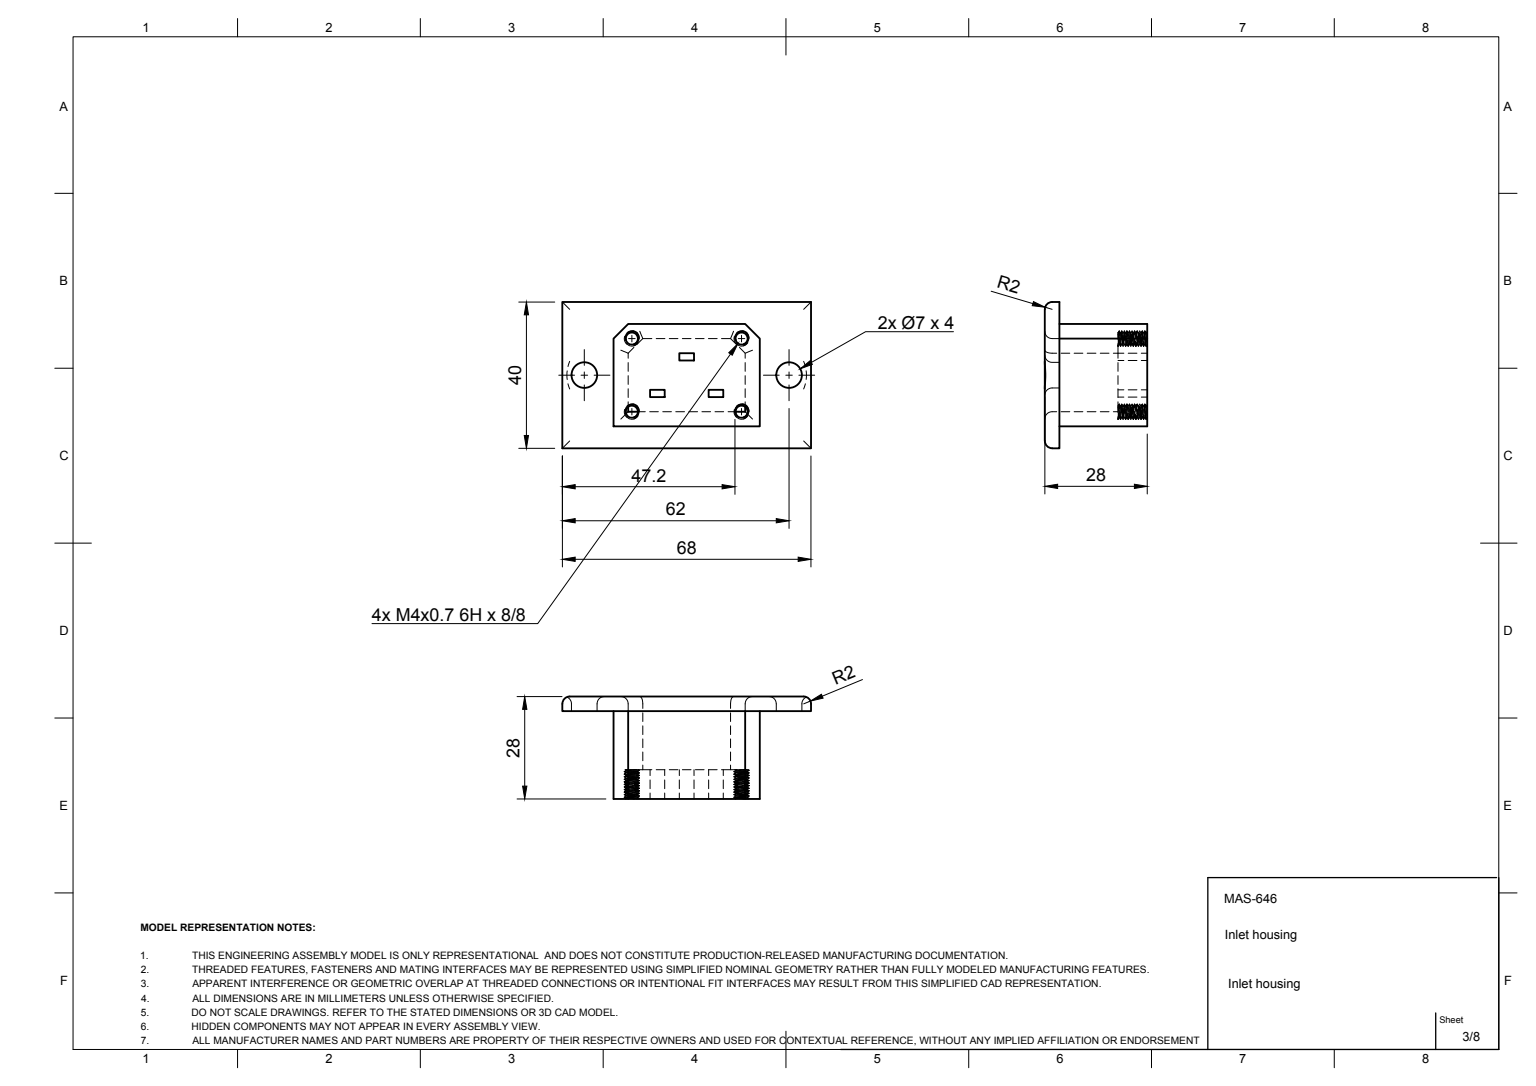
ISO-10303-21;
HEADER;
/* Generated by software containing ST-Developer
 * from STEP Tools, Inc. (www.steptools.com) 
 */

FILE_DESCRIPTION(
/* description */ ('Independent keyed three-contact power inlet for the IEC-connector des
ign category. Longer ground blade, retained contacts, wire termination
 holes and sealed bolted panel interface. Nominal custom interface; IE
C dimensional compatibility and electrical ratings are not assigned.'),

/* implementation_level */ '2;1');

FILE_NAME(
/* name */ 'Inlet housing.step',
/* time_stamp */ '2026-11-08T19:55:04-08:00',
/* author */ (''),
/* organization */ (''),
/* preprocessor_version */ 'ST-DEVELOPER v20.2',
/* originating_system */ 'Autodesk Translation Framework v15.17.0.0',
/* authorisation */ '');

FILE_SCHEMA (('AUTOMOTIVE_DESIGN { 1 0 10303 214 3 1 1 }'));
ENDSEC;

DATA;
#10=MECHANICAL_DESIGN_GEOMETRIC_PRESENTATION_REPRESENTATION('',(#109),#21880);
#89=SHAPE_REPRESENTATION_RELATIONSHIP('SRR','None',#21925,#99);
#99=ADVANCED_BREP_SHAPE_REPRESENTATION('',(#119),#21870);
#109=STYLED_ITEM('',(#21984),#119);
#119=MANIFOLD_SOLID_BREP('Body1',#6381);
#129=B_SPLINE_SURFACE_WITH_KNOTS('',3,3,((#11744,#11745,#11746,#11747,#11748,
#11749,#11750,#11751,#11752,#11753,#11754,#11755,#11756,#11757,#11758,#11759,
#11760,#11761,#11762,#11763,#11764,#11765,#11766,#11767,#11768,#11769,#11770,
#11771,#11772,#11773,#11774,#11775,#11776,#11777,#11778,#11779,#11780,#11781,
#11782,#11783,#11784,#11785,#11786,#11787,#11788,#11789,#11790,#11791,#11792,
#11793,#11794,#11795,#11796,#11797,#11798,#11799,#11800,#11801,#11802,#11803,
#11804,#11805,#11806,#11807,#11808,#11809,#11810,#11811,#11812,#11813,#11814,
#11815,#11816,#11817,#11818,#11819,#11820),(#11821,#11822,#11823,#11824,
#11825,#11826,#11827,#11828,#11829,#11830,#11831,#11832,#11833,#11834,#11835,
#11836,#11837,#11838,#11839,#11840,#11841,#11842,#11843,#11844,#11845,#11846,
#11847,#11848,#11849,#11850,#11851,#11852,#11853,#11854,#11855,#11856,#11857,
#11858,#11859,#11860,#11861,#11862,#11863,#11864,#11865,#11866,#11867,#11868,
#11869,#11870,#11871,#11872,#11873,#11874,#11875,#11876,#11877,#11878,#11879,
#11880,#11881,#11882,#11883,#11884,#11885,#11886,#11887,#11888,#11889,#11890,
#11891,#11892,#11893,#11894,#11895,#11896,#11897),(#11898,#11899,#11900,
#11901,#11902,#11903,#11904,#11905,#11906,#11907,#11908,#11909,#11910,#11911,
#11912,#11913,#11914,#11915,#11916,#11917,#11918,#11919,#11920,#11921,#11922,
#11923,#11924,#11925,#11926,#11927,#11928,#11929,#11930,#11931,#11932,#11933,
#11934,#11935,#11936,#11937,#11938,#11939,#11940,#11941,#11942,#11943,#11944,
#11945,#11946,#11947,#11948,#11949,#11950,#11951,#11952,#11953,#11954,#11955,
#11956,#11957,#11958,#11959,#11960,#11961,#11962,#11963,#11964,#11965,#11966,
#11967,#11968,#11969,#11970,#11971,#11972,#11973,#11974),(#11975,#11976,
#11977,#11978,#11979,#11980,#11981,#11982,#11983,#11984,#11985,#11986,#11987,
#11988,#11989,#11990,#11991,#11992,#11993,#11994,#11995,#11996,#11997,#11998,
#11999,#12000,#12001,#12002,#12003,#12004,#12005,#12006,#12007,#12008,#12009,
#12010,#12011,#12012,#12013,#12014,#12015,#12016,#12017,#12018,#12019,#12020,
#12021,#12022,#12023,#12024,#12025,#12026,#12027,#12028,#12029,#12030,#12031,
#12032,#12033,#12034,#12035,#12036,#12037,#12038,#12039,#12040,#12041,#12042,
#12043,#12044,#12045,#12046,#12047,#12048,#12049,#12050,#12051)),
 .UNSPECIFIED.,.F.,.F.,.F.,(4,4),(4,1,1,1,1,1,1,1,1,1,1,1,1,1,1,1,1,1,1,
1,1,1,1,1,1,1,1,1,1,1,1,1,1,1,1,1,1,1,1,1,1,1,1,1,1,1,1,1,1,1,1,1,1,1,1,
1,1,1,1,1,1,1,1,1,1,1,1,1,1,1,1,1,1,1,4),(0.,0.0448889834294934),(11.8615800042567,
12.859180611653,13.8567812190493,14.8543818264456,15.8519824338419,16.8495830412382,
17.8471836486345,18.8447842560309,19.8423848634272,20.8399854708235,21.8375860782198,
22.8351866856161,23.8327872930124,24.8303879004087,25.827988507805,26.8255891152013,
27.8231897225976,28.8207903299939,29.8183909373903,30.8159915447866,31.8135921521829,
32.8111927595792,33.8087933669755,34.8063939743718,35.8039945817681,36.8015951891644,
37.7991957965607,38.796796403957,39.7943970113533,40.7919976187497,41.789598226146,
42.7871988335423,43.7847994409386,44.7824000483349,45.7800006557312,46.7776012631275,
47.7752018705238,48.7728024779201,49.7704030853164,50.7680036927128,51.7656043001091,
52.7632049075054,53.7608055149017,54.758406122298,55.7560067296943,56.7536073370906,
57.7512079444869,58.7488085518832,59.7464091592795,60.7440097666758,61.7416103740722,
62.7392109814685,63.7368115888648,64.7344121962611,65.7320128036574,66.7296134110537,
67.72721401845,68.7248146258463,69.7224152332426,70.7200158406389,71.7176164480352,
72.7152170554316,73.7128176628279,74.7104182702242,75.7080188776205,76.7056194850168,
77.7032200924131,78.7008206998094,79.6984213072057,80.696021914602,81.6936225219983,
82.6912231293946,83.688823736791,84.6864243441873,85.6840249515836),
 .UNSPECIFIED.);
#130=B_SPLINE_SURFACE_WITH_KNOTS('',3,3,((#12248,#12249,#12250,#12251,#12252,
#12253,#12254,#12255,#12256,#12257,#12258,#12259,#12260,#12261,#12262,#12263,
#12264,#12265,#12266,#12267,#12268,#12269,#12270,#12271,#12272,#12273,#12274,
#12275,#12276,#12277,#12278,#12279,#12280,#12281,#12282,#12283,#12284,#12285,
#12286,#12287,#12288,#12289,#12290,#12291,#12292,#12293,#12294,#12295,#12296,
#12297,#12298,#12299,#12300,#12301,#12302,#12303,#12304,#12305,#12306,#12307,
#12308,#12309,#12310,#12311,#12312,#12313,#12314,#12315,#12316,#12317,#12318,
#12319,#12320,#12321,#12322,#12323,#12324),(#12325,#12326,#12327,#12328,
#12329,#12330,#12331,#12332,#12333,#12334,#12335,#12336,#12337,#12338,#12339,
#12340,#12341,#12342,#12343,#12344,#12345,#12346,#12347,#12348,#12349,#12350,
#12351,#12352,#12353,#12354,#12355,#12356,#12357,#12358,#12359,#12360,#12361,
#12362,#12363,#12364,#12365,#12366,#12367,#12368,#12369,#12370,#12371,#12372,
#12373,#12374,#12375,#12376,#12377,#12378,#12379,#12380,#12381,#12382,#12383,
#12384,#12385,#12386,#12387,#12388,#12389,#12390,#12391,#12392,#12393,#12394,
#12395,#12396,#12397,#12398,#12399,#12400,#12401),(#12402,#12403,#12404,
#12405,#12406,#12407,#12408,#12409,#12410,#12411,#12412,#12413,#12414,#12415,
#12416,#12417,#12418,#12419,#12420,#12421,#12422,#12423,#12424,#12425,#12426,
#12427,#12428,#12429,#12430,#12431,#12432,#12433,#12434,#12435,#12436,#12437,
#12438,#12439,#12440,#12441,#12442,#12443,#12444,#12445,#12446,#12447,#12448,
#12449,#12450,#12451,#12452,#12453,#12454,#12455,#12456,#12457,#12458,#12459,
#12460,#12461,#12462,#12463,#12464,#12465,#12466,#12467,#12468,#12469,#12470,
#12471,#12472,#12473,#12474,#12475,#12476,#12477,#12478),(#12479,#12480,
#12481,#12482,#12483,#12484,#12485,#12486,#12487,#12488,#12489,#12490,#12491,
#12492,#12493,#12494,#12495,#12496,#12497,#12498,#12499,#12500,#12501,#12502,
#12503,#12504,#12505,#12506,#12507,#12508,#12509,#12510,#12511,#12512,#12513,
#12514,#12515,#12516,#12517,#12518,#12519,#12520,#12521,#12522,#12523,#12524,
#12525,#12526,#12527,#12528,#12529,#12530,#12531,#12532,#12533,#12534,#12535,
#12536,#12537,#12538,#12539,#12540,#12541,#12542,#12543,#12544,#12545,#12546,
#12547,#12548,#12549,#12550,#12551,#12552,#12553,#12554,#12555)),
 .UNSPECIFIED.,.F.,.F.,.F.,(4,4),(4,1,1,1,1,1,1,1,1,1,1,1,1,1,1,1,1,1,1,
1,1,1,1,1,1,1,1,1,1,1,1,1,1,1,1,1,1,1,1,1,1,1,1,1,1,1,1,1,1,1,1,1,1,1,1,
1,1,1,1,1,1,1,1,1,1,1,1,1,1,1,1,1,1,1,4),(0.,0.0448889834294934),(14.3981410127769,
15.3957416201732,16.3933422275696,17.3909428349659,18.3885434423622,19.3861440497585,
20.3837446571548,21.3813452645511,22.3789458719474,23.3765464793437,24.37414708674,
25.3717476941363,26.3693483015326,27.366948908929,28.3645495163253,29.3621501237216,
30.3597507311179,31.3573513385142,32.3549519459105,33.3525525533068,34.3501531607031,
35.3477537680994,36.3453543754957,37.342954982892,38.3405555902884,39.3381561976847,
40.335756805081,41.3333574124773,42.3309580198736,43.3285586272699,44.3261592346662,
45.3237598420625,46.3213604494588,47.3189610568551,48.3165616642514,49.3141622716478,
50.3117628790441,51.3093634864404,52.3069640938367,53.304564701233,54.3021653086293,
55.2997659160256,56.2973665234219,57.2949671308182,58.2925677382145,59.2901683456108,
60.2877689530072,61.2853695604035,62.2829701677998,63.2805707751961,64.2781713825924,
65.2757719899887,66.273372597385,67.2709732047813,68.2685738121776,69.2661744195739,
70.2637750269702,71.2613756343666,72.2589762417629,73.2565768491592,74.2541774565555,
75.2517780639518,76.2493786713481,77.2469792787444,78.2445798861407,79.242180493537,
80.2397811009333,81.2373817083296,82.2349823157259,83.2325829231223,84.2301835305186,
85.2277841379149,86.2253847453112,87.2229853527075,88.2205859601038),
 .UNSPECIFIED.);
#131=B_SPLINE_SURFACE_WITH_KNOTS('',3,3,((#13305,#13306,#13307,#13308,#13309,
#13310,#13311,#13312,#13313,#13314,#13315,#13316,#13317,#13318,#13319,#13320,
#13321,#13322,#13323,#13324,#13325,#13326,#13327,#13328,#13329,#13330,#13331,
#13332,#13333,#13334,#13335,#13336,#13337,#13338,#13339,#13340,#13341,#13342,
#13343,#13344,#13345,#13346,#13347,#13348,#13349,#13350,#13351,#13352,#13353,
#13354,#13355,#13356,#13357,#13358,#13359,#13360,#13361,#13362,#13363,#13364,
#13365,#13366,#13367,#13368,#13369,#13370,#13371,#13372,#13373,#13374,#13375,
#13376,#13377,#13378,#13379,#13380,#13381),(#13382,#13383,#13384,#13385,
#13386,#13387,#13388,#13389,#13390,#13391,#13392,#13393,#13394,#13395,#13396,
#13397,#13398,#13399,#13400,#13401,#13402,#13403,#13404,#13405,#13406,#13407,
#13408,#13409,#13410,#13411,#13412,#13413,#13414,#13415,#13416,#13417,#13418,
#13419,#13420,#13421,#13422,#13423,#13424,#13425,#13426,#13427,#13428,#13429,
#13430,#13431,#13432,#13433,#13434,#13435,#13436,#13437,#13438,#13439,#13440,
#13441,#13442,#13443,#13444,#13445,#13446,#13447,#13448,#13449,#13450,#13451,
#13452,#13453,#13454,#13455,#13456,#13457,#13458),(#13459,#13460,#13461,
#13462,#13463,#13464,#13465,#13466,#13467,#13468,#13469,#13470,#13471,#13472,
#13473,#13474,#13475,#13476,#13477,#13478,#13479,#13480,#13481,#13482,#13483,
#13484,#13485,#13486,#13487,#13488,#13489,#13490,#13491,#13492,#13493,#13494,
#13495,#13496,#13497,#13498,#13499,#13500,#13501,#13502,#13503,#13504,#13505,
#13506,#13507,#13508,#13509,#13510,#13511,#13512,#13513,#13514,#13515,#13516,
#13517,#13518,#13519,#13520,#13521,#13522,#13523,#13524,#13525,#13526,#13527,
#13528,#13529,#13530,#13531,#13532,#13533,#13534,#13535),(#13536,#13537,
#13538,#13539,#13540,#13541,#13542,#13543,#13544,#13545,#13546,#13547,#13548,
#13549,#13550,#13551,#13552,#13553,#13554,#13555,#13556,#13557,#13558,#13559,
#13560,#13561,#13562,#13563,#13564,#13565,#13566,#13567,#13568,#13569,#13570,
#13571,#13572,#13573,#13574,#13575,#13576,#13577,#13578,#13579,#13580,#13581,
#13582,#13583,#13584,#13585,#13586,#13587,#13588,#13589,#13590,#13591,#13592,
#13593,#13594,#13595,#13596,#13597,#13598,#13599,#13600,#13601,#13602,#13603,
#13604,#13605,#13606,#13607,#13608,#13609,#13610,#13611,#13612)),
 .UNSPECIFIED.,.F.,.F.,.F.,(4,4),(4,1,1,1,1,1,1,1,1,1,1,1,1,1,1,1,1,1,1,
1,1,1,1,1,1,1,1,1,1,1,1,1,1,1,1,1,1,1,1,1,1,1,1,1,1,1,1,1,1,1,1,1,1,1,1,
1,1,1,1,1,1,1,1,1,1,1,1,1,1,1,1,1,1,1,4),(0.,0.0448889834294934),(11.8615800042567,
12.859180611653,13.8567812190493,14.8543818264456,15.8519824338419,16.8495830412382,
17.8471836486345,18.8447842560308,19.8423848634271,20.8399854708235,21.8375860782198,
22.8351866856161,23.8327872930124,24.8303879004087,25.827988507805,26.8255891152013,
27.8231897225976,28.8207903299939,29.8183909373902,30.8159915447865,31.8135921521829,
32.8111927595792,33.8087933669755,34.8063939743718,35.8039945817681,36.8015951891644,
37.7991957965607,38.796796403957,39.7943970113533,40.7919976187496,41.7895982261459,
42.7871988335423,43.7847994409386,44.7824000483349,45.7800006557312,46.7776012631275,
47.7752018705238,48.7728024779201,49.7704030853164,50.7680036927127,51.765604300109,
52.7632049075054,53.7608055149017,54.758406122298,55.7560067296943,56.7536073370906,
57.7512079444869,58.7488085518832,59.7464091592795,60.7440097666758,61.7416103740721,
62.7392109814684,63.7368115888648,64.7344121962611,65.7320128036574,66.7296134110537,
67.72721401845,68.7248146258463,69.7224152332426,70.7200158406389,71.7176164480352,
72.7152170554315,73.7128176628278,74.7104182702242,75.7080188776205,76.7056194850168,
77.7032200924131,78.7008206998094,79.6984213072057,80.696021914602,81.6936225219983,
82.6912231293946,83.6888237367909,84.6864243441872,85.6840249515836),
 .UNSPECIFIED.);
#132=B_SPLINE_SURFACE_WITH_KNOTS('',3,3,((#13726,#13727,#13728,#13729,#13730,
#13731,#13732,#13733,#13734,#13735,#13736,#13737,#13738,#13739,#13740,#13741,
#13742,#13743,#13744,#13745,#13746,#13747,#13748,#13749,#13750,#13751,#13752,
#13753,#13754,#13755,#13756,#13757,#13758,#13759,#13760,#13761,#13762,#13763,
#13764,#13765,#13766,#13767,#13768,#13769,#13770,#13771,#13772,#13773,#13774,
#13775,#13776,#13777,#13778,#13779,#13780,#13781,#13782,#13783,#13784,#13785,
#13786,#13787,#13788,#13789,#13790,#13791,#13792,#13793,#13794,#13795,#13796,
#13797,#13798,#13799,#13800,#13801,#13802),(#13803,#13804,#13805,#13806,
#13807,#13808,#13809,#13810,#13811,#13812,#13813,#13814,#13815,#13816,#13817,
#13818,#13819,#13820,#13821,#13822,#13823,#13824,#13825,#13826,#13827,#13828,
#13829,#13830,#13831,#13832,#13833,#13834,#13835,#13836,#13837,#13838,#13839,
#13840,#13841,#13842,#13843,#13844,#13845,#13846,#13847,#13848,#13849,#13850,
#13851,#13852,#13853,#13854,#13855,#13856,#13857,#13858,#13859,#13860,#13861,
#13862,#13863,#13864,#13865,#13866,#13867,#13868,#13869,#13870,#13871,#13872,
#13873,#13874,#13875,#13876,#13877,#13878,#13879),(#13880,#13881,#13882,
#13883,#13884,#13885,#13886,#13887,#13888,#13889,#13890,#13891,#13892,#13893,
#13894,#13895,#13896,#13897,#13898,#13899,#13900,#13901,#13902,#13903,#13904,
#13905,#13906,#13907,#13908,#13909,#13910,#13911,#13912,#13913,#13914,#13915,
#13916,#13917,#13918,#13919,#13920,#13921,#13922,#13923,#13924,#13925,#13926,
#13927,#13928,#13929,#13930,#13931,#13932,#13933,#13934,#13935,#13936,#13937,
#13938,#13939,#13940,#13941,#13942,#13943,#13944,#13945,#13946,#13947,#13948,
#13949,#13950,#13951,#13952,#13953,#13954,#13955,#13956),(#13957,#13958,
#13959,#13960,#13961,#13962,#13963,#13964,#13965,#13966,#13967,#13968,#13969,
#13970,#13971,#13972,#13973,#13974,#13975,#13976,#13977,#13978,#13979,#13980,
#13981,#13982,#13983,#13984,#13985,#13986,#13987,#13988,#13989,#13990,#13991,
#13992,#13993,#13994,#13995,#13996,#13997,#13998,#13999,#14000,#14001,#14002,
#14003,#14004,#14005,#14006,#14007,#14008,#14009,#14010,#14011,#14012,#14013,
#14014,#14015,#14016,#14017,#14018,#14019,#14020,#14021,#14022,#14023,#14024,
#14025,#14026,#14027,#14028,#14029,#14030,#14031,#14032,#14033)),
 .UNSPECIFIED.,.F.,.F.,.F.,(4,4),(4,1,1,1,1,1,1,1,1,1,1,1,1,1,1,1,1,1,1,
1,1,1,1,1,1,1,1,1,1,1,1,1,1,1,1,1,1,1,1,1,1,1,1,1,1,1,1,1,1,1,1,1,1,1,1,
1,1,1,1,1,1,1,1,1,1,1,1,1,1,1,1,1,1,1,4),(0.,0.0448889834294934),(14.3981410127769,
15.3957416201732,16.3933422275695,17.3909428349659,18.3885434423622,19.3861440497585,
20.3837446571548,21.3813452645511,22.3789458719474,23.3765464793437,24.37414708674,
25.3717476941363,26.3693483015326,27.3669489089289,28.3645495163252,29.3621501237216,
30.3597507311179,31.3573513385142,32.3549519459105,33.3525525533068,34.3501531607031,
35.3477537680994,36.3453543754957,37.342954982892,38.3405555902883,39.3381561976846,
40.335756805081,41.3333574124773,42.3309580198736,43.3285586272699,44.3261592346662,
45.3237598420625,46.3213604494588,47.3189610568551,48.3165616642514,49.3141622716477,
50.3117628790441,51.3093634864404,52.3069640938367,53.304564701233,54.3021653086293,
55.2997659160256,56.2973665234219,57.2949671308182,58.2925677382145,59.2901683456108,
60.2877689530071,61.2853695604035,62.2829701677998,63.2805707751961,64.2781713825924,
65.2757719899887,66.273372597385,67.2709732047813,68.2685738121776,69.2661744195739,
70.2637750269702,71.2613756343665,72.2589762417629,73.2565768491592,74.2541774565555,
75.2517780639518,76.2493786713481,77.2469792787444,78.2445798861407,79.242180493537,
80.2397811009333,81.2373817083296,82.2349823157259,83.2325829231222,84.2301835305186,
85.2277841379149,86.2253847453112,87.2229853527075,88.2205859601038),
 .UNSPECIFIED.);
#133=B_SPLINE_SURFACE_WITH_KNOTS('',3,3,((#14163,#14164,#14165,#14166,#14167,
#14168,#14169,#14170,#14171,#14172,#14173,#14174,#14175,#14176,#14177,#14178,
#14179,#14180,#14181,#14182,#14183,#14184,#14185,#14186,#14187,#14188,#14189,
#14190,#14191,#14192,#14193,#14194,#14195,#14196,#14197,#14198,#14199,#14200,
#14201,#14202,#14203,#14204,#14205,#14206,#14207,#14208,#14209,#14210,#14211,
#14212,#14213,#14214,#14215,#14216,#14217,#14218,#14219,#14220,#14221,#14222,
#14223,#14224,#14225,#14226,#14227,#14228,#14229,#14230,#14231,#14232,#14233,
#14234,#14235,#14236,#14237,#14238,#14239),(#14240,#14241,#14242,#14243,
#14244,#14245,#14246,#14247,#14248,#14249,#14250,#14251,#14252,#14253,#14254,
#14255,#14256,#14257,#14258,#14259,#14260,#14261,#14262,#14263,#14264,#14265,
#14266,#14267,#14268,#14269,#14270,#14271,#14272,#14273,#14274,#14275,#14276,
#14277,#14278,#14279,#14280,#14281,#14282,#14283,#14284,#14285,#14286,#14287,
#14288,#14289,#14290,#14291,#14292,#14293,#14294,#14295,#14296,#14297,#14298,
#14299,#14300,#14301,#14302,#14303,#14304,#14305,#14306,#14307,#14308,#14309,
#14310,#14311,#14312,#14313,#14314,#14315,#14316),(#14317,#14318,#14319,
#14320,#14321,#14322,#14323,#14324,#14325,#14326,#14327,#14328,#14329,#14330,
#14331,#14332,#14333,#14334,#14335,#14336,#14337,#14338,#14339,#14340,#14341,
#14342,#14343,#14344,#14345,#14346,#14347,#14348,#14349,#14350,#14351,#14352,
#14353,#14354,#14355,#14356,#14357,#14358,#14359,#14360,#14361,#14362,#14363,
#14364,#14365,#14366,#14367,#14368,#14369,#14370,#14371,#14372,#14373,#14374,
#14375,#14376,#14377,#14378,#14379,#14380,#14381,#14382,#14383,#14384,#14385,
#14386,#14387,#14388,#14389,#14390,#14391,#14392,#14393),(#14394,#14395,
#14396,#14397,#14398,#14399,#14400,#14401,#14402,#14403,#14404,#14405,#14406,
#14407,#14408,#14409,#14410,#14411,#14412,#14413,#14414,#14415,#14416,#14417,
#14418,#14419,#14420,#14421,#14422,#14423,#14424,#14425,#14426,#14427,#14428,
#14429,#14430,#14431,#14432,#14433,#14434,#14435,#14436,#14437,#14438,#14439,
#14440,#14441,#14442,#14443,#14444,#14445,#14446,#14447,#14448,#14449,#14450,
#14451,#14452,#14453,#14454,#14455,#14456,#14457,#14458,#14459,#14460,#14461,
#14462,#14463,#14464,#14465,#14466,#14467,#14468,#14469,#14470)),
 .UNSPECIFIED.,.F.,.F.,.F.,(4,4),(4,1,1,1,1,1,1,1,1,1,1,1,1,1,1,1,1,1,1,
1,1,1,1,1,1,1,1,1,1,1,1,1,1,1,1,1,1,1,1,1,1,1,1,1,1,1,1,1,1,1,1,1,1,1,1,
1,1,1,1,1,1,1,1,1,1,1,1,1,1,1,1,1,1,1,4),(0.,0.0448889834294934),(11.8615800042567,
12.859180611653,13.8567812190493,14.8543818264456,15.8519824338419,16.8495830412382,
17.8471836486345,18.8447842560308,19.8423848634271,20.8399854708235,21.8375860782198,
22.8351866856161,23.8327872930124,24.8303879004087,25.827988507805,26.8255891152013,
27.8231897225976,28.8207903299939,29.8183909373902,30.8159915447865,31.8135921521829,
32.8111927595792,33.8087933669755,34.8063939743718,35.8039945817681,36.8015951891644,
37.7991957965607,38.796796403957,39.7943970113533,40.7919976187496,41.7895982261459,
42.7871988335423,43.7847994409386,44.7824000483349,45.7800006557312,46.7776012631275,
47.7752018705238,48.7728024779201,49.7704030853164,50.7680036927127,51.765604300109,
52.7632049075054,53.7608055149017,54.758406122298,55.7560067296943,56.7536073370906,
57.7512079444869,58.7488085518832,59.7464091592795,60.7440097666758,61.7416103740721,
62.7392109814684,63.7368115888648,64.7344121962611,65.7320128036574,66.7296134110537,
67.72721401845,68.7248146258463,69.7224152332426,70.7200158406389,71.7176164480352,
72.7152170554315,73.7128176628278,74.7104182702242,75.7080188776205,76.7056194850168,
77.7032200924131,78.7008206998094,79.6984213072057,80.696021914602,81.6936225219983,
82.6912231293946,83.6888237367909,84.6864243441872,85.6840249515836),
 .UNSPECIFIED.);
#134=B_SPLINE_SURFACE_WITH_KNOTS('',3,3,((#14584,#14585,#14586,#14587,#14588,
#14589,#14590,#14591,#14592,#14593,#14594,#14595,#14596,#14597,#14598,#14599,
#14600,#14601,#14602,#14603,#14604,#14605,#14606,#14607,#14608,#14609,#14610,
#14611,#14612,#14613,#14614,#14615,#14616,#14617,#14618,#14619,#14620,#14621,
#14622,#14623,#14624,#14625,#14626,#14627,#14628,#14629,#14630,#14631,#14632,
#14633,#14634,#14635,#14636,#14637,#14638,#14639,#14640,#14641,#14642,#14643,
#14644,#14645,#14646,#14647,#14648,#14649,#14650,#14651,#14652,#14653,#14654,
#14655,#14656,#14657,#14658,#14659,#14660),(#14661,#14662,#14663,#14664,
#14665,#14666,#14667,#14668,#14669,#14670,#14671,#14672,#14673,#14674,#14675,
#14676,#14677,#14678,#14679,#14680,#14681,#14682,#14683,#14684,#14685,#14686,
#14687,#14688,#14689,#14690,#14691,#14692,#14693,#14694,#14695,#14696,#14697,
#14698,#14699,#14700,#14701,#14702,#14703,#14704,#14705,#14706,#14707,#14708,
#14709,#14710,#14711,#14712,#14713,#14714,#14715,#14716,#14717,#14718,#14719,
#14720,#14721,#14722,#14723,#14724,#14725,#14726,#14727,#14728,#14729,#14730,
#14731,#14732,#14733,#14734,#14735,#14736,#14737),(#14738,#14739,#14740,
#14741,#14742,#14743,#14744,#14745,#14746,#14747,#14748,#14749,#14750,#14751,
#14752,#14753,#14754,#14755,#14756,#14757,#14758,#14759,#14760,#14761,#14762,
#14763,#14764,#14765,#14766,#14767,#14768,#14769,#14770,#14771,#14772,#14773,
#14774,#14775,#14776,#14777,#14778,#14779,#14780,#14781,#14782,#14783,#14784,
#14785,#14786,#14787,#14788,#14789,#14790,#14791,#14792,#14793,#14794,#14795,
#14796,#14797,#14798,#14799,#14800,#14801,#14802,#14803,#14804,#14805,#14806,
#14807,#14808,#14809,#14810,#14811,#14812,#14813,#14814),(#14815,#14816,
#14817,#14818,#14819,#14820,#14821,#14822,#14823,#14824,#14825,#14826,#14827,
#14828,#14829,#14830,#14831,#14832,#14833,#14834,#14835,#14836,#14837,#14838,
#14839,#14840,#14841,#14842,#14843,#14844,#14845,#14846,#14847,#14848,#14849,
#14850,#14851,#14852,#14853,#14854,#14855,#14856,#14857,#14858,#14859,#14860,
#14861,#14862,#14863,#14864,#14865,#14866,#14867,#14868,#14869,#14870,#14871,
#14872,#14873,#14874,#14875,#14876,#14877,#14878,#14879,#14880,#14881,#14882,
#14883,#14884,#14885,#14886,#14887,#14888,#14889,#14890,#14891)),
 .UNSPECIFIED.,.F.,.F.,.F.,(4,4),(4,1,1,1,1,1,1,1,1,1,1,1,1,1,1,1,1,1,1,
1,1,1,1,1,1,1,1,1,1,1,1,1,1,1,1,1,1,1,1,1,1,1,1,1,1,1,1,1,1,1,1,1,1,1,1,
1,1,1,1,1,1,1,1,1,1,1,1,1,1,1,1,1,1,1,4),(0.,0.0448889834294934),(14.3981410127769,
15.3957416201732,16.3933422275695,17.3909428349659,18.3885434423622,19.3861440497585,
20.3837446571548,21.3813452645511,22.3789458719474,23.3765464793437,24.37414708674,
25.3717476941363,26.3693483015326,27.3669489089289,28.3645495163252,29.3621501237216,
30.3597507311179,31.3573513385142,32.3549519459105,33.3525525533068,34.3501531607031,
35.3477537680994,36.3453543754957,37.342954982892,38.3405555902883,39.3381561976846,
40.335756805081,41.3333574124773,42.3309580198736,43.3285586272699,44.3261592346662,
45.3237598420625,46.3213604494588,47.3189610568551,48.3165616642514,49.3141622716477,
50.3117628790441,51.3093634864404,52.3069640938367,53.304564701233,54.3021653086293,
55.2997659160256,56.2973665234219,57.2949671308182,58.2925677382145,59.2901683456108,
60.2877689530071,61.2853695604035,62.2829701677998,63.2805707751961,64.2781713825924,
65.2757719899887,66.273372597385,67.2709732047813,68.2685738121776,69.2661744195739,
70.2637750269702,71.2613756343665,72.2589762417629,73.2565768491592,74.2541774565555,
75.2517780639518,76.2493786713481,77.2469792787444,78.2445798861407,79.242180493537,
80.2397811009333,81.2373817083296,82.2349823157259,83.2325829231222,84.2301835305186,
85.2277841379149,86.2253847453112,87.2229853527075,88.2205859601038),
 .UNSPECIFIED.);
#135=B_SPLINE_SURFACE_WITH_KNOTS('',3,3,((#15021,#15022,#15023,#15024,#15025,
#15026,#15027,#15028,#15029,#15030,#15031,#15032,#15033,#15034,#15035,#15036,
#15037,#15038,#15039,#15040,#15041,#15042,#15043,#15044,#15045,#15046,#15047,
#15048,#15049,#15050,#15051,#15052,#15053,#15054,#15055,#15056,#15057,#15058,
#15059,#15060,#15061,#15062,#15063,#15064,#15065,#15066,#15067,#15068,#15069,
#15070,#15071,#15072,#15073,#15074,#15075,#15076,#15077,#15078,#15079,#15080,
#15081,#15082,#15083,#15084,#15085,#15086,#15087,#15088,#15089,#15090,#15091,
#15092,#15093,#15094,#15095,#15096,#15097),(#15098,#15099,#15100,#15101,
#15102,#15103,#15104,#15105,#15106,#15107,#15108,#15109,#15110,#15111,#15112,
#15113,#15114,#15115,#15116,#15117,#15118,#15119,#15120,#15121,#15122,#15123,
#15124,#15125,#15126,#15127,#15128,#15129,#15130,#15131,#15132,#15133,#15134,
#15135,#15136,#15137,#15138,#15139,#15140,#15141,#15142,#15143,#15144,#15145,
#15146,#15147,#15148,#15149,#15150,#15151,#15152,#15153,#15154,#15155,#15156,
#15157,#15158,#15159,#15160,#15161,#15162,#15163,#15164,#15165,#15166,#15167,
#15168,#15169,#15170,#15171,#15172,#15173,#15174),(#15175,#15176,#15177,
#15178,#15179,#15180,#15181,#15182,#15183,#15184,#15185,#15186,#15187,#15188,
#15189,#15190,#15191,#15192,#15193,#15194,#15195,#15196,#15197,#15198,#15199,
#15200,#15201,#15202,#15203,#15204,#15205,#15206,#15207,#15208,#15209,#15210,
#15211,#15212,#15213,#15214,#15215,#15216,#15217,#15218,#15219,#15220,#15221,
#15222,#15223,#15224,#15225,#15226,#15227,#15228,#15229,#15230,#15231,#15232,
#15233,#15234,#15235,#15236,#15237,#15238,#15239,#15240,#15241,#15242,#15243,
#15244,#15245,#15246,#15247,#15248,#15249,#15250,#15251),(#15252,#15253,
#15254,#15255,#15256,#15257,#15258,#15259,#15260,#15261,#15262,#15263,#15264,
#15265,#15266,#15267,#15268,#15269,#15270,#15271,#15272,#15273,#15274,#15275,
#15276,#15277,#15278,#15279,#15280,#15281,#15282,#15283,#15284,#15285,#15286,
#15287,#15288,#15289,#15290,#15291,#15292,#15293,#15294,#15295,#15296,#15297,
#15298,#15299,#15300,#15301,#15302,#15303,#15304,#15305,#15306,#15307,#15308,
#15309,#15310,#15311,#15312,#15313,#15314,#15315,#15316,#15317,#15318,#15319,
#15320,#15321,#15322,#15323,#15324,#15325,#15326,#15327,#15328)),
 .UNSPECIFIED.,.F.,.F.,.F.,(4,4),(4,1,1,1,1,1,1,1,1,1,1,1,1,1,1,1,1,1,1,
1,1,1,1,1,1,1,1,1,1,1,1,1,1,1,1,1,1,1,1,1,1,1,1,1,1,1,1,1,1,1,1,1,1,1,1,
1,1,1,1,1,1,1,1,1,1,1,1,1,1,1,1,1,1,1,4),(0.,0.0448889834294934),(11.8615800042567,
12.859180611653,13.8567812190493,14.8543818264456,15.8519824338419,16.8495830412382,
17.8471836486345,18.8447842560309,19.8423848634272,20.8399854708235,21.8375860782198,
22.8351866856161,23.8327872930124,24.8303879004087,25.827988507805,26.8255891152013,
27.8231897225976,28.8207903299939,29.8183909373903,30.8159915447866,31.8135921521829,
32.8111927595792,33.8087933669755,34.8063939743718,35.8039945817681,36.8015951891644,
37.7991957965607,38.796796403957,39.7943970113533,40.7919976187497,41.789598226146,
42.7871988335423,43.7847994409386,44.7824000483349,45.7800006557312,46.7776012631275,
47.7752018705238,48.7728024779201,49.7704030853164,50.7680036927127,51.7656043001091,
52.7632049075054,53.7608055149017,54.758406122298,55.7560067296943,56.7536073370906,
57.7512079444869,58.7488085518832,59.7464091592795,60.7440097666758,61.7416103740721,
62.7392109814685,63.7368115888648,64.7344121962611,65.7320128036574,66.7296134110537,
67.72721401845,68.7248146258463,69.7224152332426,70.7200158406389,71.7176164480352,
72.7152170554315,73.7128176628279,74.7104182702242,75.7080188776205,76.7056194850168,
77.7032200924131,78.7008206998094,79.6984213072057,80.696021914602,81.6936225219983,
82.6912231293946,83.688823736791,84.6864243441873,85.6840249515836),
 .UNSPECIFIED.);
#136=B_SPLINE_SURFACE_WITH_KNOTS('',3,3,((#15442,#15443,#15444,#15445,#15446,
#15447,#15448,#15449,#15450,#15451,#15452,#15453,#15454,#15455,#15456,#15457,
#15458,#15459,#15460,#15461,#15462,#15463,#15464,#15465,#15466,#15467,#15468,
#15469,#15470,#15471,#15472,#15473,#15474,#15475,#15476,#15477,#15478,#15479,
#15480,#15481,#15482,#15483,#15484,#15485,#15486,#15487,#15488,#15489,#15490,
#15491,#15492,#15493,#15494,#15495,#15496,#15497,#15498,#15499,#15500,#15501,
#15502,#15503,#15504,#15505,#15506,#15507,#15508,#15509,#15510,#15511,#15512,
#15513,#15514,#15515,#15516,#15517,#15518),(#15519,#15520,#15521,#15522,
#15523,#15524,#15525,#15526,#15527,#15528,#15529,#15530,#15531,#15532,#15533,
#15534,#15535,#15536,#15537,#15538,#15539,#15540,#15541,#15542,#15543,#15544,
#15545,#15546,#15547,#15548,#15549,#15550,#15551,#15552,#15553,#15554,#15555,
#15556,#15557,#15558,#15559,#15560,#15561,#15562,#15563,#15564,#15565,#15566,
#15567,#15568,#15569,#15570,#15571,#15572,#15573,#15574,#15575,#15576,#15577,
#15578,#15579,#15580,#15581,#15582,#15583,#15584,#15585,#15586,#15587,#15588,
#15589,#15590,#15591,#15592,#15593,#15594,#15595),(#15596,#15597,#15598,
#15599,#15600,#15601,#15602,#15603,#15604,#15605,#15606,#15607,#15608,#15609,
#15610,#15611,#15612,#15613,#15614,#15615,#15616,#15617,#15618,#15619,#15620,
#15621,#15622,#15623,#15624,#15625,#15626,#15627,#15628,#15629,#15630,#15631,
#15632,#15633,#15634,#15635,#15636,#15637,#15638,#15639,#15640,#15641,#15642,
#15643,#15644,#15645,#15646,#15647,#15648,#15649,#15650,#15651,#15652,#15653,
#15654,#15655,#15656,#15657,#15658,#15659,#15660,#15661,#15662,#15663,#15664,
#15665,#15666,#15667,#15668,#15669,#15670,#15671,#15672),(#15673,#15674,
#15675,#15676,#15677,#15678,#15679,#15680,#15681,#15682,#15683,#15684,#15685,
#15686,#15687,#15688,#15689,#15690,#15691,#15692,#15693,#15694,#15695,#15696,
#15697,#15698,#15699,#15700,#15701,#15702,#15703,#15704,#15705,#15706,#15707,
#15708,#15709,#15710,#15711,#15712,#15713,#15714,#15715,#15716,#15717,#15718,
#15719,#15720,#15721,#15722,#15723,#15724,#15725,#15726,#15727,#15728,#15729,
#15730,#15731,#15732,#15733,#15734,#15735,#15736,#15737,#15738,#15739,#15740,
#15741,#15742,#15743,#15744,#15745,#15746,#15747,#15748,#15749)),
 .UNSPECIFIED.,.F.,.F.,.F.,(4,4),(4,1,1,1,1,1,1,1,1,1,1,1,1,1,1,1,1,1,1,
1,1,1,1,1,1,1,1,1,1,1,1,1,1,1,1,1,1,1,1,1,1,1,1,1,1,1,1,1,1,1,1,1,1,1,1,
1,1,1,1,1,1,1,1,1,1,1,1,1,1,1,1,1,1,1,4),(0.,0.0448889834294934),(14.3981410127769,
15.3957416201732,16.3933422275696,17.3909428349659,18.3885434423622,19.3861440497585,
20.3837446571548,21.3813452645511,22.3789458719474,23.3765464793437,24.37414708674,
25.3717476941363,26.3693483015326,27.366948908929,28.3645495163253,29.3621501237216,
30.3597507311179,31.3573513385142,32.3549519459105,33.3525525533068,34.3501531607031,
35.3477537680994,36.3453543754957,37.342954982892,38.3405555902884,39.3381561976847,
40.335756805081,41.3333574124773,42.3309580198736,43.3285586272699,44.3261592346662,
45.3237598420625,46.3213604494588,47.3189610568551,48.3165616642514,49.3141622716478,
50.3117628790441,51.3093634864404,52.3069640938367,53.304564701233,54.3021653086293,
55.2997659160256,56.2973665234219,57.2949671308182,58.2925677382145,59.2901683456108,
60.2877689530072,61.2853695604035,62.2829701677998,63.2805707751961,64.2781713825924,
65.2757719899887,66.273372597385,67.2709732047813,68.2685738121776,69.2661744195739,
70.2637750269702,71.2613756343666,72.2589762417629,73.2565768491592,74.2541774565555,
75.2517780639518,76.2493786713481,77.2469792787444,78.2445798861407,79.242180493537,
80.2397811009333,81.2373817083296,82.2349823157259,83.2325829231223,84.2301835305186,
85.2277841379149,86.2253847453112,87.2229853527075,88.2205859601038),
 .UNSPECIFIED.);
#143=TOROIDAL_SURFACE('',#6643,5.5,2.);
#144=TOROIDAL_SURFACE('',#6647,5.5,2.);
#145=FACE_BOUND('',#771,.T.);
#146=FACE_BOUND('',#786,.T.);
#147=FACE_BOUND('',#787,.T.);
#148=FACE_BOUND('',#788,.T.);
#149=FACE_BOUND('',#789,.T.);
#150=FACE_BOUND('',#790,.T.);
#151=FACE_BOUND('',#791,.T.);
#152=FACE_BOUND('',#792,.T.);
#153=FACE_BOUND('',#803,.T.);
#154=FACE_BOUND('',#804,.T.);
#155=FACE_BOUND('',#805,.T.);
#156=FACE_BOUND('',#827,.T.);
#157=FACE_BOUND('',#828,.T.);
#158=FACE_BOUND('',#829,.T.);
#197=PLANE('',#6626);
#198=PLANE('',#6627);
#199=PLANE('',#6628);
#200=PLANE('',#6629);
#201=PLANE('',#6641);
#202=PLANE('',#6642);
#203=PLANE('',#6656);
#204=PLANE('',#6660);
#205=PLANE('',#6661);
#206=PLANE('',#6663);
#207=PLANE('',#6666);
#208=PLANE('',#6668);
#209=PLANE('',#6669);
#210=PLANE('',#6670);
#211=PLANE('',#6671);
#212=PLANE('',#6672);
#213=PLANE('',#6673);
#214=PLANE('',#6674);
#215=PLANE('',#6675);
#216=PLANE('',#6676);
#217=PLANE('',#6677);
#218=PLANE('',#6678);
#219=PLANE('',#6679);
#220=PLANE('',#6680);
#221=PLANE('',#6681);
#222=PLANE('',#6682);
#223=PLANE('',#6683);
#224=PLANE('',#6684);
#225=PLANE('',#6685);
#226=PLANE('',#6686);
#227=PLANE('',#6687);
#228=PLANE('',#6688);
#229=PLANE('',#6689);
#230=PLANE('',#6690);
#231=PLANE('',#6691);
#232=PLANE('',#6692);
#313=ELLIPSE('',#6615,2.16478440058479,2.);
#314=ELLIPSE('',#6616,2.16478440058479,2.);
#315=ELLIPSE('',#6618,2.16478440058479,2.);
#316=ELLIPSE('',#6620,2.16478440058479,2.);
#317=ELLIPSE('',#6622,2.82842712474619,2.);
#318=ELLIPSE('',#6624,2.82842712474619,2.);
#319=ELLIPSE('',#6634,2.82842712474619,2.);
#320=ELLIPSE('',#6635,2.82842712474619,2.);
#321=ELLIPSE('',#6637,2.82842712474619,2.);
#322=ELLIPSE('',#6639,2.82842712474619,2.);
#323=FACE_OUTER_BOUND('',#669,.T.);
#324=FACE_OUTER_BOUND('',#670,.T.);
#325=FACE_OUTER_BOUND('',#671,.T.);
#326=FACE_OUTER_BOUND('',#672,.T.);
#327=FACE_OUTER_BOUND('',#673,.T.);
#328=FACE_OUTER_BOUND('',#674,.T.);
#329=FACE_OUTER_BOUND('',#675,.T.);
#330=FACE_OUTER_BOUND('',#676,.T.);
#331=FACE_OUTER_BOUND('',#677,.T.);
#332=FACE_OUTER_BOUND('',#678,.T.);
#333=FACE_OUTER_BOUND('',#679,.T.);
#334=FACE_OUTER_BOUND('',#680,.T.);
#335=FACE_OUTER_BOUND('',#681,.T.);
#336=FACE_OUTER_BOUND('',#682,.T.);
#337=FACE_OUTER_BOUND('',#683,.T.);
#338=FACE_OUTER_BOUND('',#684,.T.);
#339=FACE_OUTER_BOUND('',#685,.T.);
#340=FACE_OUTER_BOUND('',#686,.T.);
#341=FACE_OUTER_BOUND('',#687,.T.);
#342=FACE_OUTER_BOUND('',#688,.T.);
#343=FACE_OUTER_BOUND('',#689,.T.);
#344=FACE_OUTER_BOUND('',#690,.T.);
#345=FACE_OUTER_BOUND('',#691,.T.);
#346=FACE_OUTER_BOUND('',#692,.T.);
#347=FACE_OUTER_BOUND('',#693,.T.);
#348=FACE_OUTER_BOUND('',#694,.T.);
#349=FACE_OUTER_BOUND('',#695,.T.);
#350=FACE_OUTER_BOUND('',#696,.T.);
#351=FACE_OUTER_BOUND('',#697,.T.);
#352=FACE_OUTER_BOUND('',#698,.T.);
#353=FACE_OUTER_BOUND('',#699,.T.);
#354=FACE_OUTER_BOUND('',#700,.T.);
#355=FACE_OUTER_BOUND('',#701,.T.);
#356=FACE_OUTER_BOUND('',#702,.T.);
#357=FACE_OUTER_BOUND('',#703,.T.);
#358=FACE_OUTER_BOUND('',#704,.T.);
#359=FACE_OUTER_BOUND('',#705,.T.);
#360=FACE_OUTER_BOUND('',#706,.T.);
#361=FACE_OUTER_BOUND('',#707,.T.);
#362=FACE_OUTER_BOUND('',#708,.T.);
#363=FACE_OUTER_BOUND('',#709,.T.);
#364=FACE_OUTER_BOUND('',#710,.T.);
#365=FACE_OUTER_BOUND('',#711,.T.);
#366=FACE_OUTER_BOUND('',#712,.T.);
#367=FACE_OUTER_BOUND('',#713,.T.);
#368=FACE_OUTER_BOUND('',#714,.T.);
#369=FACE_OUTER_BOUND('',#715,.T.);
#370=FACE_OUTER_BOUND('',#716,.T.);
#371=FACE_OUTER_BOUND('',#717,.T.);
#372=FACE_OUTER_BOUND('',#718,.T.);
#373=FACE_OUTER_BOUND('',#719,.T.);
#374=FACE_OUTER_BOUND('',#720,.T.);
#375=FACE_OUTER_BOUND('',#721,.T.);
#376=FACE_OUTER_BOUND('',#722,.T.);
#377=FACE_OUTER_BOUND('',#723,.T.);
#378=FACE_OUTER_BOUND('',#724,.T.);
#379=FACE_OUTER_BOUND('',#725,.T.);
#380=FACE_OUTER_BOUND('',#726,.T.);
#381=FACE_OUTER_BOUND('',#727,.T.);
#382=FACE_OUTER_BOUND('',#728,.T.);
#383=FACE_OUTER_BOUND('',#729,.T.);
#384=FACE_OUTER_BOUND('',#730,.T.);
#385=FACE_OUTER_BOUND('',#731,.T.);
#386=FACE_OUTER_BOUND('',#732,.T.);
#387=FACE_OUTER_BOUND('',#733,.T.);
#388=FACE_OUTER_BOUND('',#734,.T.);
#389=FACE_OUTER_BOUND('',#735,.T.);
#390=FACE_OUTER_BOUND('',#736,.T.);
#391=FACE_OUTER_BOUND('',#737,.T.);
#392=FACE_OUTER_BOUND('',#738,.T.);
#393=FACE_OUTER_BOUND('',#739,.T.);
#394=FACE_OUTER_BOUND('',#740,.T.);
#395=FACE_OUTER_BOUND('',#741,.T.);
#396=FACE_OUTER_BOUND('',#742,.T.);
#397=FACE_OUTER_BOUND('',#743,.T.);
#398=FACE_OUTER_BOUND('',#744,.T.);
#399=FACE_OUTER_BOUND('',#745,.T.);
#400=FACE_OUTER_BOUND('',#746,.T.);
#401=FACE_OUTER_BOUND('',#747,.T.);
#402=FACE_OUTER_BOUND('',#748,.T.);
#403=FACE_OUTER_BOUND('',#749,.T.);
#404=FACE_OUTER_BOUND('',#750,.T.);
#405=FACE_OUTER_BOUND('',#751,.T.);
#406=FACE_OUTER_BOUND('',#752,.T.);
#407=FACE_OUTER_BOUND('',#753,.T.);
#408=FACE_OUTER_BOUND('',#754,.T.);
#409=FACE_OUTER_BOUND('',#755,.T.);
#410=FACE_OUTER_BOUND('',#756,.T.);
#411=FACE_OUTER_BOUND('',#757,.T.);
#412=FACE_OUTER_BOUND('',#758,.T.);
#413=FACE_OUTER_BOUND('',#759,.T.);
#414=FACE_OUTER_BOUND('',#760,.T.);
#415=FACE_OUTER_BOUND('',#761,.T.);
#416=FACE_OUTER_BOUND('',#762,.T.);
#417=FACE_OUTER_BOUND('',#763,.T.);
#418=FACE_OUTER_BOUND('',#764,.T.);
#419=FACE_OUTER_BOUND('',#765,.T.);
#420=FACE_OUTER_BOUND('',#766,.T.);
#421=FACE_OUTER_BOUND('',#767,.T.);
#422=FACE_OUTER_BOUND('',#768,.T.);
#423=FACE_OUTER_BOUND('',#769,.T.);
#424=FACE_OUTER_BOUND('',#770,.T.);
#425=FACE_OUTER_BOUND('',#772,.T.);
#426=FACE_OUTER_BOUND('',#773,.T.);
#427=FACE_OUTER_BOUND('',#774,.T.);
#428=FACE_OUTER_BOUND('',#775,.T.);
#429=FACE_OUTER_BOUND('',#776,.T.);
#430=FACE_OUTER_BOUND('',#777,.T.);
#431=FACE_OUTER_BOUND('',#778,.T.);
#432=FACE_OUTER_BOUND('',#779,.T.);
#433=FACE_OUTER_BOUND('',#780,.T.);
#434=FACE_OUTER_BOUND('',#781,.T.);
#435=FACE_OUTER_BOUND('',#782,.T.);
#436=FACE_OUTER_BOUND('',#783,.T.);
#437=FACE_OUTER_BOUND('',#784,.T.);
#438=FACE_OUTER_BOUND('',#785,.T.);
#439=FACE_OUTER_BOUND('',#793,.T.);
#440=FACE_OUTER_BOUND('',#794,.T.);
#441=FACE_OUTER_BOUND('',#795,.T.);
#442=FACE_OUTER_BOUND('',#796,.T.);
#443=FACE_OUTER_BOUND('',#797,.T.);
#444=FACE_OUTER_BOUND('',#798,.T.);
#445=FACE_OUTER_BOUND('',#799,.T.);
#446=FACE_OUTER_BOUND('',#800,.T.);
#447=FACE_OUTER_BOUND('',#801,.T.);
#448=FACE_OUTER_BOUND('',#802,.T.);
#449=FACE_OUTER_BOUND('',#806,.T.);
#450=FACE_OUTER_BOUND('',#807,.T.);
#451=FACE_OUTER_BOUND('',#808,.T.);
#452=FACE_OUTER_BOUND('',#809,.T.);
#453=FACE_OUTER_BOUND('',#810,.T.);
#454=FACE_OUTER_BOUND('',#811,.T.);
#455=FACE_OUTER_BOUND('',#812,.T.);
#456=FACE_OUTER_BOUND('',#813,.T.);
#457=FACE_OUTER_BOUND('',#814,.T.);
#458=FACE_OUTER_BOUND('',#815,.T.);
#459=FACE_OUTER_BOUND('',#816,.T.);
#460=FACE_OUTER_BOUND('',#817,.T.);
#461=FACE_OUTER_BOUND('',#818,.T.);
#462=FACE_OUTER_BOUND('',#819,.T.);
#463=FACE_OUTER_BOUND('',#820,.T.);
#464=FACE_OUTER_BOUND('',#821,.T.);
#465=FACE_OUTER_BOUND('',#822,.T.);
#466=FACE_OUTER_BOUND('',#823,.T.);
#467=FACE_OUTER_BOUND('',#824,.T.);
#468=FACE_OUTER_BOUND('',#825,.T.);
#469=FACE_OUTER_BOUND('',#826,.T.);
#470=FACE_OUTER_BOUND('',#830,.T.);
#471=FACE_OUTER_BOUND('',#831,.T.);
#472=FACE_OUTER_BOUND('',#832,.T.);
#473=FACE_OUTER_BOUND('',#833,.T.);
#474=FACE_OUTER_BOUND('',#834,.T.);
#475=FACE_OUTER_BOUND('',#835,.T.);
#476=FACE_OUTER_BOUND('',#836,.T.);
#477=FACE_OUTER_BOUND('',#837,.T.);
#478=FACE_OUTER_BOUND('',#838,.T.);
#479=FACE_OUTER_BOUND('',#839,.T.);
#480=FACE_OUTER_BOUND('',#840,.T.);
#669=EDGE_LOOP('',(#3975,#3976,#3977,#3978));
#670=EDGE_LOOP('',(#3979,#3980,#3981,#3982));
#671=EDGE_LOOP('',(#3983,#3984,#3985,#3986));
#672=EDGE_LOOP('',(#3987,#3988,#3989,#3990));
#673=EDGE_LOOP('',(#3991,#3992,#3993,#3994));
#674=EDGE_LOOP('',(#3995,#3996,#3997,#3998));
#675=EDGE_LOOP('',(#3999,#4000,#4001,#4002));
#676=EDGE_LOOP('',(#4003,#4004,#4005,#4006));
#677=EDGE_LOOP('',(#4007,#4008,#4009,#4010));
#678=EDGE_LOOP('',(#4011,#4012,#4013,#4014));
#679=EDGE_LOOP('',(#4015,#4016,#4017,#4018));
#680=EDGE_LOOP('',(#4019,#4020,#4021,#4022));
#681=EDGE_LOOP('',(#4023,#4024,#4025,#4026));
#682=EDGE_LOOP('',(#4027,#4028,#4029,#4030));
#683=EDGE_LOOP('',(#4031,#4032,#4033,#4034));
#684=EDGE_LOOP('',(#4035,#4036,#4037,#4038));
#685=EDGE_LOOP('',(#4039,#4040,#4041,#4042));
#686=EDGE_LOOP('',(#4043,#4044,#4045,#4046));
#687=EDGE_LOOP('',(#4047,#4048,#4049,#4050));
#688=EDGE_LOOP('',(#4051,#4052,#4053,#4054));
#689=EDGE_LOOP('',(#4055,#4056,#4057,#4058));
#690=EDGE_LOOP('',(#4059,#4060,#4061,#4062));
#691=EDGE_LOOP('',(#4063,#4064,#4065,#4066));
#692=EDGE_LOOP('',(#4067,#4068,#4069,#4070));
#693=EDGE_LOOP('',(#4071,#4072,#4073,#4074));
#694=EDGE_LOOP('',(#4075,#4076,#4077,#4078));
#695=EDGE_LOOP('',(#4079,#4080,#4081,#4082));
#696=EDGE_LOOP('',(#4083,#4084,#4085,#4086));
#697=EDGE_LOOP('',(#4087,#4088,#4089,#4090));
#698=EDGE_LOOP('',(#4091,#4092,#4093,#4094));
#699=EDGE_LOOP('',(#4095,#4096,#4097,#4098));
#700=EDGE_LOOP('',(#4099,#4100,#4101,#4102));
#701=EDGE_LOOP('',(#4103,#4104,#4105,#4106,#4107));
#702=EDGE_LOOP('',(#4108,#4109,#4110,#4111));
#703=EDGE_LOOP('',(#4112,#4113,#4114,#4115));
#704=EDGE_LOOP('',(#4116,#4117,#4118,#4119));
#705=EDGE_LOOP('',(#4120,#4121,#4122,#4123));
#706=EDGE_LOOP('',(#4124,#4125,#4126,#4127));
#707=EDGE_LOOP('',(#4128,#4129,#4130,#4131));
#708=EDGE_LOOP('',(#4132,#4133,#4134,#4135));
#709=EDGE_LOOP('',(#4136,#4137,#4138,#4139));
#710=EDGE_LOOP('',(#4140,#4141,#4142,#4143));
#711=EDGE_LOOP('',(#4144,#4145,#4146,#4147));
#712=EDGE_LOOP('',(#4148,#4149,#4150,#4151,#4152));
#713=EDGE_LOOP('',(#4153,#4154,#4155,#4156));
#714=EDGE_LOOP('',(#4157,#4158,#4159,#4160));
#715=EDGE_LOOP('',(#4161,#4162,#4163,#4164));
#716=EDGE_LOOP('',(#4165,#4166,#4167,#4168));
#717=EDGE_LOOP('',(#4169,#4170,#4171,#4172));
#718=EDGE_LOOP('',(#4173,#4174,#4175,#4176));
#719=EDGE_LOOP('',(#4177,#4178,#4179,#4180));
#720=EDGE_LOOP('',(#4181,#4182,#4183,#4184));
#721=EDGE_LOOP('',(#4185,#4186,#4187,#4188));
#722=EDGE_LOOP('',(#4189,#4190,#4191,#4192));
#723=EDGE_LOOP('',(#4193,#4194,#4195,#4196));
#724=EDGE_LOOP('',(#4197,#4198,#4199,#4200));
#725=EDGE_LOOP('',(#4201,#4202,#4203,#4204));
#726=EDGE_LOOP('',(#4205,#4206,#4207,#4208));
#727=EDGE_LOOP('',(#4209,#4210,#4211,#4212));
#728=EDGE_LOOP('',(#4213,#4214,#4215,#4216));
#729=EDGE_LOOP('',(#4217,#4218,#4219,#4220));
#730=EDGE_LOOP('',(#4221,#4222,#4223,#4224));
#731=EDGE_LOOP('',(#4225,#4226,#4227,#4228));
#732=EDGE_LOOP('',(#4229,#4230,#4231,#4232));
#733=EDGE_LOOP('',(#4233,#4234,#4235,#4236));
#734=EDGE_LOOP('',(#4237,#4238,#4239,#4240));
#735=EDGE_LOOP('',(#4241,#4242,#4243,#4244));
#736=EDGE_LOOP('',(#4245,#4246,#4247,#4248));
#737=EDGE_LOOP('',(#4249,#4250,#4251,#4252));
#738=EDGE_LOOP('',(#4253,#4254,#4255,#4256));
#739=EDGE_LOOP('',(#4257,#4258,#4259,#4260));
#740=EDGE_LOOP('',(#4261,#4262,#4263,#4264));
#741=EDGE_LOOP('',(#4265,#4266,#4267,#4268));
#742=EDGE_LOOP('',(#4269,#4270,#4271,#4272));
#743=EDGE_LOOP('',(#4273,#4274,#4275,#4276));
#744=EDGE_LOOP('',(#4277,#4278,#4279,#4280));
#745=EDGE_LOOP('',(#4281,#4282,#4283,#4284));
#746=EDGE_LOOP('',(#4285,#4286,#4287,#4288));
#747=EDGE_LOOP('',(#4289,#4290,#4291,#4292));
#748=EDGE_LOOP('',(#4293,#4294,#4295,#4296));
#749=EDGE_LOOP('',(#4297,#4298,#4299,#4300));
#750=EDGE_LOOP('',(#4301,#4302,#4303,#4304));
#751=EDGE_LOOP('',(#4305,#4306,#4307,#4308));
#752=EDGE_LOOP('',(#4309,#4310,#4311,#4312));
#753=EDGE_LOOP('',(#4313,#4314,#4315,#4316));
#754=EDGE_LOOP('',(#4317,#4318,#4319,#4320));
#755=EDGE_LOOP('',(#4321,#4322,#4323,#4324));
#756=EDGE_LOOP('',(#4325,#4326,#4327,#4328));
#757=EDGE_LOOP('',(#4329,#4330,#4331,#4332));
#758=EDGE_LOOP('',(#4333,#4334,#4335,#4336));
#759=EDGE_LOOP('',(#4337,#4338,#4339,#4340));
#760=EDGE_LOOP('',(#4341,#4342,#4343,#4344));
#761=EDGE_LOOP('',(#4345,#4346,#4347,#4348));
#762=EDGE_LOOP('',(#4349,#4350,#4351,#4352));
#763=EDGE_LOOP('',(#4353,#4354,#4355,#4356));
#764=EDGE_LOOP('',(#4357,#4358,#4359,#4360));
#765=EDGE_LOOP('',(#4361,#4362,#4363,#4364));
#766=EDGE_LOOP('',(#4365,#4366,#4367,#4368));
#767=EDGE_LOOP('',(#4369,#4370,#4371,#4372,#4373,#4374));
#768=EDGE_LOOP('',(#4375,#4376,#4377,#4378,#4379));
#769=EDGE_LOOP('',(#4380,#4381,#4382,#4383));
#770=EDGE_LOOP('',(#4384,#4385,#4386,#4387,#4388,#4389,#4390,#4391,#4392));
#771=EDGE_LOOP('',(#4393,#4394,#4395,#4396,#4397,#4398));
#772=EDGE_LOOP('',(#4399,#4400,#4401,#4402,#4403,#4404,#4405));
#773=EDGE_LOOP('',(#4406,#4407,#4408,#4409));
#774=EDGE_LOOP('',(#4410,#4411,#4412,#4413,#4414,#4415));
#775=EDGE_LOOP('',(#4416,#4417,#4418,#4419));
#776=EDGE_LOOP('',(#4420,#4421,#4422,#4423));
#777=EDGE_LOOP('',(#4424,#4425,#4426,#4427));
#778=EDGE_LOOP('',(#4428,#4429,#4430,#4431,#4432,#4433,#4434));
#779=EDGE_LOOP('',(#4435,#4436,#4437,#4438,#4439,#4440,#4441));
#780=EDGE_LOOP('',(#4442,#4443,#4444,#4445,#4446));
#781=EDGE_LOOP('',(#4447,#4448,#4449,#4450,#4451));
#782=EDGE_LOOP('',(#4452,#4453,#4454,#4455));
#783=EDGE_LOOP('',(#4456,#4457,#4458,#4459,#4460,#4461,#4462,#4463,#4464,
#4465,#4466,#4467,#4468,#4469,#4470,#4471,#4472,#4473,#4474,#4475,#4476,
#4477,#4478,#4479,#4480,#4481,#4482,#4483));
#784=EDGE_LOOP('',(#4484,#4485,#4486,#4487,#4488,#4489,#4490,#4491,#4492,
#4493,#4494,#4495,#4496,#4497,#4498,#4499,#4500,#4501,#4502,#4503,#4504,
#4505,#4506,#4507,#4508,#4509,#4510));
#785=EDGE_LOOP('',(#4511,#4512,#4513,#4514,#4515,#4516));
#786=EDGE_LOOP('',(#4517,#4518,#4519,#4520));
#787=EDGE_LOOP('',(#4521,#4522,#4523,#4524));
#788=EDGE_LOOP('',(#4525,#4526,#4527,#4528));
#789=EDGE_LOOP('',(#4529,#4530,#4531,#4532));
#790=EDGE_LOOP('',(#4533,#4534,#4535,#4536));
#791=EDGE_LOOP('',(#4537,#4538,#4539,#4540));
#792=EDGE_LOOP('',(#4541,#4542,#4543,#4544));
#793=EDGE_LOOP('',(#4545,#4546,#4547,#4548));
#794=EDGE_LOOP('',(#4549,#4550,#4551,#4552,#4553,#4554,#4555,#4556,#4557,
#4558,#4559,#4560,#4561,#4562,#4563,#4564,#4565,#4566,#4567,#4568,#4569,
#4570,#4571,#4572,#4573,#4574,#4575));
#795=EDGE_LOOP('',(#4576,#4577,#4578,#4579,#4580,#4581,#4582,#4583,#4584,
#4585,#4586,#4587,#4588,#4589,#4590,#4591,#4592,#4593,#4594,#4595,#4596,
#4597,#4598,#4599,#4600,#4601,#4602));
#796=EDGE_LOOP('',(#4603,#4604,#4605,#4606));
#797=EDGE_LOOP('',(#4607,#4608,#4609,#4610,#4611,#4612,#4613,#4614,#4615,
#4616,#4617,#4618,#4619,#4620,#4621,#4622,#4623,#4624,#4625,#4626,#4627,
#4628,#4629,#4630,#4631,#4632,#4633));
#798=EDGE_LOOP('',(#4634,#4635,#4636,#4637,#4638,#4639,#4640,#4641,#4642,
#4643,#4644,#4645,#4646,#4647,#4648,#4649,#4650,#4651,#4652,#4653,#4654,
#4655,#4656,#4657,#4658,#4659,#4660));
#799=EDGE_LOOP('',(#4661,#4662,#4663,#4664));
#800=EDGE_LOOP('',(#4665,#4666,#4667,#4668,#4669,#4670,#4671,#4672,#4673,
#4674,#4675,#4676,#4677,#4678,#4679,#4680,#4681,#4682,#4683,#4684,#4685,
#4686,#4687,#4688,#4689,#4690,#4691));
#801=EDGE_LOOP('',(#4692,#4693,#4694,#4695,#4696,#4697,#4698,#4699,#4700,
#4701,#4702,#4703,#4704,#4705,#4706,#4707,#4708,#4709,#4710,#4711,#4712,
#4713,#4714,#4715,#4716,#4717,#4718,#4719));
#802=EDGE_LOOP('',(#4720,#4721,#4722,#4723,#4724,#4725,#4726,#4727,#4728,
#4729));
#803=EDGE_LOOP('',(#4730,#4731,#4732,#4733));
#804=EDGE_LOOP('',(#4734,#4735,#4736,#4737));
#805=EDGE_LOOP('',(#4738,#4739,#4740,#4741));
#806=EDGE_LOOP('',(#4742,#4743,#4744,#4745,#4746,#4747));
#807=EDGE_LOOP('',(#4748,#4749,#4750,#4751));
#808=EDGE_LOOP('',(#4752,#4753,#4754,#4755,#4756,#4757));
#809=EDGE_LOOP('',(#4758,#4759,#4760,#4761));
#810=EDGE_LOOP('',(#4762,#4763,#4764,#4765));
#811=EDGE_LOOP('',(#4766,#4767,#4768,#4769));
#812=EDGE_LOOP('',(#4770,#4771,#4772,#4773));
#813=EDGE_LOOP('',(#4774,#4775,#4776,#4777));
#814=EDGE_LOOP('',(#4778,#4779,#4780,#4781));
#815=EDGE_LOOP('',(#4782,#4783,#4784,#4785));
#816=EDGE_LOOP('',(#4786,#4787,#4788,#4789));
#817=EDGE_LOOP('',(#4790,#4791,#4792,#4793));
#818=EDGE_LOOP('',(#4794,#4795,#4796,#4797));
#819=EDGE_LOOP('',(#4798,#4799,#4800,#4801));
#820=EDGE_LOOP('',(#4802,#4803,#4804,#4805));
#821=EDGE_LOOP('',(#4806,#4807,#4808,#4809));
#822=EDGE_LOOP('',(#4810,#4811,#4812,#4813));
#823=EDGE_LOOP('',(#4814,#4815,#4816,#4817));
#824=EDGE_LOOP('',(#4818,#4819,#4820,#4821));
#825=EDGE_LOOP('',(#4822,#4823,#4824,#4825));
#826=EDGE_LOOP('',(#4826,#4827,#4828,#4829));
#827=EDGE_LOOP('',(#4830));
#828=EDGE_LOOP('',(#4831));
#829=EDGE_LOOP('',(#4832,#4833,#4834,#4835,#4836,#4837));
#830=EDGE_LOOP('',(#4838,#4839,#4840,#4841));
#831=EDGE_LOOP('',(#4842,#4843,#4844,#4845));
#832=EDGE_LOOP('',(#4846,#4847,#4848,#4849));
#833=EDGE_LOOP('',(#4850,#4851,#4852,#4853));
#834=EDGE_LOOP('',(#4854,#4855,#4856,#4857));
#835=EDGE_LOOP('',(#4858,#4859,#4860,#4861));
#836=EDGE_LOOP('',(#4862,#4863,#4864,#4865));
#837=EDGE_LOOP('',(#4866,#4867,#4868,#4869,#4870));
#838=EDGE_LOOP('',(#4871,#4872,#4873,#4874));
#839=EDGE_LOOP('',(#4875,#4876,#4877,#4878));
#840=EDGE_LOOP('',(#4879,#4880,#4881,#4882));
#1067=CIRCLE('',#6505,1.666);
#1068=CIRCLE('',#6516,1.666);
#1069=CIRCLE('',#6518,1.666);
#1070=CIRCLE('',#6529,1.666);
#1071=CIRCLE('',#6531,1.666);
#1072=CIRCLE('',#6542,1.666);
#1073=CIRCLE('',#6543,1.666);
#1074=CIRCLE('',#6545,1.666);
#1075=CIRCLE('',#6556,1.666);
#1076=CIRCLE('',#6557,1.666);
#1077=CIRCLE('',#6559,2.05475);
#1078=CIRCLE('',#6571,2.05475);
#1079=CIRCLE('',#6573,2.05475);
#1080=CIRCLE('',#6585,2.05475);
#1081=CIRCLE('',#6587,2.05475);
#1082=CIRCLE('',#6599,2.05475);
#1083=CIRCLE('',#6601,2.05475);
#1084=CIRCLE('',#6613,2.05475);
#1085=CIRCLE('',#6630,5.5);
#1086=CIRCLE('',#6631,5.5);
#1087=CIRCLE('',#6632,5.5);
#1088=CIRCLE('',#6644,2.);
#1089=CIRCLE('',#6645,3.5);
#1090=CIRCLE('',#6646,3.5);
#1091=CIRCLE('',#6648,2.);
#1092=CIRCLE('',#6649,3.5);
#1093=CIRCLE('',#6650,3.5);
#1094=CIRCLE('',#6652,3.5);
#1095=CIRCLE('',#6654,3.5);
#1162=B_SPLINE_CURVE_WITH_KNOTS('',3,(#8360,#8361,#8362,#8363,#8364,#8365,
#8366,#8367,#8368,#8369,#8370,#8371,#8372),.UNSPECIFIED.,.F.,.F.,(4,3,3,
3,4),(70.4248606341474,70.8296431251379,71.8272437325342,72.8248443399306,
73.8224449473268),.UNSPECIFIED.);
#1163=B_SPLINE_CURVE_WITH_KNOTS('',3,(#8375,#8376,#8377,#8378,#8379,#8380,
#8381,#8382,#8383,#8384,#8385,#8386,#8387,#8388,#8389,#8390,#8391,#8392,
#8393),.UNSPECIFIED.,.F.,.F.,(4,3,3,3,3,3,4),(-71.8078320820524,-70.829643125138,
-69.8320425177416,-68.8344419103453,-67.836841302949,-66.8392406955527,
-66.6782363354882),.UNSPECIFIED.);
#1164=B_SPLINE_CURVE_WITH_KNOTS('',3,(#8398,#8399,#8400,#8401,#8402,#8403,
#8404,#8405,#8406,#8407,#8408,#8409,#8410,#8411,#8412,#8413,#8414,#8415,
#8416,#8417,#8418,#8419),.UNSPECIFIED.,.F.,.F.,(4,3,3,3,3,3,3,4),(64.1416753269678,
64.8440394807601,65.8416400881564,66.8392406955527,67.836841302949,68.8344419103453,
69.8320425177416,70.4248606341474),.UNSPECIFIED.);
#1165=B_SPLINE_CURVE_WITH_KNOTS('',3,(#8420,#8421,#8422,#8423,#8424,#8425,
#8426,#8427,#8428,#8429,#8430,#8431,#8432,#8433,#8434,#8435,#8436,#8437,
#8438,#8439,#8440,#8441),.UNSPECIFIED.,.F.,.F.,(4,3,3,3,3,3,3,4),(-66.6782363354882,
-65.8416400881564,-64.8440394807601,-63.8464388733638,-62.8488382659675,
-61.8512376585712,-60.8536370511749,-60.3950510283086),.UNSPECIFIED.);
#1166=B_SPLINE_CURVE_WITH_KNOTS('',3,(#8446,#8447,#8448,#8449,#8450,#8451,
#8452,#8453,#8454,#8455,#8456,#8457,#8458,#8459,#8460,#8461,#8462,#8463,
#8464,#8465,#8466,#8467),.UNSPECIFIED.,.F.,.F.,(4,3,3,3,3,3,3,4),(57.8584900197882,
58.8584358363822,59.8560364437785,60.8536370511749,61.8512376585712,62.8488382659675,
63.8464388733638,64.1416753269678),.UNSPECIFIED.);
#1167=B_SPLINE_CURVE_WITH_KNOTS('',3,(#8468,#8469,#8470,#8471,#8472,#8473,
#8474,#8475,#8476,#8477,#8478,#8479,#8480,#8481,#8482,#8483,#8484,#8485,
#8486,#8487,#8488,#8489),.UNSPECIFIED.,.F.,.F.,(4,3,3,3,3,3,3,4),(-60.3950510283086,
-59.8560364437785,-58.8584358363822,-57.8608352289859,-56.8632346215896,
-55.8656340141933,-54.868033406797,-54.111865721129),.UNSPECIFIED.);
#1168=B_SPLINE_CURVE_WITH_KNOTS('',3,(#8494,#8495,#8496,#8497,#8498,#8499,
#8500,#8501,#8502,#8503,#8504,#8505,#8506,#8507,#8508,#8509,#8510,#8511,
#8512,#8513,#8514,#8515),.UNSPECIFIED.,.F.,.F.,(4,3,3,3,3,3,3,4),(51.5753047126087,
51.8752315846081,52.8728321920044,53.8704327994007,54.868033406797,55.8656340141933,
56.8632346215896,57.8584900197882),.UNSPECIFIED.);
#1169=B_SPLINE_CURVE_WITH_KNOTS('',3,(#8516,#8517,#8518,#8519,#8520,#8521,
#8522,#8523,#8524,#8525,#8526,#8527,#8528,#8529,#8530,#8531,#8532,#8533,
#8534,#8535,#8536,#8537,#8538,#8539,#8540),.UNSPECIFIED.,.F.,.F.,(4,3,3,
3,3,3,3,3,4),(-54.111865721129,-53.8704327994007,-52.8728321920044,-51.8752315846081,
-50.8776309772118,-49.8800303698155,-48.8824297624191,-47.8848291550228,
-47.8286804139494),.UNSPECIFIED.);
#1170=B_SPLINE_CURVE_WITH_KNOTS('',3,(#8545,#8546,#8547,#8548,#8549,#8550,
#8551,#8552,#8553,#8554,#8555,#8556,#8557,#8558,#8559,#8560,#8561,#8562,
#8563,#8564,#8565,#8566),.UNSPECIFIED.,.F.,.F.,(4,3,3,3,3,3,3,4),(45.2921194054291,
45.8896279402302,46.8872285476265,47.8848291550228,48.8824297624192,49.8800303698155,
50.8776309772118,51.5753047126087),.UNSPECIFIED.);
#1171=B_SPLINE_CURVE_WITH_KNOTS('',3,(#8567,#8568,#8569,#8570,#8571,#8572,
#8573,#8574,#8575,#8576,#8577,#8578,#8579,#8580,#8581,#8582,#8583,#8584,
#8585,#8586,#8587,#8588),.UNSPECIFIED.,.F.,.F.,(4,3,3,3,3,3,3,4),(-47.8286804139494,
-46.8872285476265,-45.8896279402302,-44.8920273328339,-43.8944267254376,
-42.8968261180413,-41.899225510645,-41.5454951067698),.UNSPECIFIED.);
#1172=B_SPLINE_CURVE_WITH_KNOTS('',3,(#8593,#8594,#8595,#8596,#8597,#8598,
#8599,#8600,#8601,#8602,#8603,#8604,#8605,#8606,#8607,#8608,#8609,#8610,
#8611,#8612,#8613,#8614),.UNSPECIFIED.,.F.,.F.,(4,3,3,3,3,3,3,4),(39.0089340982495,
39.9040242958524,40.9016249032487,41.899225510645,42.8968261180413,43.8944267254376,
44.8920273328339,45.2921194054291),.UNSPECIFIED.);
#1173=B_SPLINE_CURVE_WITH_KNOTS('',3,(#8615,#8616,#8617,#8618,#8619,#8620,
#8621,#8622,#8623,#8624,#8625,#8626,#8627,#8628,#8629,#8630,#8631,#8632,
#8633,#8634,#8635,#8636),.UNSPECIFIED.,.F.,.F.,(4,3,3,3,3,3,3,4),(-41.5454951067698,
-40.9016249032487,-39.9040242958524,-38.9064236884561,-37.9088230810597,
-36.9112224736634,-35.9136218662671,-35.2623097995902),.UNSPECIFIED.);
#1174=B_SPLINE_CURVE_WITH_KNOTS('',3,(#8641,#8642,#8643,#8644,#8645,#8646,
#8647,#8648,#8649,#8650,#8651,#8652,#8653,#8654,#8655,#8656,#8657,#8658,
#8659,#8660,#8661,#8662,#8663,#8664,#8665),.UNSPECIFIED.,.F.,.F.,(4,3,3,
3,3,3,3,3,4),(32.7257487910699,32.9208200440782,33.9184206514745,34.9160212588708,
35.9136218662671,36.9112224736634,37.9088230810598,38.9064236884561,39.0089340982495),
 .UNSPECIFIED.);
#1175=B_SPLINE_CURVE_WITH_KNOTS('',3,(#8666,#8667,#8668,#8669,#8670,#8671,
#8672,#8673,#8674,#8675,#8676,#8677,#8678,#8679,#8680,#8681,#8682,#8683,
#8684,#8685,#8686,#8687),.UNSPECIFIED.,.F.,.F.,(4,3,3,3,3,3,3,4),(-35.2623097995902,
-34.9160212588708,-33.9184206514745,-32.9208200440782,-31.9232194366819,
-30.9256188292856,-29.9280182218893,-28.9791244924106),.UNSPECIFIED.);
#1176=B_SPLINE_CURVE_WITH_KNOTS('',3,(#8692,#8693,#8694,#8695,#8696,#8697,
#8698,#8699,#8700,#8701,#8702,#8703,#8704,#8705,#8706,#8707,#8708,#8709,
#8710,#8711,#8712,#8713),.UNSPECIFIED.,.F.,.F.,(4,3,3,3,3,3,3,4),(26.4425634838903,
26.9352163997003,27.9328170070967,28.930417614493,29.9280182218893,30.9256188292856,
31.9232194366819,32.7257487910699),.UNSPECIFIED.);
#1177=B_SPLINE_CURVE_WITH_KNOTS('',3,(#8714,#8715,#8716,#8717,#8718,#8719,
#8720,#8721,#8722,#8723,#8724,#8725,#8726,#8727,#8728,#8729,#8730,#8731,
#8732,#8733,#8734,#8735,#8736,#8737,#8738),.UNSPECIFIED.,.F.,.F.,(4,3,3,
3,3,3,3,3,4),(-28.9791244924106,-28.930417614493,-27.9328170070967,-26.9352163997003,
-25.937615792304,-24.9400151849077,-23.9424145775114,-22.9448139701151,
-22.695939185231),.UNSPECIFIED.);
#1178=B_SPLINE_CURVE_WITH_KNOTS('',3,(#8743,#8744,#8745,#8746,#8747,#8748,
#8749,#8750,#8751,#8752,#8753,#8754,#8755,#8756,#8757,#8758,#8759,#8760,
#8761,#8762,#8763,#8764),.UNSPECIFIED.,.F.,.F.,(4,3,3,3,3,3,3,4),(20.1593781767107,
20.9496127553225,21.9472133627188,22.9448139701151,23.9424145775114,24.9400151849077,
25.937615792304,26.4425634838903),.UNSPECIFIED.);
#1179=B_SPLINE_CURVE_WITH_KNOTS('',3,(#8765,#8766,#8767,#8768,#8769,#8770,
#8771,#8772,#8773,#8774,#8775,#8776,#8777,#8778,#8779,#8780,#8781,#8782,
#8783,#8784,#8785,#8786),.UNSPECIFIED.,.F.,.F.,(4,3,3,3,3,3,3,4),(-22.695939185231,
-21.9472133627188,-20.9496127553225,-19.9520121479262,-18.9544115405299,
-17.9568109331336,-16.9592103257373,-16.4127538780514),.UNSPECIFIED.);
#1180=B_SPLINE_CURVE_WITH_KNOTS('',3,(#8791,#8792,#8793,#8794,#8795,#8796,
#8797,#8798,#8799,#8800,#8801,#8802,#8803,#8804,#8805,#8806,#8807,#8808,
#8809,#8810,#8811,#8812,#8813,#8814,#8815),.UNSPECIFIED.,.F.,.F.,(4,3,3,
3,3,3,3,3,4),(13.8761928695311,13.9664085035483,14.9640091109446,15.9616097183409,
16.9592103257373,17.9568109331336,18.9544115405299,19.9520121479262,20.1593781767107),
 .UNSPECIFIED.);
#1181=B_SPLINE_CURVE_WITH_KNOTS('',3,(#8816,#8817,#8818,#8819,#8820,#8821,
#8822,#8823,#8824,#8825,#8826,#8827,#8828,#8829,#8830,#8831,#8832,#8833,
#8834,#8835,#8836,#8837),.UNSPECIFIED.,.F.,.F.,(4,3,3,3,3,3,3,4),(-16.4127538780514,
-15.9616097183409,-14.9640091109446,-13.9664085035483,-12.968807896152,
-11.9712072887557,-10.9736066813594,-10.1295685708718),.UNSPECIFIED.);
#1182=B_SPLINE_CURVE_WITH_KNOTS('',3,(#8843,#8844,#8845,#8846,#8847,#8848,
#8849,#8850,#8851,#8852,#8853,#8854,#8855),.UNSPECIFIED.,.F.,.F.,(4,3,3,
3,4),(-3.84638326369224,-2.99280182218893,-1.99520121479262,-0.99760060739631,
0.),.UNSPECIFIED.);
#1183=B_SPLINE_CURVE_WITH_KNOTS('',3,(#8858,#8859,#8860,#8861,#8862,#8863,
#8864,#8865,#8866,#8867,#8868,#8869,#8870,#8871,#8872,#8873,#8874,#8875,
#8876),.UNSPECIFIED.,.F.,.F.,(4,3,3,3,3,3,4),(2.01461286527443,2.99280182218893,
3.99040242958524,4.98800303698155,5.98560364437786,6.98320425177416,7.59300756235153),
 .UNSPECIFIED.);
#1184=B_SPLINE_CURVE_WITH_KNOTS('',3,(#8882,#8883,#8884,#8885,#8886,#8887,
#8888,#8889,#8890,#8891,#8892,#8893,#8894),.UNSPECIFIED.,.F.,.F.,(4,3,3,
3,4),(70.4248606341474,70.8296431251379,71.8272437325342,72.8248443399306,
73.8224449473269),.UNSPECIFIED.);
#1185=B_SPLINE_CURVE_WITH_KNOTS('',3,(#8897,#8898,#8899,#8900,#8901,#8902,
#8903,#8904,#8905,#8906,#8907,#8908,#8909,#8910,#8911,#8912,#8913,#8914,
#8915),.UNSPECIFIED.,.F.,.F.,(4,3,3,3,3,3,4),(-71.8078320820524,-70.829643125138,
-69.8320425177416,-68.8344419103453,-67.836841302949,-66.8392406955527,
-66.6782363354882),.UNSPECIFIED.);
#1186=B_SPLINE_CURVE_WITH_KNOTS('',3,(#8920,#8921,#8922,#8923,#8924,#8925,
#8926,#8927,#8928,#8929,#8930,#8931,#8932,#8933,#8934,#8935,#8936,#8937,
#8938,#8939,#8940,#8941),.UNSPECIFIED.,.F.,.F.,(4,3,3,3,3,3,3,4),(64.1416753269678,
64.8440394807601,65.8416400881564,66.8392406955527,67.836841302949,68.8344419103453,
69.8320425177416,70.4248606341474),.UNSPECIFIED.);
#1187=B_SPLINE_CURVE_WITH_KNOTS('',3,(#8942,#8943,#8944,#8945,#8946,#8947,
#8948,#8949,#8950,#8951,#8952,#8953,#8954,#8955,#8956,#8957,#8958,#8959,
#8960,#8961,#8962,#8963),.UNSPECIFIED.,.F.,.F.,(4,3,3,3,3,3,3,4),(-66.6782363354882,
-65.8416400881564,-64.8440394807601,-63.8464388733638,-62.8488382659675,
-61.8512376585712,-60.8536370511749,-60.3950510283086),.UNSPECIFIED.);
#1188=B_SPLINE_CURVE_WITH_KNOTS('',3,(#8968,#8969,#8970,#8971,#8972,#8973,
#8974,#8975,#8976,#8977,#8978,#8979,#8980,#8981,#8982,#8983,#8984,#8985,
#8986,#8987,#8988,#8989),.UNSPECIFIED.,.F.,.F.,(4,3,3,3,3,3,3,4),(57.8584900197882,
58.8584358363822,59.8560364437785,60.8536370511749,61.8512376585712,62.8488382659675,
63.8464388733638,64.1416753269678),.UNSPECIFIED.);
#1189=B_SPLINE_CURVE_WITH_KNOTS('',3,(#8990,#8991,#8992,#8993,#8994,#8995,
#8996,#8997,#8998,#8999,#9000,#9001,#9002,#9003,#9004,#9005,#9006,#9007,
#9008,#9009,#9010,#9011),.UNSPECIFIED.,.F.,.F.,(4,3,3,3,3,3,3,4),(-60.3950510283086,
-59.8560364437785,-58.8584358363822,-57.8608352289859,-56.8632346215896,
-55.8656340141933,-54.868033406797,-54.111865721129),.UNSPECIFIED.);
#1190=B_SPLINE_CURVE_WITH_KNOTS('',3,(#9016,#9017,#9018,#9019,#9020,#9021,
#9022,#9023,#9024,#9025,#9026,#9027,#9028,#9029,#9030,#9031,#9032,#9033,
#9034,#9035,#9036,#9037),.UNSPECIFIED.,.F.,.F.,(4,3,3,3,3,3,3,4),(51.5753047126087,
51.8752315846081,52.8728321920044,53.8704327994007,54.868033406797,55.8656340141933,
56.8632346215896,57.8584900197882),.UNSPECIFIED.);
#1191=B_SPLINE_CURVE_WITH_KNOTS('',3,(#9038,#9039,#9040,#9041,#9042,#9043,
#9044,#9045,#9046,#9047,#9048,#9049,#9050,#9051,#9052,#9053,#9054,#9055,
#9056,#9057,#9058,#9059,#9060,#9061,#9062),.UNSPECIFIED.,.F.,.F.,(4,3,3,
3,3,3,3,3,4),(-54.111865721129,-53.8704327994007,-52.8728321920044,-51.8752315846081,
-50.8776309772118,-49.8800303698155,-48.8824297624191,-47.8848291550228,
-47.8286804139494),.UNSPECIFIED.);
#1192=B_SPLINE_CURVE_WITH_KNOTS('',3,(#9067,#9068,#9069,#9070,#9071,#9072,
#9073,#9074,#9075,#9076,#9077,#9078,#9079,#9080,#9081,#9082,#9083,#9084,
#9085,#9086,#9087,#9088),.UNSPECIFIED.,.F.,.F.,(4,3,3,3,3,3,3,4),(45.2921194054291,
45.8896279402302,46.8872285476265,47.8848291550228,48.8824297624192,49.8800303698155,
50.8776309772118,51.5753047126087),.UNSPECIFIED.);
#1193=B_SPLINE_CURVE_WITH_KNOTS('',3,(#9089,#9090,#9091,#9092,#9093,#9094,
#9095,#9096,#9097,#9098,#9099,#9100,#9101,#9102,#9103,#9104,#9105,#9106,
#9107,#9108,#9109,#9110),.UNSPECIFIED.,.F.,.F.,(4,3,3,3,3,3,3,4),(-47.8286804139494,
-46.8872285476265,-45.8896279402302,-44.8920273328339,-43.8944267254376,
-42.8968261180413,-41.899225510645,-41.5454951067698),.UNSPECIFIED.);
#1194=B_SPLINE_CURVE_WITH_KNOTS('',3,(#9115,#9116,#9117,#9118,#9119,#9120,
#9121,#9122,#9123,#9124,#9125,#9126,#9127,#9128,#9129,#9130,#9131,#9132,
#9133,#9134,#9135,#9136),.UNSPECIFIED.,.F.,.F.,(4,3,3,3,3,3,3,4),(39.0089340982495,
39.9040242958524,40.9016249032487,41.899225510645,42.8968261180413,43.8944267254376,
44.8920273328339,45.2921194054291),.UNSPECIFIED.);
#1195=B_SPLINE_CURVE_WITH_KNOTS('',3,(#9137,#9138,#9139,#9140,#9141,#9142,
#9143,#9144,#9145,#9146,#9147,#9148,#9149,#9150,#9151,#9152,#9153,#9154,
#9155,#9156,#9157,#9158),.UNSPECIFIED.,.F.,.F.,(4,3,3,3,3,3,3,4),(-41.5454951067698,
-40.9016249032487,-39.9040242958524,-38.9064236884561,-37.9088230810597,
-36.9112224736634,-35.9136218662671,-35.2623097995902),.UNSPECIFIED.);
#1196=B_SPLINE_CURVE_WITH_KNOTS('',3,(#9163,#9164,#9165,#9166,#9167,#9168,
#9169,#9170,#9171,#9172,#9173,#9174,#9175,#9176,#9177,#9178,#9179,#9180,
#9181,#9182,#9183,#9184,#9185,#9186,#9187),.UNSPECIFIED.,.F.,.F.,(4,3,3,
3,3,3,3,3,4),(32.7257487910699,32.9208200440782,33.9184206514745,34.9160212588708,
35.9136218662671,36.9112224736634,37.9088230810598,38.9064236884561,39.0089340982495),
 .UNSPECIFIED.);
#1197=B_SPLINE_CURVE_WITH_KNOTS('',3,(#9188,#9189,#9190,#9191,#9192,#9193,
#9194,#9195,#9196,#9197,#9198,#9199,#9200,#9201,#9202,#9203,#9204,#9205,
#9206,#9207,#9208,#9209),.UNSPECIFIED.,.F.,.F.,(4,3,3,3,3,3,3,4),(-35.2623097995902,
-34.9160212588708,-33.9184206514745,-32.9208200440782,-31.9232194366819,
-30.9256188292856,-29.9280182218893,-28.9791244924106),.UNSPECIFIED.);
#1198=B_SPLINE_CURVE_WITH_KNOTS('',3,(#9214,#9215,#9216,#9217,#9218,#9219,
#9220,#9221,#9222,#9223,#9224,#9225,#9226,#9227,#9228,#9229,#9230,#9231,
#9232,#9233,#9234,#9235),.UNSPECIFIED.,.F.,.F.,(4,3,3,3,3,3,3,4),(26.4425634838903,
26.9352163997003,27.9328170070967,28.930417614493,29.9280182218893,30.9256188292856,
31.9232194366819,32.7257487910699),.UNSPECIFIED.);
#1199=B_SPLINE_CURVE_WITH_KNOTS('',3,(#9236,#9237,#9238,#9239,#9240,#9241,
#9242,#9243,#9244,#9245,#9246,#9247,#9248,#9249,#9250,#9251,#9252,#9253,
#9254,#9255,#9256,#9257,#9258,#9259,#9260),.UNSPECIFIED.,.F.,.F.,(4,3,3,
3,3,3,3,3,4),(-28.9791244924106,-28.930417614493,-27.9328170070967,-26.9352163997003,
-25.937615792304,-24.9400151849077,-23.9424145775114,-22.9448139701151,
-22.695939185231),.UNSPECIFIED.);
#1200=B_SPLINE_CURVE_WITH_KNOTS('',3,(#9265,#9266,#9267,#9268,#9269,#9270,
#9271,#9272,#9273,#9274,#9275,#9276,#9277,#9278,#9279,#9280,#9281,#9282,
#9283,#9284,#9285,#9286),.UNSPECIFIED.,.F.,.F.,(4,3,3,3,3,3,3,4),(20.1593781767107,
20.9496127553225,21.9472133627188,22.9448139701151,23.9424145775114,24.9400151849077,
25.937615792304,26.4425634838903),.UNSPECIFIED.);
#1201=B_SPLINE_CURVE_WITH_KNOTS('',3,(#9287,#9288,#9289,#9290,#9291,#9292,
#9293,#9294,#9295,#9296,#9297,#9298,#9299,#9300,#9301,#9302,#9303,#9304,
#9305,#9306,#9307,#9308),.UNSPECIFIED.,.F.,.F.,(4,3,3,3,3,3,3,4),(-22.695939185231,
-21.9472133627188,-20.9496127553225,-19.9520121479262,-18.9544115405299,
-17.9568109331336,-16.9592103257373,-16.4127538780514),.UNSPECIFIED.);
#1202=B_SPLINE_CURVE_WITH_KNOTS('',3,(#9313,#9314,#9315,#9316,#9317,#9318,
#9319,#9320,#9321,#9322,#9323,#9324,#9325,#9326,#9327,#9328,#9329,#9330,
#9331,#9332,#9333,#9334,#9335,#9336,#9337),.UNSPECIFIED.,.F.,.F.,(4,3,3,
3,3,3,3,3,4),(13.8761928695311,13.9664085035483,14.9640091109446,15.9616097183409,
16.9592103257373,17.9568109331336,18.9544115405299,19.9520121479262,20.1593781767107),
 .UNSPECIFIED.);
#1203=B_SPLINE_CURVE_WITH_KNOTS('',3,(#9338,#9339,#9340,#9341,#9342,#9343,
#9344,#9345,#9346,#9347,#9348,#9349,#9350,#9351,#9352,#9353,#9354,#9355,
#9356,#9357,#9358,#9359),.UNSPECIFIED.,.F.,.F.,(4,3,3,3,3,3,3,4),(-16.4127538780514,
-15.9616097183409,-14.9640091109446,-13.9664085035483,-12.968807896152,
-11.9712072887557,-10.9736066813594,-10.1295685708718),.UNSPECIFIED.);
#1204=B_SPLINE_CURVE_WITH_KNOTS('',3,(#9365,#9366,#9367,#9368,#9369,#9370,
#9371,#9372,#9373,#9374,#9375,#9376,#9377),.UNSPECIFIED.,.F.,.F.,(4,3,3,
3,4),(-3.84638326369225,-2.99280182218893,-1.99520121479262,-0.997600607396308,
0.),.UNSPECIFIED.);
#1205=B_SPLINE_CURVE_WITH_KNOTS('',3,(#9380,#9381,#9382,#9383,#9384,#9385,
#9386,#9387,#9388,#9389,#9390,#9391,#9392,#9393,#9394,#9395,#9396,#9397,
#9398),.UNSPECIFIED.,.F.,.F.,(4,3,3,3,3,3,4),(2.01461286527445,2.99280182218893,
3.99040242958524,4.98800303698155,5.98560364437786,6.98320425177416,7.59300756235153),
 .UNSPECIFIED.);
#1206=B_SPLINE_CURVE_WITH_KNOTS('',3,(#9404,#9405,#9406,#9407,#9408,#9409,
#9410,#9411,#9412,#9413,#9414,#9415,#9416),.UNSPECIFIED.,.F.,.F.,(4,3,3,
3,4),(70.4248606341474,70.8296431251379,71.8272437325342,72.8248443399306,
73.8224449473269),.UNSPECIFIED.);
#1207=B_SPLINE_CURVE_WITH_KNOTS('',3,(#9419,#9420,#9421,#9422,#9423,#9424,
#9425,#9426,#9427,#9428,#9429,#9430,#9431,#9432,#9433,#9434,#9435,#9436,
#9437),.UNSPECIFIED.,.F.,.F.,(4,3,3,3,3,3,4),(-71.8078320820524,-70.829643125138,
-69.8320425177417,-68.8344419103453,-67.836841302949,-66.8392406955527,
-66.6782363354881),.UNSPECIFIED.);
#1208=B_SPLINE_CURVE_WITH_KNOTS('',3,(#9442,#9443,#9444,#9445,#9446,#9447,
#9448,#9449,#9450,#9451,#9452,#9453,#9454,#9455,#9456,#9457,#9458,#9459,
#9460,#9461,#9462,#9463),.UNSPECIFIED.,.F.,.F.,(4,3,3,3,3,3,3,4),(64.1416753269678,
64.8440394807601,65.8416400881564,66.8392406955527,67.836841302949,68.8344419103453,
69.8320425177416,70.4248606341474),.UNSPECIFIED.);
#1209=B_SPLINE_CURVE_WITH_KNOTS('',3,(#9464,#9465,#9466,#9467,#9468,#9469,
#9470,#9471,#9472,#9473,#9474,#9475,#9476,#9477,#9478,#9479,#9480,#9481,
#9482,#9483,#9484,#9485),.UNSPECIFIED.,.F.,.F.,(4,3,3,3,3,3,3,4),(-66.6782363354881,
-65.8416400881564,-64.8440394807601,-63.8464388733638,-62.8488382659675,
-61.8512376585712,-60.8536370511749,-60.3950510283085),.UNSPECIFIED.);
#1210=B_SPLINE_CURVE_WITH_KNOTS('',3,(#9490,#9491,#9492,#9493,#9494,#9495,
#9496,#9497,#9498,#9499,#9500,#9501,#9502,#9503,#9504,#9505,#9506,#9507,
#9508,#9509,#9510,#9511),.UNSPECIFIED.,.F.,.F.,(4,3,3,3,3,3,3,4),(57.8584900197882,
58.8584358363823,59.8560364437786,60.8536370511749,61.8512376585712,62.8488382659675,
63.8464388733638,64.1416753269678),.UNSPECIFIED.);
#1211=B_SPLINE_CURVE_WITH_KNOTS('',3,(#9512,#9513,#9514,#9515,#9516,#9517,
#9518,#9519,#9520,#9521,#9522,#9523,#9524,#9525,#9526,#9527,#9528,#9529,
#9530,#9531,#9532,#9533),.UNSPECIFIED.,.F.,.F.,(4,3,3,3,3,3,3,4),(-60.3950510283085,
-59.8560364437786,-58.8584358363823,-57.8608352289859,-56.8632346215896,
-55.8656340141933,-54.868033406797,-54.111865721129),.UNSPECIFIED.);
#1212=B_SPLINE_CURVE_WITH_KNOTS('',3,(#9538,#9539,#9540,#9541,#9542,#9543,
#9544,#9545,#9546,#9547,#9548,#9549,#9550,#9551,#9552,#9553,#9554,#9555,
#9556,#9557,#9558,#9559),.UNSPECIFIED.,.F.,.F.,(4,3,3,3,3,3,3,4),(51.5753047126087,
51.8752315846081,52.8728321920044,53.8704327994007,54.868033406797,55.8656340141933,
56.8632346215896,57.8584900197882),.UNSPECIFIED.);
#1213=B_SPLINE_CURVE_WITH_KNOTS('',3,(#9560,#9561,#9562,#9563,#9564,#9565,
#9566,#9567,#9568,#9569,#9570,#9571,#9572,#9573,#9574,#9575,#9576,#9577,
#9578,#9579,#9580,#9581,#9582,#9583,#9584),.UNSPECIFIED.,.F.,.F.,(4,3,3,
3,3,3,3,3,4),(-54.111865721129,-53.8704327994007,-52.8728321920044,-51.8752315846081,
-50.8776309772118,-49.8800303698155,-48.8824297624192,-47.8848291550228,
-47.8286804139494),.UNSPECIFIED.);
#1214=B_SPLINE_CURVE_WITH_KNOTS('',3,(#9589,#9590,#9591,#9592,#9593,#9594,
#9595,#9596,#9597,#9598,#9599,#9600,#9601,#9602,#9603,#9604,#9605,#9606,
#9607,#9608,#9609,#9610),.UNSPECIFIED.,.F.,.F.,(4,3,3,3,3,3,3,4),(45.2921194054291,
45.8896279402302,46.8872285476265,47.8848291550228,48.8824297624192,49.8800303698155,
50.8776309772118,51.5753047126087),.UNSPECIFIED.);
#1215=B_SPLINE_CURVE_WITH_KNOTS('',3,(#9611,#9612,#9613,#9614,#9615,#9616,
#9617,#9618,#9619,#9620,#9621,#9622,#9623,#9624,#9625,#9626,#9627,#9628,
#9629,#9630,#9631,#9632),.UNSPECIFIED.,.F.,.F.,(4,3,3,3,3,3,3,4),(-47.8286804139494,
-46.8872285476265,-45.8896279402302,-44.8920273328339,-43.8944267254376,
-42.8968261180413,-41.899225510645,-41.5454951067698),.UNSPECIFIED.);
#1216=B_SPLINE_CURVE_WITH_KNOTS('',3,(#9637,#9638,#9639,#9640,#9641,#9642,
#9643,#9644,#9645,#9646,#9647,#9648,#9649,#9650,#9651,#9652,#9653,#9654,
#9655,#9656,#9657,#9658),.UNSPECIFIED.,.F.,.F.,(4,3,3,3,3,3,3,4),(39.0089340982495,
39.9040242958524,40.9016249032487,41.899225510645,42.8968261180413,43.8944267254376,
44.8920273328339,45.2921194054291),.UNSPECIFIED.);
#1217=B_SPLINE_CURVE_WITH_KNOTS('',3,(#9659,#9660,#9661,#9662,#9663,#9664,
#9665,#9666,#9667,#9668,#9669,#9670,#9671,#9672,#9673,#9674,#9675,#9676,
#9677,#9678,#9679,#9680),.UNSPECIFIED.,.F.,.F.,(4,3,3,3,3,3,3,4),(-41.5454951067698,
-40.9016249032487,-39.9040242958524,-38.9064236884561,-37.9088230810597,
-36.9112224736634,-35.9136218662671,-35.2623097995902),.UNSPECIFIED.);
#1218=B_SPLINE_CURVE_WITH_KNOTS('',3,(#9685,#9686,#9687,#9688,#9689,#9690,
#9691,#9692,#9693,#9694,#9695,#9696,#9697,#9698,#9699,#9700,#9701,#9702,
#9703,#9704,#9705,#9706,#9707,#9708,#9709),.UNSPECIFIED.,.F.,.F.,(4,3,3,
3,3,3,3,3,4),(32.7257487910699,32.9208200440782,33.9184206514745,34.9160212588708,
35.9136218662671,36.9112224736634,37.9088230810597,38.9064236884561,39.0089340982495),
 .UNSPECIFIED.);
#1219=B_SPLINE_CURVE_WITH_KNOTS('',3,(#9710,#9711,#9712,#9713,#9714,#9715,
#9716,#9717,#9718,#9719,#9720,#9721,#9722,#9723,#9724,#9725,#9726,#9727,
#9728,#9729,#9730,#9731),.UNSPECIFIED.,.F.,.F.,(4,3,3,3,3,3,3,4),(-35.2623097995902,
-34.9160212588708,-33.9184206514745,-32.9208200440782,-31.9232194366819,
-30.9256188292856,-29.9280182218893,-28.9791244924106),.UNSPECIFIED.);
#1220=B_SPLINE_CURVE_WITH_KNOTS('',3,(#9736,#9737,#9738,#9739,#9740,#9741,
#9742,#9743,#9744,#9745,#9746,#9747,#9748,#9749,#9750,#9751,#9752,#9753,
#9754,#9755,#9756,#9757),.UNSPECIFIED.,.F.,.F.,(4,3,3,3,3,3,3,4),(26.4425634838903,
26.9352163997003,27.9328170070966,28.930417614493,29.9280182218893,30.9256188292856,
31.9232194366819,32.7257487910699),.UNSPECIFIED.);
#1221=B_SPLINE_CURVE_WITH_KNOTS('',3,(#9758,#9759,#9760,#9761,#9762,#9763,
#9764,#9765,#9766,#9767,#9768,#9769,#9770,#9771,#9772,#9773,#9774,#9775,
#9776,#9777,#9778,#9779,#9780,#9781,#9782),.UNSPECIFIED.,.F.,.F.,(4,3,3,
3,3,3,3,3,4),(-28.9791244924106,-28.930417614493,-27.9328170070967,-26.9352163997004,
-25.937615792304,-24.9400151849077,-23.9424145775114,-22.9448139701151,
-22.695939185231),.UNSPECIFIED.);
#1222=B_SPLINE_CURVE_WITH_KNOTS('',3,(#9787,#9788,#9789,#9790,#9791,#9792,
#9793,#9794,#9795,#9796,#9797,#9798,#9799,#9800,#9801,#9802,#9803,#9804,
#9805,#9806,#9807,#9808),.UNSPECIFIED.,.F.,.F.,(4,3,3,3,3,3,3,4),(20.1593781767107,
20.9496127553225,21.9472133627188,22.9448139701151,23.9424145775114,24.9400151849077,
25.937615792304,26.4425634838903),.UNSPECIFIED.);
#1223=B_SPLINE_CURVE_WITH_KNOTS('',3,(#9809,#9810,#9811,#9812,#9813,#9814,
#9815,#9816,#9817,#9818,#9819,#9820,#9821,#9822,#9823,#9824,#9825,#9826,
#9827,#9828,#9829,#9830),.UNSPECIFIED.,.F.,.F.,(4,3,3,3,3,3,3,4),(-22.695939185231,
-21.9472133627188,-20.9496127553225,-19.9520121479262,-18.9544115405299,
-17.9568109331336,-16.9592103257373,-16.4127538780514),.UNSPECIFIED.);
#1224=B_SPLINE_CURVE_WITH_KNOTS('',3,(#9835,#9836,#9837,#9838,#9839,#9840,
#9841,#9842,#9843,#9844,#9845,#9846,#9847,#9848,#9849,#9850,#9851,#9852,
#9853,#9854,#9855,#9856,#9857,#9858,#9859),.UNSPECIFIED.,.F.,.F.,(4,3,3,
3,3,3,3,3,4),(13.8761928695311,13.9664085035483,14.9640091109446,15.9616097183409,
16.9592103257373,17.9568109331336,18.9544115405299,19.9520121479262,20.1593781767107),
 .UNSPECIFIED.);
#1225=B_SPLINE_CURVE_WITH_KNOTS('',3,(#9860,#9861,#9862,#9863,#9864,#9865,
#9866,#9867,#9868,#9869,#9870,#9871,#9872,#9873,#9874,#9875,#9876,#9877,
#9878,#9879,#9880,#9881),.UNSPECIFIED.,.F.,.F.,(4,3,3,3,3,3,3,4),(-16.4127538780514,
-15.9616097183409,-14.9640091109446,-13.9664085035483,-12.968807896152,
-11.9712072887557,-10.9736066813594,-10.1295685708718),.UNSPECIFIED.);
#1226=B_SPLINE_CURVE_WITH_KNOTS('',3,(#9887,#9888,#9889,#9890,#9891,#9892,
#9893,#9894,#9895,#9896,#9897,#9898,#9899),.UNSPECIFIED.,.F.,.F.,(4,3,3,
3,4),(-3.84638326369224,-2.99280182218893,-1.99520121479262,-0.99760060739631,
0.),.UNSPECIFIED.);
#1227=B_SPLINE_CURVE_WITH_KNOTS('',3,(#9904,#9905,#9906,#9907,#9908,#9909,
#9910,#9911,#9912,#9913,#9914,#9915,#9916,#9917,#9918,#9919,#9920,#9921,
#9922),.UNSPECIFIED.,.F.,.F.,(4,3,3,3,3,3,4),(2.01461286527445,2.99280182218893,
3.99040242958524,4.98800303698155,5.98560364437786,6.98320425177417,7.59300756235153),
 .UNSPECIFIED.);
#1228=B_SPLINE_CURVE_WITH_KNOTS('',3,(#9928,#9929,#9930,#9931,#9932,#9933,
#9934,#9935,#9936,#9937,#9938,#9939,#9940),.UNSPECIFIED.,.F.,.F.,(4,3,3,
3,4),(70.4248606341474,70.8296431251379,71.8272437325342,72.8248443399306,
73.8224449473269),.UNSPECIFIED.);
#1229=B_SPLINE_CURVE_WITH_KNOTS('',3,(#9943,#9944,#9945,#9946,#9947,#9948,
#9949,#9950,#9951,#9952,#9953,#9954,#9955,#9956,#9957,#9958,#9959,#9960,
#9961),.UNSPECIFIED.,.F.,.F.,(4,3,3,3,3,3,4),(-71.8078320820524,-70.8296431251379,
-69.8320425177416,-68.8344419103453,-67.836841302949,-66.8392406955527,
-66.6782363354881),.UNSPECIFIED.);
#1230=B_SPLINE_CURVE_WITH_KNOTS('',3,(#9966,#9967,#9968,#9969,#9970,#9971,
#9972,#9973,#9974,#9975,#9976,#9977,#9978,#9979,#9980,#9981,#9982,#9983,
#9984,#9985,#9986,#9987),.UNSPECIFIED.,.F.,.F.,(4,3,3,3,3,3,3,4),(64.1416753269678,
64.8440394807601,65.8416400881564,66.8392406955527,67.836841302949,68.8344419103453,
69.8320425177416,70.4248606341474),.UNSPECIFIED.);
#1231=B_SPLINE_CURVE_WITH_KNOTS('',3,(#9988,#9989,#9990,#9991,#9992,#9993,
#9994,#9995,#9996,#9997,#9998,#9999,#10000,#10001,#10002,#10003,#10004,
#10005,#10006,#10007,#10008,#10009),.UNSPECIFIED.,.F.,.F.,(4,3,3,3,3,3,
3,4),(-66.6782363354881,-65.8416400881564,-64.8440394807601,-63.8464388733638,
-62.8488382659675,-61.8512376585712,-60.8536370511749,-60.3950510283085),
 .UNSPECIFIED.);
#1232=B_SPLINE_CURVE_WITH_KNOTS('',3,(#10014,#10015,#10016,#10017,#10018,
#10019,#10020,#10021,#10022,#10023,#10024,#10025,#10026,#10027,#10028,#10029,
#10030,#10031,#10032,#10033,#10034,#10035),.UNSPECIFIED.,.F.,.F.,(4,3,3,
3,3,3,3,4),(57.8584900197882,58.8584358363823,59.8560364437786,60.8536370511749,
61.8512376585712,62.8488382659675,63.8464388733638,64.1416753269678),
 .UNSPECIFIED.);
#1233=B_SPLINE_CURVE_WITH_KNOTS('',3,(#10036,#10037,#10038,#10039,#10040,
#10041,#10042,#10043,#10044,#10045,#10046,#10047,#10048,#10049,#10050,#10051,
#10052,#10053,#10054,#10055,#10056,#10057),.UNSPECIFIED.,.F.,.F.,(4,3,3,
3,3,3,3,4),(-60.3950510283085,-59.8560364437785,-58.8584358363822,-57.8608352289859,
-56.8632346215896,-55.8656340141933,-54.868033406797,-54.111865721129),
 .UNSPECIFIED.);
#1234=B_SPLINE_CURVE_WITH_KNOTS('',3,(#10062,#10063,#10064,#10065,#10066,
#10067,#10068,#10069,#10070,#10071,#10072,#10073,#10074,#10075,#10076,#10077,
#10078,#10079,#10080,#10081,#10082,#10083),.UNSPECIFIED.,.F.,.F.,(4,3,3,
3,3,3,3,4),(51.5753047126087,51.8752315846081,52.8728321920044,53.8704327994007,
54.868033406797,55.8656340141933,56.8632346215896,57.8584900197882),
 .UNSPECIFIED.);
#1235=B_SPLINE_CURVE_WITH_KNOTS('',3,(#10084,#10085,#10086,#10087,#10088,
#10089,#10090,#10091,#10092,#10093,#10094,#10095,#10096,#10097,#10098,#10099,
#10100,#10101,#10102,#10103,#10104,#10105,#10106,#10107,#10108),
 .UNSPECIFIED.,.F.,.F.,(4,3,3,3,3,3,3,3,4),(-54.111865721129,-53.8704327994007,
-52.8728321920044,-51.8752315846081,-50.8776309772118,-49.8800303698155,
-48.8824297624191,-47.8848291550228,-47.8286804139494),.UNSPECIFIED.);
#1236=B_SPLINE_CURVE_WITH_KNOTS('',3,(#10113,#10114,#10115,#10116,#10117,
#10118,#10119,#10120,#10121,#10122,#10123,#10124,#10125,#10126,#10127,#10128,
#10129,#10130,#10131,#10132,#10133,#10134),.UNSPECIFIED.,.F.,.F.,(4,3,3,
3,3,3,3,4),(45.2921194054291,45.8896279402302,46.8872285476265,47.8848291550228,
48.8824297624192,49.8800303698155,50.8776309772118,51.5753047126087),
 .UNSPECIFIED.);
#1237=B_SPLINE_CURVE_WITH_KNOTS('',3,(#10135,#10136,#10137,#10138,#10139,
#10140,#10141,#10142,#10143,#10144,#10145,#10146,#10147,#10148,#10149,#10150,
#10151,#10152,#10153,#10154,#10155,#10156),.UNSPECIFIED.,.F.,.F.,(4,3,3,
3,3,3,3,4),(-47.8286804139494,-46.8872285476265,-45.8896279402302,-44.8920273328339,
-43.8944267254376,-42.8968261180413,-41.899225510645,-41.5454951067698),
 .UNSPECIFIED.);
#1238=B_SPLINE_CURVE_WITH_KNOTS('',3,(#10161,#10162,#10163,#10164,#10165,
#10166,#10167,#10168,#10169,#10170,#10171,#10172,#10173,#10174,#10175,#10176,
#10177,#10178,#10179,#10180,#10181,#10182),.UNSPECIFIED.,.F.,.F.,(4,3,3,
3,3,3,3,4),(39.0089340982495,39.9040242958524,40.9016249032487,41.899225510645,
42.8968261180413,43.8944267254376,44.8920273328339,45.2921194054291),
 .UNSPECIFIED.);
#1239=B_SPLINE_CURVE_WITH_KNOTS('',3,(#10183,#10184,#10185,#10186,#10187,
#10188,#10189,#10190,#10191,#10192,#10193,#10194,#10195,#10196,#10197,#10198,
#10199,#10200,#10201,#10202,#10203,#10204),.UNSPECIFIED.,.F.,.F.,(4,3,3,
3,3,3,3,4),(-41.5454951067698,-40.9016249032487,-39.9040242958524,-38.9064236884561,
-37.9088230810597,-36.9112224736634,-35.9136218662671,-35.2623097995902),
 .UNSPECIFIED.);
#1240=B_SPLINE_CURVE_WITH_KNOTS('',3,(#10209,#10210,#10211,#10212,#10213,
#10214,#10215,#10216,#10217,#10218,#10219,#10220,#10221,#10222,#10223,#10224,
#10225,#10226,#10227,#10228,#10229,#10230,#10231,#10232,#10233),
 .UNSPECIFIED.,.F.,.F.,(4,3,3,3,3,3,3,3,4),(32.7257487910699,32.9208200440782,
33.9184206514745,34.9160212588708,35.9136218662671,36.9112224736634,37.9088230810597,
38.9064236884561,39.0089340982495),.UNSPECIFIED.);
#1241=B_SPLINE_CURVE_WITH_KNOTS('',3,(#10234,#10235,#10236,#10237,#10238,
#10239,#10240,#10241,#10242,#10243,#10244,#10245,#10246,#10247,#10248,#10249,
#10250,#10251,#10252,#10253,#10254,#10255),.UNSPECIFIED.,.F.,.F.,(4,3,3,
3,3,3,3,4),(-35.2623097995902,-34.9160212588708,-33.9184206514745,-32.9208200440782,
-31.9232194366819,-30.9256188292856,-29.9280182218893,-28.9791244924106),
 .UNSPECIFIED.);
#1242=B_SPLINE_CURVE_WITH_KNOTS('',3,(#10260,#10261,#10262,#10263,#10264,
#10265,#10266,#10267,#10268,#10269,#10270,#10271,#10272,#10273,#10274,#10275,
#10276,#10277,#10278,#10279,#10280,#10281),.UNSPECIFIED.,.F.,.F.,(4,3,3,
3,3,3,3,4),(26.4425634838903,26.9352163997003,27.9328170070967,28.930417614493,
29.9280182218893,30.9256188292856,31.9232194366819,32.7257487910699),
 .UNSPECIFIED.);
#1243=B_SPLINE_CURVE_WITH_KNOTS('',3,(#10282,#10283,#10284,#10285,#10286,
#10287,#10288,#10289,#10290,#10291,#10292,#10293,#10294,#10295,#10296,#10297,
#10298,#10299,#10300,#10301,#10302,#10303,#10304,#10305,#10306),
 .UNSPECIFIED.,.F.,.F.,(4,3,3,3,3,3,3,3,4),(-28.9791244924106,-28.930417614493,
-27.9328170070967,-26.9352163997003,-25.937615792304,-24.9400151849077,
-23.9424145775114,-22.9448139701151,-22.695939185231),.UNSPECIFIED.);
#1244=B_SPLINE_CURVE_WITH_KNOTS('',3,(#10311,#10312,#10313,#10314,#10315,
#10316,#10317,#10318,#10319,#10320,#10321,#10322,#10323,#10324,#10325,#10326,
#10327,#10328,#10329,#10330,#10331,#10332),.UNSPECIFIED.,.F.,.F.,(4,3,3,
3,3,3,3,4),(20.1593781767107,20.9496127553225,21.9472133627188,22.9448139701151,
23.9424145775114,24.9400151849077,25.937615792304,26.4425634838903),
 .UNSPECIFIED.);
#1245=B_SPLINE_CURVE_WITH_KNOTS('',3,(#10333,#10334,#10335,#10336,#10337,
#10338,#10339,#10340,#10341,#10342,#10343,#10344,#10345,#10346,#10347,#10348,
#10349,#10350,#10351,#10352,#10353,#10354),.UNSPECIFIED.,.F.,.F.,(4,3,3,
3,3,3,3,4),(-22.695939185231,-21.9472133627188,-20.9496127553225,-19.9520121479262,
-18.9544115405299,-17.9568109331336,-16.9592103257372,-16.4127538780514),
 .UNSPECIFIED.);
#1246=B_SPLINE_CURVE_WITH_KNOTS('',3,(#10359,#10360,#10361,#10362,#10363,
#10364,#10365,#10366,#10367,#10368,#10369,#10370,#10371,#10372,#10373,#10374,
#10375,#10376,#10377,#10378,#10379,#10380,#10381,#10382,#10383),
 .UNSPECIFIED.,.F.,.F.,(4,3,3,3,3,3,3,3,4),(13.8761928695311,13.9664085035483,
14.9640091109446,15.9616097183409,16.9592103257373,17.9568109331336,18.9544115405299,
19.9520121479262,20.1593781767107),.UNSPECIFIED.);
#1247=B_SPLINE_CURVE_WITH_KNOTS('',3,(#10384,#10385,#10386,#10387,#10388,
#10389,#10390,#10391,#10392,#10393,#10394,#10395,#10396,#10397,#10398,#10399,
#10400,#10401,#10402,#10403,#10404,#10405),.UNSPECIFIED.,.F.,.F.,(4,3,3,
3,3,3,3,4),(-16.4127538780514,-15.9616097183409,-14.9640091109446,-13.9664085035483,
-12.968807896152,-11.9712072887557,-10.9736066813594,-10.1295685708718),
 .UNSPECIFIED.);
#1248=B_SPLINE_CURVE_WITH_KNOTS('',3,(#10411,#10412,#10413,#10414,#10415,
#10416,#10417,#10418,#10419,#10420,#10421,#10422,#10423),.UNSPECIFIED.,
 .F.,.F.,(4,3,3,3,4),(-3.84638326369224,-2.99280182218893,-1.99520121479262,
-0.99760060739631,0.),.UNSPECIFIED.);
#1249=B_SPLINE_CURVE_WITH_KNOTS('',3,(#10428,#10429,#10430,#10431,#10432,
#10433,#10434,#10435,#10436,#10437,#10438,#10439,#10440,#10441,#10442,#10443,
#10444,#10445,#10446),.UNSPECIFIED.,.F.,.F.,(4,3,3,3,3,3,4),(2.01461286527445,
2.99280182218893,3.99040242958524,4.98800303698155,5.98560364437786,6.98320425177417,
7.59300756235153),.UNSPECIFIED.);
#1250=B_SPLINE_CURVE_WITH_KNOTS('',3,(#10452,#10453,#10454,#10455),
 .UNSPECIFIED.,.F.,.F.,(4,4),(84.8230016469244,85.6840249515836),
 .UNSPECIFIED.);
#1251=B_SPLINE_CURVE_WITH_KNOTS('',3,(#10458,#10459,#10460,#10461,#10462),
 .UNSPECIFIED.,.F.,.F.,(4,1,4),(84.8230016469244,85.2277841379149,86.2059730948294),
 .UNSPECIFIED.);
#1252=B_SPLINE_CURVE_WITH_KNOTS('',3,(#10467,#10468,#10469,#10470,#10471,
#10472,#10473,#10474,#10475,#10476,#10477),.UNSPECIFIED.,.F.,.F.,(4,1,1,
1,1,1,1,1,4),(78.5398163397448,78.7008206998094,79.6984213072057,80.696021914602,
81.6936225219983,82.6912231293946,83.688823736791,84.6864243441873,84.8230016469244),
 .UNSPECIFIED.);
#1253=B_SPLINE_CURVE_WITH_KNOTS('',3,(#10478,#10479,#10480,#10481,#10482,
#10483,#10484,#10485,#10486,#10487),.UNSPECIFIED.,.F.,.F.,(4,1,1,1,1,1,
1,4),(78.5398163397448,79.242180493537,80.2397811009333,81.2373817083296,
82.2349823157259,83.2325829231223,84.2301835305186,84.8230016469244),
 .UNSPECIFIED.);
#1254=B_SPLINE_CURVE_WITH_KNOTS('',3,(#10492,#10493,#10494,#10495,#10496,
#10497,#10498,#10499,#10500,#10501),.UNSPECIFIED.,.F.,.F.,(4,1,1,1,1,1,
1,4),(72.2566310325652,72.7152170554315,73.7128176628279,74.7104182702242,
75.7080188776205,76.7056194850168,77.7032200924131,78.5398163397448),
 .UNSPECIFIED.);
#1255=B_SPLINE_CURVE_WITH_KNOTS('',3,(#10502,#10503,#10504,#10505,#10506,
#10507,#10508,#10509,#10510,#10511,#10512),.UNSPECIFIED.,.F.,.F.,(4,1,1,
1,1,1,1,1,4),(72.2566310325652,72.2589762417629,73.2565768491592,74.2541774565555,
75.2517780639518,76.2493786713481,77.2469792787444,78.2445798861407,78.5398163397448),
 .UNSPECIFIED.);
#1256=B_SPLINE_CURVE_WITH_KNOTS('',3,(#10517,#10518,#10519,#10520,#10521,
#10522,#10523,#10524,#10525,#10526),.UNSPECIFIED.,.F.,.F.,(4,1,1,1,1,1,
1,4),(65.9734457253856,66.7296134110537,67.72721401845,68.7248146258463,
69.7224152332426,70.7200158406389,71.7176164480352,72.2566310325652),
 .UNSPECIFIED.);
#1257=B_SPLINE_CURVE_WITH_KNOTS('',3,(#10527,#10528,#10529,#10530,#10531,
#10532,#10533,#10534,#10535,#10536),.UNSPECIFIED.,.F.,.F.,(4,1,1,1,1,1,
1,4),(65.9734457253856,66.273372597385,67.2709732047813,68.2685738121776,
69.2661744195739,70.2637750269702,71.2613756343666,72.2566310325652),
 .UNSPECIFIED.);
#1258=B_SPLINE_CURVE_WITH_KNOTS('',3,(#10541,#10542,#10543,#10544,#10545,
#10546,#10547,#10548,#10549,#10550,#10551),.UNSPECIFIED.,.F.,.F.,(4,1,1,
1,1,1,1,1,4),(59.690260418206,59.7464091592795,60.7440097666758,61.7416103740721,
62.7392109814685,63.7368115888648,64.7344121962611,65.7320128036574,65.9734457253856),
 .UNSPECIFIED.);
#1259=B_SPLINE_CURVE_WITH_KNOTS('',3,(#10552,#10553,#10554,#10555,#10556,
#10557,#10558,#10559,#10560,#10561),.UNSPECIFIED.,.F.,.F.,(4,1,1,1,1,1,
1,4),(59.6902604182061,60.2877689530072,61.2853695604035,62.2829701677998,
63.2805707751961,64.2781713825924,65.2757719899887,65.9734457253856),
 .UNSPECIFIED.);
#1260=B_SPLINE_CURVE_WITH_KNOTS('',3,(#10566,#10567,#10568,#10569,#10570,
#10571,#10572,#10573,#10574,#10575),.UNSPECIFIED.,.F.,.F.,(4,1,1,1,1,1,
1,4),(53.4070751110265,53.7608055149017,54.758406122298,55.7560067296943,
56.7536073370906,57.7512079444869,58.7488085518832,59.690260418206),
 .UNSPECIFIED.);
#1261=B_SPLINE_CURVE_WITH_KNOTS('',3,(#10576,#10577,#10578,#10579,#10580,
#10581,#10582,#10583,#10584,#10585),.UNSPECIFIED.,.F.,.F.,(4,1,1,1,1,1,
1,4),(53.4070751110265,54.3021653086293,55.2997659160256,56.2973665234219,
57.2949671308182,58.2925677382145,59.2901683456108,59.6902604182061),
 .UNSPECIFIED.);
#1262=B_SPLINE_CURVE_WITH_KNOTS('',3,(#10590,#10591,#10592,#10593,#10594,
#10595,#10596,#10597,#10598,#10599),.UNSPECIFIED.,.F.,.F.,(4,1,1,1,1,1,
1,4),(47.1238898038469,47.7752018705238,48.7728024779201,49.7704030853164,
50.7680036927127,51.7656043001091,52.7632049075054,53.4070751110265),
 .UNSPECIFIED.);
#1263=B_SPLINE_CURVE_WITH_KNOTS('',3,(#10600,#10601,#10602,#10603,#10604,
#10605,#10606,#10607,#10608,#10609,#10610),.UNSPECIFIED.,.F.,.F.,(4,1,1,
1,1,1,1,1,4),(47.1238898038469,47.3189610568551,48.3165616642514,49.3141622716478,
50.3117628790441,51.3093634864404,52.3069640938367,53.304564701233,53.4070751110265),
 .UNSPECIFIED.);
#1264=B_SPLINE_CURVE_WITH_KNOTS('',3,(#10615,#10616,#10617,#10618,#10619,
#10620,#10621,#10622,#10623,#10624),.UNSPECIFIED.,.F.,.F.,(4,1,1,1,1,1,
1,4),(40.8407044966673,41.789598226146,42.7871988335423,43.7847994409386,
44.7824000483349,45.7800006557312,46.7776012631275,47.1238898038469),
 .UNSPECIFIED.);
#1265=B_SPLINE_CURVE_WITH_KNOTS('',3,(#10625,#10626,#10627,#10628,#10629,
#10630,#10631,#10632,#10633,#10634),.UNSPECIFIED.,.F.,.F.,(4,1,1,1,1,1,
1,4),(40.8407044966673,41.3333574124773,42.3309580198736,43.3285586272699,
44.3261592346662,45.3237598420625,46.3213604494588,47.1238898038469),
 .UNSPECIFIED.);
#1266=B_SPLINE_CURVE_WITH_KNOTS('',3,(#10639,#10640,#10641,#10642,#10643,
#10644,#10645,#10646,#10647,#10648,#10649),.UNSPECIFIED.,.F.,.F.,(4,1,1,
1,1,1,1,1,4),(34.5575191894877,34.8063939743718,35.8039945817681,36.8015951891644,
37.7991957965607,38.796796403957,39.7943970113533,40.7919976187497,40.8407044966673),
 .UNSPECIFIED.);
#1267=B_SPLINE_CURVE_WITH_KNOTS('',3,(#10650,#10651,#10652,#10653,#10654,
#10655,#10656,#10657,#10658,#10659),.UNSPECIFIED.,.F.,.F.,(4,1,1,1,1,1,
1,4),(34.5575191894877,35.3477537680994,36.3453543754957,37.342954982892,
38.3405555902884,39.3381561976847,40.335756805081,40.8407044966673),
 .UNSPECIFIED.);
#1268=B_SPLINE_CURVE_WITH_KNOTS('',3,(#10664,#10665,#10666,#10667,#10668,
#10669,#10670,#10671,#10672,#10673),.UNSPECIFIED.,.F.,.F.,(4,1,1,1,1,1,
1,4),(28.2743338823081,28.8207903299939,29.8183909373903,30.8159915447866,
31.8135921521829,32.8111927595792,33.8087933669755,34.5575191894877),
 .UNSPECIFIED.);
#1269=B_SPLINE_CURVE_WITH_KNOTS('',3,(#10674,#10675,#10676,#10677,#10678,
#10679,#10680,#10681,#10682,#10683,#10684),.UNSPECIFIED.,.F.,.F.,(4,1,1,
1,1,1,1,1,4),(28.2743338823081,28.3645495163253,29.3621501237216,30.3597507311179,
31.3573513385142,32.3549519459105,33.3525525533068,34.3501531607031,34.5575191894877),
 .UNSPECIFIED.);
#1270=B_SPLINE_CURVE_WITH_KNOTS('',3,(#10689,#10690,#10691,#10692,#10693,
#10694,#10695,#10696,#10697,#10698),.UNSPECIFIED.,.F.,.F.,(4,1,1,1,1,1,
1,4),(21.9911485751285,22.8351866856161,23.8327872930124,24.8303879004087,
25.827988507805,26.8255891152013,27.8231897225976,28.2743338823081),
 .UNSPECIFIED.);
#1271=B_SPLINE_CURVE_WITH_KNOTS('',3,(#10699,#10700,#10701,#10702,#10703,
#10704,#10705,#10706,#10707,#10708),.UNSPECIFIED.,.F.,.F.,(4,1,1,1,1,1,
1,4),(21.9911485751285,22.3789458719474,23.3765464793437,24.37414708674,
25.3717476941363,26.3693483015326,27.366948908929,28.2743338823081),
 .UNSPECIFIED.);
#1272=B_SPLINE_CURVE_WITH_KNOTS('',3,(#10714,#10715,#10716,#10717,#10718),
 .UNSPECIFIED.,.F.,.F.,(4,1,4),(14.3981410127769,15.3957416201732,15.7079632679489),
 .UNSPECIFIED.);
#1273=B_SPLINE_CURVE_WITH_KNOTS('',3,(#10721,#10722,#10723,#10724,#10725),
 .UNSPECIFIED.,.F.,.F.,(4,1,4),(13.8761928695311,14.8543818264456,15.7079632679489),
 .UNSPECIFIED.);
#1274=B_SPLINE_CURVE_WITH_KNOTS('',3,(#10731,#10732,#10733,#10734),
 .UNSPECIFIED.,.F.,.F.,(4,4),(84.8230016469244,85.6840249515836),
 .UNSPECIFIED.);
#1275=B_SPLINE_CURVE_WITH_KNOTS('',3,(#10737,#10738,#10739,#10740,#10741),
 .UNSPECIFIED.,.F.,.F.,(4,1,4),(84.8230016469244,85.2277841379149,86.2059730948294),
 .UNSPECIFIED.);
#1276=B_SPLINE_CURVE_WITH_KNOTS('',3,(#10746,#10747,#10748,#10749,#10750,
#10751,#10752,#10753,#10754,#10755,#10756),.UNSPECIFIED.,.F.,.F.,(4,1,1,
1,1,1,1,1,4),(78.5398163397448,78.7008206998094,79.6984213072057,80.696021914602,
81.6936225219983,82.6912231293946,83.6888237367909,84.6864243441872,84.8230016469244),
 .UNSPECIFIED.);
#1277=B_SPLINE_CURVE_WITH_KNOTS('',3,(#10757,#10758,#10759,#10760,#10761,
#10762,#10763,#10764,#10765,#10766),.UNSPECIFIED.,.F.,.F.,(4,1,1,1,1,1,
1,4),(78.5398163397448,79.242180493537,80.2397811009333,81.2373817083296,
82.2349823157259,83.2325829231222,84.2301835305186,84.8230016469244),
 .UNSPECIFIED.);
#1278=B_SPLINE_CURVE_WITH_KNOTS('',3,(#10771,#10772,#10773,#10774,#10775,
#10776,#10777,#10778,#10779,#10780),.UNSPECIFIED.,.F.,.F.,(4,1,1,1,1,1,
1,4),(72.2566310325652,72.7152170554315,73.7128176628278,74.7104182702242,
75.7080188776205,76.7056194850168,77.7032200924131,78.5398163397448),
 .UNSPECIFIED.);
#1279=B_SPLINE_CURVE_WITH_KNOTS('',3,(#10781,#10782,#10783,#10784,#10785,
#10786,#10787,#10788,#10789,#10790,#10791),.UNSPECIFIED.,.F.,.F.,(4,1,1,
1,1,1,1,1,4),(72.2566310325652,72.2589762417629,73.2565768491592,74.2541774565555,
75.2517780639518,76.2493786713481,77.2469792787444,78.2445798861407,78.5398163397448),
 .UNSPECIFIED.);
#1280=B_SPLINE_CURVE_WITH_KNOTS('',3,(#10796,#10797,#10798,#10799,#10800,
#10801,#10802,#10803,#10804,#10805),.UNSPECIFIED.,.F.,.F.,(4,1,1,1,1,1,
1,4),(65.9734457253856,66.7296134110537,67.72721401845,68.7248146258463,
69.7224152332426,70.7200158406389,71.7176164480352,72.2566310325652),
 .UNSPECIFIED.);
#1281=B_SPLINE_CURVE_WITH_KNOTS('',3,(#10806,#10807,#10808,#10809,#10810,
#10811,#10812,#10813,#10814,#10815),.UNSPECIFIED.,.F.,.F.,(4,1,1,1,1,1,
1,4),(65.9734457253856,66.273372597385,67.2709732047813,68.2685738121776,
69.2661744195739,70.2637750269702,71.2613756343665,72.2566310325652),
 .UNSPECIFIED.);
#1282=B_SPLINE_CURVE_WITH_KNOTS('',3,(#10820,#10821,#10822,#10823,#10824,
#10825,#10826,#10827,#10828,#10829,#10830),.UNSPECIFIED.,.F.,.F.,(4,1,1,
1,1,1,1,1,4),(59.690260418206,59.7464091592795,60.7440097666758,61.7416103740721,
62.7392109814684,63.7368115888648,64.7344121962611,65.7320128036574,65.9734457253856),
 .UNSPECIFIED.);
#1283=B_SPLINE_CURVE_WITH_KNOTS('',3,(#10831,#10832,#10833,#10834,#10835,
#10836,#10837,#10838,#10839,#10840),.UNSPECIFIED.,.F.,.F.,(4,1,1,1,1,1,
1,4),(59.6902604182061,60.2877689530071,61.2853695604035,62.2829701677998,
63.2805707751961,64.2781713825924,65.2757719899887,65.9734457253856),
 .UNSPECIFIED.);
#1284=B_SPLINE_CURVE_WITH_KNOTS('',3,(#10845,#10846,#10847,#10848,#10849,
#10850,#10851,#10852,#10853,#10854),.UNSPECIFIED.,.F.,.F.,(4,1,1,1,1,1,
1,4),(53.4070751110265,53.7608055149017,54.758406122298,55.7560067296943,
56.7536073370906,57.7512079444869,58.7488085518832,59.690260418206),
 .UNSPECIFIED.);
#1285=B_SPLINE_CURVE_WITH_KNOTS('',3,(#10855,#10856,#10857,#10858,#10859,
#10860,#10861,#10862,#10863,#10864),.UNSPECIFIED.,.F.,.F.,(4,1,1,1,1,1,
1,4),(53.4070751110265,54.3021653086293,55.2997659160256,56.2973665234219,
57.2949671308182,58.2925677382145,59.2901683456108,59.6902604182061),
 .UNSPECIFIED.);
#1286=B_SPLINE_CURVE_WITH_KNOTS('',3,(#10869,#10870,#10871,#10872,#10873,
#10874,#10875,#10876,#10877,#10878),.UNSPECIFIED.,.F.,.F.,(4,1,1,1,1,1,
1,4),(47.1238898038469,47.7752018705238,48.7728024779201,49.7704030853164,
50.7680036927127,51.765604300109,52.7632049075054,53.4070751110265),
 .UNSPECIFIED.);
#1287=B_SPLINE_CURVE_WITH_KNOTS('',3,(#10879,#10880,#10881,#10882,#10883,
#10884,#10885,#10886,#10887,#10888,#10889),.UNSPECIFIED.,.F.,.F.,(4,1,1,
1,1,1,1,1,4),(47.1238898038469,47.3189610568551,48.3165616642514,49.3141622716477,
50.3117628790441,51.3093634864404,52.3069640938367,53.304564701233,53.4070751110265),
 .UNSPECIFIED.);
#1288=B_SPLINE_CURVE_WITH_KNOTS('',3,(#10894,#10895,#10896,#10897,#10898,
#10899,#10900,#10901,#10902,#10903),.UNSPECIFIED.,.F.,.F.,(4,1,1,1,1,1,
1,4),(40.8407044966673,41.7895982261459,42.7871988335423,43.7847994409386,
44.7824000483349,45.7800006557312,46.7776012631275,47.1238898038469),
 .UNSPECIFIED.);
#1289=B_SPLINE_CURVE_WITH_KNOTS('',3,(#10904,#10905,#10906,#10907,#10908,
#10909,#10910,#10911,#10912,#10913),.UNSPECIFIED.,.F.,.F.,(4,1,1,1,1,1,
1,4),(40.8407044966673,41.3333574124773,42.3309580198736,43.3285586272699,
44.3261592346662,45.3237598420625,46.3213604494588,47.1238898038469),
 .UNSPECIFIED.);
#1290=B_SPLINE_CURVE_WITH_KNOTS('',3,(#10918,#10919,#10920,#10921,#10922,
#10923,#10924,#10925,#10926,#10927,#10928),.UNSPECIFIED.,.F.,.F.,(4,1,1,
1,1,1,1,1,4),(34.5575191894877,34.8063939743718,35.8039945817681,36.8015951891644,
37.7991957965607,38.796796403957,39.7943970113533,40.7919976187496,40.8407044966673),
 .UNSPECIFIED.);
#1291=B_SPLINE_CURVE_WITH_KNOTS('',3,(#10929,#10930,#10931,#10932,#10933,
#10934,#10935,#10936,#10937,#10938),.UNSPECIFIED.,.F.,.F.,(4,1,1,1,1,1,
1,4),(34.5575191894877,35.3477537680994,36.3453543754957,37.342954982892,
38.3405555902883,39.3381561976846,40.335756805081,40.8407044966673),
 .UNSPECIFIED.);
#1292=B_SPLINE_CURVE_WITH_KNOTS('',3,(#10943,#10944,#10945,#10946,#10947,
#10948,#10949,#10950,#10951,#10952),.UNSPECIFIED.,.F.,.F.,(4,1,1,1,1,1,
1,4),(28.2743338823081,28.8207903299939,29.8183909373902,30.8159915447865,
31.8135921521829,32.8111927595792,33.8087933669755,34.5575191894877),
 .UNSPECIFIED.);
#1293=B_SPLINE_CURVE_WITH_KNOTS('',3,(#10953,#10954,#10955,#10956,#10957,
#10958,#10959,#10960,#10961,#10962,#10963),.UNSPECIFIED.,.F.,.F.,(4,1,1,
1,1,1,1,1,4),(28.2743338823081,28.3645495163252,29.3621501237216,30.3597507311179,
31.3573513385142,32.3549519459105,33.3525525533068,34.3501531607031,34.5575191894877),
 .UNSPECIFIED.);
#1294=B_SPLINE_CURVE_WITH_KNOTS('',3,(#10968,#10969,#10970,#10971,#10972,
#10973,#10974,#10975,#10976,#10977),.UNSPECIFIED.,.F.,.F.,(4,1,1,1,1,1,
1,4),(21.9911485751285,22.8351866856161,23.8327872930124,24.8303879004087,
25.827988507805,26.8255891152013,27.8231897225976,28.2743338823081),
 .UNSPECIFIED.);
#1295=B_SPLINE_CURVE_WITH_KNOTS('',3,(#10978,#10979,#10980,#10981,#10982,
#10983,#10984,#10985,#10986,#10987),.UNSPECIFIED.,.F.,.F.,(4,1,1,1,1,1,
1,4),(21.9911485751285,22.3789458719474,23.3765464793437,24.37414708674,
25.3717476941363,26.3693483015326,27.3669489089289,28.2743338823081),
 .UNSPECIFIED.);
#1296=B_SPLINE_CURVE_WITH_KNOTS('',3,(#10993,#10994,#10995,#10996,#10997),
 .UNSPECIFIED.,.F.,.F.,(4,1,4),(14.3981410127769,15.3957416201732,15.7079632679489),
 .UNSPECIFIED.);
#1297=B_SPLINE_CURVE_WITH_KNOTS('',3,(#11000,#11001,#11002,#11003,#11004),
 .UNSPECIFIED.,.F.,.F.,(4,1,4),(13.8761928695311,14.8543818264456,15.7079632679489),
 .UNSPECIFIED.);
#1298=B_SPLINE_CURVE_WITH_KNOTS('',3,(#11010,#11011,#11012,#11013),
 .UNSPECIFIED.,.F.,.F.,(4,4),(84.8230016469244,85.6840249515836),
 .UNSPECIFIED.);
#1299=B_SPLINE_CURVE_WITH_KNOTS('',3,(#11016,#11017,#11018,#11019,#11020),
 .UNSPECIFIED.,.F.,.F.,(4,1,4),(84.8230016469244,85.2277841379149,86.2059730948294),
 .UNSPECIFIED.);
#1300=B_SPLINE_CURVE_WITH_KNOTS('',3,(#11025,#11026,#11027,#11028,#11029,
#11030,#11031,#11032,#11033,#11034,#11035),.UNSPECIFIED.,.F.,.F.,(4,1,1,
1,1,1,1,1,4),(78.5398163397448,78.7008206998094,79.6984213072057,80.696021914602,
81.6936225219983,82.6912231293946,83.6888237367909,84.6864243441872,84.8230016469244),
 .UNSPECIFIED.);
#1301=B_SPLINE_CURVE_WITH_KNOTS('',3,(#11036,#11037,#11038,#11039,#11040,
#11041,#11042,#11043,#11044,#11045),.UNSPECIFIED.,.F.,.F.,(4,1,1,1,1,1,
1,4),(78.5398163397448,79.242180493537,80.2397811009333,81.2373817083296,
82.2349823157259,83.2325829231222,84.2301835305186,84.8230016469244),
 .UNSPECIFIED.);
#1302=B_SPLINE_CURVE_WITH_KNOTS('',3,(#11050,#11051,#11052,#11053,#11054,
#11055,#11056,#11057,#11058,#11059),.UNSPECIFIED.,.F.,.F.,(4,1,1,1,1,1,
1,4),(72.2566310325652,72.7152170554315,73.7128176628278,74.7104182702242,
75.7080188776205,76.7056194850168,77.7032200924131,78.5398163397448),
 .UNSPECIFIED.);
#1303=B_SPLINE_CURVE_WITH_KNOTS('',3,(#11060,#11061,#11062,#11063,#11064,
#11065,#11066,#11067,#11068,#11069,#11070),.UNSPECIFIED.,.F.,.F.,(4,1,1,
1,1,1,1,1,4),(72.2566310325652,72.2589762417629,73.2565768491592,74.2541774565555,
75.2517780639518,76.2493786713481,77.2469792787444,78.2445798861407,78.5398163397448),
 .UNSPECIFIED.);
#1304=B_SPLINE_CURVE_WITH_KNOTS('',3,(#11075,#11076,#11077,#11078,#11079,
#11080,#11081,#11082,#11083,#11084),.UNSPECIFIED.,.F.,.F.,(4,1,1,1,1,1,
1,4),(65.9734457253856,66.7296134110537,67.72721401845,68.7248146258463,
69.7224152332426,70.7200158406389,71.7176164480352,72.2566310325652),
 .UNSPECIFIED.);
#1305=B_SPLINE_CURVE_WITH_KNOTS('',3,(#11085,#11086,#11087,#11088,#11089,
#11090,#11091,#11092,#11093,#11094),.UNSPECIFIED.,.F.,.F.,(4,1,1,1,1,1,
1,4),(65.9734457253856,66.273372597385,67.2709732047813,68.2685738121776,
69.2661744195739,70.2637750269702,71.2613756343665,72.2566310325652),
 .UNSPECIFIED.);
#1306=B_SPLINE_CURVE_WITH_KNOTS('',3,(#11099,#11100,#11101,#11102,#11103,
#11104,#11105,#11106,#11107,#11108,#11109),.UNSPECIFIED.,.F.,.F.,(4,1,1,
1,1,1,1,1,4),(59.690260418206,59.7464091592795,60.7440097666758,61.7416103740721,
62.7392109814684,63.7368115888648,64.7344121962611,65.7320128036574,65.9734457253856),
 .UNSPECIFIED.);
#1307=B_SPLINE_CURVE_WITH_KNOTS('',3,(#11110,#11111,#11112,#11113,#11114,
#11115,#11116,#11117,#11118,#11119),.UNSPECIFIED.,.F.,.F.,(4,1,1,1,1,1,
1,4),(59.690260418206,60.2877689530071,61.2853695604035,62.2829701677998,
63.2805707751961,64.2781713825924,65.2757719899887,65.9734457253856),
 .UNSPECIFIED.);
#1308=B_SPLINE_CURVE_WITH_KNOTS('',3,(#11124,#11125,#11126,#11127,#11128,
#11129,#11130,#11131,#11132,#11133),.UNSPECIFIED.,.F.,.F.,(4,1,1,1,1,1,
1,4),(53.4070751110265,53.7608055149017,54.758406122298,55.7560067296943,
56.7536073370906,57.7512079444869,58.7488085518832,59.690260418206),
 .UNSPECIFIED.);
#1309=B_SPLINE_CURVE_WITH_KNOTS('',3,(#11134,#11135,#11136,#11137,#11138,
#11139,#11140,#11141,#11142,#11143),.UNSPECIFIED.,.F.,.F.,(4,1,1,1,1,1,
1,4),(53.4070751110265,54.3021653086293,55.2997659160256,56.2973665234219,
57.2949671308182,58.2925677382145,59.2901683456108,59.690260418206),
 .UNSPECIFIED.);
#1310=B_SPLINE_CURVE_WITH_KNOTS('',3,(#11148,#11149,#11150,#11151,#11152,
#11153,#11154,#11155,#11156,#11157),.UNSPECIFIED.,.F.,.F.,(4,1,1,1,1,1,
1,4),(47.1238898038469,47.7752018705238,48.7728024779201,49.7704030853164,
50.7680036927127,51.765604300109,52.7632049075054,53.4070751110265),
 .UNSPECIFIED.);
#1311=B_SPLINE_CURVE_WITH_KNOTS('',3,(#11158,#11159,#11160,#11161,#11162,
#11163,#11164,#11165,#11166,#11167,#11168),.UNSPECIFIED.,.F.,.F.,(4,1,1,
1,1,1,1,1,4),(47.1238898038469,47.3189610568551,48.3165616642514,49.3141622716477,
50.3117628790441,51.3093634864404,52.3069640938367,53.304564701233,53.4070751110265),
 .UNSPECIFIED.);
#1312=B_SPLINE_CURVE_WITH_KNOTS('',3,(#11173,#11174,#11175,#11176,#11177,
#11178,#11179,#11180,#11181,#11182),.UNSPECIFIED.,.F.,.F.,(4,1,1,1,1,1,
1,4),(40.8407044966673,41.7895982261459,42.7871988335423,43.7847994409386,
44.7824000483349,45.7800006557312,46.7776012631275,47.1238898038469),
 .UNSPECIFIED.);
#1313=B_SPLINE_CURVE_WITH_KNOTS('',3,(#11183,#11184,#11185,#11186,#11187,
#11188,#11189,#11190,#11191,#11192),.UNSPECIFIED.,.F.,.F.,(4,1,1,1,1,1,
1,4),(40.8407044966673,41.3333574124773,42.3309580198736,43.3285586272699,
44.3261592346662,45.3237598420625,46.3213604494588,47.1238898038469),
 .UNSPECIFIED.);
#1314=B_SPLINE_CURVE_WITH_KNOTS('',3,(#11197,#11198,#11199,#11200,#11201,
#11202,#11203,#11204,#11205,#11206,#11207),.UNSPECIFIED.,.F.,.F.,(4,1,1,
1,1,1,1,1,4),(34.5575191894877,34.8063939743718,35.8039945817681,36.8015951891644,
37.7991957965607,38.796796403957,39.7943970113533,40.7919976187496,40.8407044966673),
 .UNSPECIFIED.);
#1315=B_SPLINE_CURVE_WITH_KNOTS('',3,(#11208,#11209,#11210,#11211,#11212,
#11213,#11214,#11215,#11216,#11217),.UNSPECIFIED.,.F.,.F.,(4,1,1,1,1,1,
1,4),(34.5575191894877,35.3477537680994,36.3453543754957,37.342954982892,
38.3405555902883,39.3381561976846,40.335756805081,40.8407044966673),
 .UNSPECIFIED.);
#1316=B_SPLINE_CURVE_WITH_KNOTS('',3,(#11222,#11223,#11224,#11225,#11226,
#11227,#11228,#11229,#11230,#11231),.UNSPECIFIED.,.F.,.F.,(4,1,1,1,1,1,
1,4),(28.2743338823081,28.8207903299939,29.8183909373902,30.8159915447865,
31.8135921521829,32.8111927595792,33.8087933669755,34.5575191894877),
 .UNSPECIFIED.);
#1317=B_SPLINE_CURVE_WITH_KNOTS('',3,(#11232,#11233,#11234,#11235,#11236,
#11237,#11238,#11239,#11240,#11241,#11242),.UNSPECIFIED.,.F.,.F.,(4,1,1,
1,1,1,1,1,4),(28.2743338823081,28.3645495163252,29.3621501237216,30.3597507311179,
31.3573513385142,32.3549519459105,33.3525525533068,34.3501531607031,34.5575191894877),
 .UNSPECIFIED.);
#1318=B_SPLINE_CURVE_WITH_KNOTS('',3,(#11247,#11248,#11249,#11250,#11251,
#11252,#11253,#11254,#11255,#11256),.UNSPECIFIED.,.F.,.F.,(4,1,1,1,1,1,
1,4),(21.9911485751285,22.8351866856161,23.8327872930124,24.8303879004087,
25.827988507805,26.8255891152013,27.8231897225976,28.2743338823081),
 .UNSPECIFIED.);
#1319=B_SPLINE_CURVE_WITH_KNOTS('',3,(#11257,#11258,#11259,#11260,#11261,
#11262,#11263,#11264,#11265,#11266),.UNSPECIFIED.,.F.,.F.,(4,1,1,1,1,1,
1,4),(21.9911485751285,22.3789458719474,23.3765464793437,24.37414708674,
25.3717476941363,26.3693483015326,27.3669489089289,28.2743338823081),
 .UNSPECIFIED.);
#1320=B_SPLINE_CURVE_WITH_KNOTS('',3,(#11272,#11273,#11274,#11275,#11276),
 .UNSPECIFIED.,.F.,.F.,(4,1,4),(14.3981410127769,15.3957416201732,15.7079632679489),
 .UNSPECIFIED.);
#1321=B_SPLINE_CURVE_WITH_KNOTS('',3,(#11279,#11280,#11281,#11282,#11283),
 .UNSPECIFIED.,.F.,.F.,(4,1,4),(13.8761928695311,14.8543818264456,15.7079632679489),
 .UNSPECIFIED.);
#1322=B_SPLINE_CURVE_WITH_KNOTS('',3,(#11289,#11290,#11291,#11292),
 .UNSPECIFIED.,.F.,.F.,(4,4),(84.8230016469244,85.6840249515836),
 .UNSPECIFIED.);
#1323=B_SPLINE_CURVE_WITH_KNOTS('',3,(#11295,#11296,#11297,#11298,#11299),
 .UNSPECIFIED.,.F.,.F.,(4,1,4),(84.8230016469244,85.2277841379149,86.2059730948294),
 .UNSPECIFIED.);
#1324=B_SPLINE_CURVE_WITH_KNOTS('',3,(#11304,#11305,#11306,#11307,#11308,
#11309,#11310,#11311,#11312,#11313,#11314),.UNSPECIFIED.,.F.,.F.,(4,1,1,
1,1,1,1,1,4),(78.5398163397448,78.7008206998094,79.6984213072057,80.696021914602,
81.6936225219983,82.6912231293946,83.688823736791,84.6864243441873,84.8230016469244),
 .UNSPECIFIED.);
#1325=B_SPLINE_CURVE_WITH_KNOTS('',3,(#11315,#11316,#11317,#11318,#11319,
#11320,#11321,#11322,#11323,#11324),.UNSPECIFIED.,.F.,.F.,(4,1,1,1,1,1,
1,4),(78.5398163397448,79.242180493537,80.2397811009333,81.2373817083296,
82.2349823157259,83.2325829231223,84.2301835305186,84.8230016469244),
 .UNSPECIFIED.);
#1326=B_SPLINE_CURVE_WITH_KNOTS('',3,(#11329,#11330,#11331,#11332,#11333,
#11334,#11335,#11336,#11337,#11338),.UNSPECIFIED.,.F.,.F.,(4,1,1,1,1,1,
1,4),(72.2566310325652,72.7152170554316,73.7128176628279,74.7104182702242,
75.7080188776205,76.7056194850168,77.7032200924131,78.5398163397448),
 .UNSPECIFIED.);
#1327=B_SPLINE_CURVE_WITH_KNOTS('',3,(#11339,#11340,#11341,#11342,#11343,
#11344,#11345,#11346,#11347,#11348,#11349),.UNSPECIFIED.,.F.,.F.,(4,1,1,
1,1,1,1,1,4),(72.2566310325652,72.2589762417629,73.2565768491592,74.2541774565555,
75.2517780639518,76.2493786713481,77.2469792787444,78.2445798861407,78.5398163397448),
 .UNSPECIFIED.);
#1328=B_SPLINE_CURVE_WITH_KNOTS('',3,(#11354,#11355,#11356,#11357,#11358,
#11359,#11360,#11361,#11362,#11363),.UNSPECIFIED.,.F.,.F.,(4,1,1,1,1,1,
1,4),(65.9734457253856,66.7296134110537,67.72721401845,68.7248146258463,
69.7224152332426,70.7200158406389,71.7176164480352,72.2566310325652),
 .UNSPECIFIED.);
#1329=B_SPLINE_CURVE_WITH_KNOTS('',3,(#11364,#11365,#11366,#11367,#11368,
#11369,#11370,#11371,#11372,#11373),.UNSPECIFIED.,.F.,.F.,(4,1,1,1,1,1,
1,4),(65.9734457253856,66.273372597385,67.2709732047813,68.2685738121776,
69.2661744195739,70.2637750269702,71.2613756343666,72.2566310325652),
 .UNSPECIFIED.);
#1330=B_SPLINE_CURVE_WITH_KNOTS('',3,(#11378,#11379,#11380,#11381,#11382,
#11383,#11384,#11385,#11386,#11387,#11388),.UNSPECIFIED.,.F.,.F.,(4,1,1,
1,1,1,1,1,4),(59.690260418206,59.7464091592795,60.7440097666758,61.7416103740722,
62.7392109814685,63.7368115888648,64.7344121962611,65.7320128036574,65.9734457253856),
 .UNSPECIFIED.);
#1331=B_SPLINE_CURVE_WITH_KNOTS('',3,(#11389,#11390,#11391,#11392,#11393,
#11394,#11395,#11396,#11397,#11398),.UNSPECIFIED.,.F.,.F.,(4,1,1,1,1,1,
1,4),(59.690260418206,60.2877689530072,61.2853695604035,62.2829701677998,
63.2805707751961,64.2781713825924,65.2757719899887,65.9734457253856),
 .UNSPECIFIED.);
#1332=B_SPLINE_CURVE_WITH_KNOTS('',3,(#11403,#11404,#11405,#11406,#11407,
#11408,#11409,#11410,#11411,#11412),.UNSPECIFIED.,.F.,.F.,(4,1,1,1,1,1,
1,4),(53.4070751110265,53.7608055149017,54.758406122298,55.7560067296943,
56.7536073370906,57.7512079444869,58.7488085518832,59.690260418206),
 .UNSPECIFIED.);
#1333=B_SPLINE_CURVE_WITH_KNOTS('',3,(#11413,#11414,#11415,#11416,#11417,
#11418,#11419,#11420,#11421,#11422),.UNSPECIFIED.,.F.,.F.,(4,1,1,1,1,1,
1,4),(53.4070751110265,54.3021653086293,55.2997659160256,56.2973665234219,
57.2949671308182,58.2925677382145,59.2901683456108,59.690260418206),
 .UNSPECIFIED.);
#1334=B_SPLINE_CURVE_WITH_KNOTS('',3,(#11427,#11428,#11429,#11430,#11431,
#11432,#11433,#11434,#11435,#11436),.UNSPECIFIED.,.F.,.F.,(4,1,1,1,1,1,
1,4),(47.1238898038469,47.7752018705238,48.7728024779201,49.7704030853164,
50.7680036927128,51.7656043001091,52.7632049075054,53.4070751110265),
 .UNSPECIFIED.);
#1335=B_SPLINE_CURVE_WITH_KNOTS('',3,(#11437,#11438,#11439,#11440,#11441,
#11442,#11443,#11444,#11445,#11446,#11447),.UNSPECIFIED.,.F.,.F.,(4,1,1,
1,1,1,1,1,4),(47.1238898038469,47.3189610568551,48.3165616642514,49.3141622716478,
50.3117628790441,51.3093634864404,52.3069640938367,53.304564701233,53.4070751110265),
 .UNSPECIFIED.);
#1336=B_SPLINE_CURVE_WITH_KNOTS('',3,(#11452,#11453,#11454,#11455,#11456,
#11457,#11458,#11459,#11460,#11461),.UNSPECIFIED.,.F.,.F.,(4,1,1,1,1,1,
1,4),(40.8407044966673,41.789598226146,42.7871988335423,43.7847994409386,
44.7824000483349,45.7800006557312,46.7776012631275,47.1238898038469),
 .UNSPECIFIED.);
#1337=B_SPLINE_CURVE_WITH_KNOTS('',3,(#11462,#11463,#11464,#11465,#11466,
#11467,#11468,#11469,#11470,#11471),.UNSPECIFIED.,.F.,.F.,(4,1,1,1,1,1,
1,4),(40.8407044966673,41.3333574124773,42.3309580198736,43.3285586272699,
44.3261592346662,45.3237598420625,46.3213604494588,47.1238898038469),
 .UNSPECIFIED.);
#1338=B_SPLINE_CURVE_WITH_KNOTS('',3,(#11476,#11477,#11478,#11479,#11480,
#11481,#11482,#11483,#11484,#11485,#11486),.UNSPECIFIED.,.F.,.F.,(4,1,1,
1,1,1,1,1,4),(34.5575191894877,34.8063939743718,35.8039945817681,36.8015951891644,
37.7991957965607,38.796796403957,39.7943970113533,40.7919976187497,40.8407044966673),
 .UNSPECIFIED.);
#1339=B_SPLINE_CURVE_WITH_KNOTS('',3,(#11487,#11488,#11489,#11490,#11491,
#11492,#11493,#11494,#11495,#11496),.UNSPECIFIED.,.F.,.F.,(4,1,1,1,1,1,
1,4),(34.5575191894877,35.3477537680994,36.3453543754957,37.342954982892,
38.3405555902884,39.3381561976847,40.335756805081,40.8407044966673),
 .UNSPECIFIED.);
#1340=B_SPLINE_CURVE_WITH_KNOTS('',3,(#11501,#11502,#11503,#11504,#11505,
#11506,#11507,#11508,#11509,#11510),.UNSPECIFIED.,.F.,.F.,(4,1,1,1,1,1,
1,4),(28.2743338823081,28.8207903299939,29.8183909373903,30.8159915447866,
31.8135921521829,32.8111927595792,33.8087933669755,34.5575191894877),
 .UNSPECIFIED.);
#1341=B_SPLINE_CURVE_WITH_KNOTS('',3,(#11511,#11512,#11513,#11514,#11515,
#11516,#11517,#11518,#11519,#11520,#11521),.UNSPECIFIED.,.F.,.F.,(4,1,1,
1,1,1,1,1,4),(28.2743338823081,28.3645495163253,29.3621501237216,30.3597507311179,
31.3573513385142,32.3549519459105,33.3525525533068,34.3501531607031,34.5575191894877),
 .UNSPECIFIED.);
#1342=B_SPLINE_CURVE_WITH_KNOTS('',3,(#11526,#11527,#11528,#11529,#11530,
#11531,#11532,#11533,#11534,#11535),.UNSPECIFIED.,.F.,.F.,(4,1,1,1,1,1,
1,4),(21.9911485751285,22.8351866856161,23.8327872930124,24.8303879004087,
25.827988507805,26.8255891152013,27.8231897225976,28.2743338823081),
 .UNSPECIFIED.);
#1343=B_SPLINE_CURVE_WITH_KNOTS('',3,(#11536,#11537,#11538,#11539,#11540,
#11541,#11542,#11543,#11544,#11545),.UNSPECIFIED.,.F.,.F.,(4,1,1,1,1,1,
1,4),(21.9911485751285,22.3789458719474,23.3765464793437,24.37414708674,
25.3717476941363,26.3693483015326,27.366948908929,28.2743338823081),
 .UNSPECIFIED.);
#1344=B_SPLINE_CURVE_WITH_KNOTS('',3,(#11551,#11552,#11553,#11554,#11555),
 .UNSPECIFIED.,.F.,.F.,(4,1,4),(14.3981410127769,15.3957416201732,15.7079632679489),
 .UNSPECIFIED.);
#1345=B_SPLINE_CURVE_WITH_KNOTS('',3,(#11558,#11559,#11560,#11561,#11562),
 .UNSPECIFIED.,.F.,.F.,(4,1,4),(13.8761928695311,14.8543818264456,15.7079632679489),
 .UNSPECIFIED.);
#1346=B_SPLINE_CURVE_WITH_KNOTS('',3,(#11639,#11640,#11641,#11642,#11643,
#11644,#11645,#11646,#11647,#11648),.UNSPECIFIED.,.F.,.F.,(4,2,2,2,4),(-0.768826429832705,
-0.767240199593363,-0.57329716583777,-0.461315679430967,-0.383620099794532),
 .UNSPECIFIED.);
#1347=B_SPLINE_CURVE_WITH_KNOTS('',3,(#11649,#11650,#11651,#11652,#11653,
#11654,#11655,#11656,#11657,#11658),.UNSPECIFIED.,.F.,.F.,(4,2,2,2,4),(-0.383620099794532,
-0.305924520158085,-0.193943033751236,0.,0.00158623023937601),
 .UNSPECIFIED.);
#1348=B_SPLINE_CURVE_WITH_KNOTS('',3,(#11669,#11670,#11671,#11672,#11673,
#11674,#11675,#11676,#11677,#11678,#11679,#11680,#11681,#11682,#11683,#11684,
#11685,#11686),.UNSPECIFIED.,.F.,.F.,(4,2,2,2,2,2,2,2,4),(-0.76882642980026,
-0.76724019956098,-0.573297165814677,-0.461315679413209,-0.383620099780493,
-0.305924520147777,-0.193943033746308,0.,0.00158623023927986),
 .UNSPECIFIED.);
#1349=B_SPLINE_CURVE_WITH_KNOTS('',3,(#11723,#11724,#11725,#11726,#11727,
#11728,#11729,#11730,#11731,#11732,#11733),.UNSPECIFIED.,.F.,.F.,(4,1,1,
1,1,1,1,1,4),(15.7079632679489,15.8519824338419,16.8495830412382,17.8471836486345,
18.8447842560309,19.8423848634272,20.8399854708235,21.8375860782198,21.9911485751285),
 .UNSPECIFIED.);
#1350=B_SPLINE_CURVE_WITH_KNOTS('',3,(#11734,#11735,#11736,#11737,#11738,
#11739,#11740,#11741,#11742,#11743),.UNSPECIFIED.,.F.,.F.,(4,1,1,1,1,1,
1,4),(15.7079632679489,16.3933422275696,17.3909428349659,18.3885434423622,
19.3861440497585,20.3837446571548,21.3813452645511,21.9911485751285),
 .UNSPECIFIED.);
#1351=B_SPLINE_CURVE_WITH_KNOTS('',3,(#12052,#12053,#12054,#12055,#12056,
#12057,#12058,#12059,#12060,#12061,#12062,#12063,#12064,#12065,#12066,#12067,
#12068,#12069,#12070,#12071,#12072,#12073,#12074,#12075,#12076,#12077,#12078,
#12079,#12080,#12081,#12082,#12083,#12084,#12085,#12086,#12087,#12088,#12089,
#12090,#12091,#12092,#12093,#12094,#12095,#12096,#12097,#12098,#12099,#12100,
#12101,#12102,#12103,#12104,#12105,#12106,#12107,#12108,#12109,#12110,#12111,
#12112,#12113,#12114,#12115,#12116,#12117,#12118,#12119,#12120,#12121,#12122,
#12123,#12124,#12125,#12126,#12127,#12128,#12129,#12130,#12131,#12132,#12133,
#12134,#12135,#12136),.UNSPECIFIED.,.F.,.F.,(4,3,3,3,3,3,3,3,3,3,3,3,3,
3,3,3,3,3,3,3,3,3,3,3,3,3,3,3,4),(0.,0.0219686281715528,0.0445463606193457,
0.0636242036118209,0.07209744784919,0.0767548581315063,0.0810487310113372,
0.102995303995266,0.124770867091271,0.14287042645824,0.150424219747402,
0.153922407205223,0.157567539717946,0.178337434372214,0.197169104559147,
0.219441601244649,0.224346217653563,0.229396798853662,0.250061927167916,
0.270722751313313,0.28567879435863,0.29689604993752,0.300623771856885,0.320395161135708,
0.334310894762281,0.33877647602486,0.357799721593331,0.375349078043162,
0.378621596831385),.UNSPECIFIED.);
#1352=B_SPLINE_CURVE_WITH_KNOTS('',3,(#12137,#12138,#12139,#12140,#12141,
#12142,#12143,#12144,#12145,#12146,#12147,#12148,#12149,#12150,#12151,#12152,
#12153,#12154,#12155,#12156,#12157,#12158,#12159,#12160,#12161,#12162,#12163,
#12164,#12165,#12166,#12167,#12168,#12169,#12170,#12171,#12172,#12173,#12174,
#12175,#12176,#12177,#12178,#12179,#12180,#12181,#12182,#12183,#12184,#12185,
#12186,#12187,#12188,#12189,#12190,#12191,#12192,#12193,#12194),
 .UNSPECIFIED.,.F.,.F.,(4,3,3,3,3,3,3,3,3,3,3,3,3,3,3,3,3,3,3,4),(-0.254990279232818,
-0.234477349668193,-0.22871674086773,-0.22506482824537,-0.203760387757535,
-0.200823997383662,-0.180338507409432,-0.158296763353209,-0.154234245100677,
-0.150791656345001,-0.129409593000311,-0.107575878454977,-0.0856092981050521,
-0.0801787505710101,-0.0759363781823176,-0.0533889982303693,-0.0308167874784648,
-0.00875888267892488,-0.00400455495965136,0.),.UNSPECIFIED.);
#1353=B_SPLINE_CURVE_WITH_KNOTS('',3,(#12195,#12196,#12197,#12198,#12199,
#12200,#12201,#12202,#12203,#12204,#12205,#12206,#12207,#12208,#12209,#12210,
#12211,#12212,#12213,#12214,#12215,#12216,#12217,#12218,#12219,#12220,#12221,
#12222),.UNSPECIFIED.,.F.,.F.,(4,3,3,3,3,3,3,3,3,4),(0.,0.0187208397268737,
0.0379355165382035,0.0581727843953796,0.0646638548438618,0.068387447778056,
0.0884839760262796,0.108890832871008,0.118884587966908,0.123178515106518),
 .UNSPECIFIED.);
#1354=B_SPLINE_CURVE_WITH_KNOTS('',3,(#12223,#12224,#12225,#12226,#12227,
#12228,#12229,#12230,#12231,#12232,#12233,#12234,#12235,#12236,#12237,#12238,
#12239,#12240,#12241,#12242,#12243,#12244,#12245,#12246,#12247),
 .UNSPECIFIED.,.F.,.F.,(4,3,3,3,3,3,3,3,4),(-10.1295685708718,-9.97600607396309,
-8.97840546656679,-7.98080485917047,-6.98320425177416,-5.98560364437785,
-4.98800303698155,-3.99040242958524,-3.84638326369224),.UNSPECIFIED.);
#1355=B_SPLINE_CURVE_WITH_KNOTS('',3,(#12556,#12557,#12558,#12559,#12560,
#12561,#12562,#12563,#12564,#12565,#12566,#12567,#12568,#12569,#12570,#12571,
#12572,#12573,#12574,#12575,#12576,#12577,#12578,#12579,#12580,#12581,#12582,
#12583,#12584,#12585,#12586,#12587,#12588,#12589,#12590,#12591,#12592,#12593,
#12594,#12595,#12596,#12597,#12598,#12599,#12600,#12601,#12602,#12603,#12604,
#12605,#12606,#12607,#12608,#12609,#12610,#12611,#12612,#12613,#12614,#12615,
#12616,#12617,#12618,#12619,#12620,#12621,#12622,#12623,#12624,#12625,#12626,
#12627,#12628,#12629,#12630,#12631,#12632,#12633,#12634,#12635,#12636,#12637),
 .UNSPECIFIED.,.F.,.F.,(4,3,3,3,3,3,3,3,3,3,3,3,3,3,3,3,3,3,3,3,3,3,3,3,
3,3,3,4),(0.,0.018600500233587,0.0384267791159037,0.0557747731379309,0.0644820401543133,
0.0684532947198101,0.0885096834401049,0.108920567554616,0.125993108488993,
0.133863030521655,0.137292306314217,0.158366893382889,0.177210731292121,
0.197737113300186,0.205654657471879,0.209128422925177,0.230132266768946,
0.251623567767457,0.26806575224317,0.278297158812869,0.284047681225798,
0.306316607432633,0.322975646846552,0.328163948660732,0.333182233583271,
0.355703596008113,0.372952765088309,0.376940817211645),.UNSPECIFIED.);
#1356=B_SPLINE_CURVE_WITH_KNOTS('',3,(#12638,#12639,#12640,#12641,#12642,
#12643,#12644,#12645,#12646,#12647,#12648,#12649,#12650,#12651,#12652,#12653,
#12654,#12655,#12656,#12657,#12658,#12659),.UNSPECIFIED.,.F.,.F.,(4,3,3,
3,3,3,3,4),(7.59300756235153,7.98080485917048,8.97840546656679,9.97600607396309,
10.9736066813594,11.9712072887557,12.968807896152,13.8761928695311),
 .UNSPECIFIED.);
#1357=B_SPLINE_CURVE_WITH_KNOTS('',3,(#12660,#12661,#12662,#12663,#12664,
#12665,#12666,#12667,#12668,#12669,#12670,#12671,#12672,#12673,#12674,#12675,
#12676,#12677,#12678,#12679,#12680,#12681,#12682,#12683,#12684,#12685,#12686,
#12687,#12688,#12689,#12690,#12691,#12692,#12693,#12694,#12695,#12696,#12697,
#12698,#12699,#12700,#12701,#12702,#12703,#12704,#12705,#12706,#12707,#12708,
#12709,#12710,#12711,#12712,#12713,#12714,#12715,#12716,#12717,#12718,#12719,
#12720,#12721,#12722,#12723,#12724,#12725,#12726,#12727,#12728,#12729,#12730,
#12731,#12732,#12733,#12734,#12735,#12736,#12737,#12738,#12739,#12740,#12741,
#12742,#12743,#12744),.UNSPECIFIED.,.F.,.F.,(4,3,3,3,3,3,3,3,3,3,3,3,3,
3,3,3,3,3,3,3,3,3,3,3,3,3,3,3,4),(-0.376940817211633,-0.354632454605328,
-0.332909565818261,-0.328060951840561,-0.305812359536112,-0.290191982632697,
-0.284249623441465,-0.278601398679216,-0.256918509535175,-0.235701747786141,
-0.214950060594018,-0.208208596987869,-0.204399741431515,-0.183824490029494,
-0.18084934430879,-0.159866544269734,-0.140290797877594,-0.135946608670285,
-0.132579097133426,-0.112119588209322,-0.0917553067258466,-0.0718282862666161,
-0.0676047210534115,-0.063655156602234,-0.0440979256320563,-0.0249133932463398,
-0.0063528163125237,-0.00326057313262047,0.),.UNSPECIFIED.);
#1358=B_SPLINE_CURVE_WITH_KNOTS('',3,(#12782,#12783,#12784,#12785,#12786,
#12787,#12788,#12789,#12790,#12791,#12792,#12793,#12794,#12795,#12796,#12797,
#12798,#12799,#12800,#12801,#12802,#12803,#12804,#12805,#12806,#12807,#12808,
#12809,#12810,#12811,#12812,#12813,#12814,#12815,#12816,#12817,#12818,#12819,
#12820,#12821,#12822,#12823,#12824,#12825,#12826,#12827,#12828,#12829,#12830,
#12831,#12832,#12833,#12834,#12835,#12836,#12837,#12838,#12839,#12840,#12841,
#12842,#12843,#12844,#12845,#12846,#12847,#12848,#12849,#12850,#12851,#12852,
#12853,#12854,#12855,#12856,#12857,#12858,#12859,#12860,#12861,#12862,#12863,
#12864,#12865,#12866),.UNSPECIFIED.,.F.,.F.,(4,3,3,3,3,3,3,3,3,3,3,3,3,
3,3,3,3,3,3,3,3,3,3,3,3,3,3,3,4),(0.,0.021968619134099,0.0445463508138711,
0.0636241950320315,0.0720974452774801,0.0767548527122233,0.0810487295372733,
0.102995302809976,0.124770868754624,0.142870427705757,0.150424219455889,
0.153922404976729,0.157567538938561,0.178337436410292,0.197169104559154,
0.219441601244656,0.22434621853845,0.229396798911011,0.250061926915346,
0.270722751583954,0.285678803759607,0.296896065746556,0.300623776312427,
0.320395169261119,0.334310908061463,0.33877648878019,0.357799740024219,
0.375349078043172,0.378621596831398),.UNSPECIFIED.);
#1359=B_SPLINE_CURVE_WITH_KNOTS('',3,(#12867,#12868,#12869,#12870,#12871,
#12872,#12873,#12874,#12875,#12876,#12877,#12878,#12879,#12880,#12881,#12882,
#12883,#12884,#12885,#12886,#12887,#12888,#12889,#12890,#12891,#12892,#12893,
#12894,#12895,#12896,#12897,#12898,#12899,#12900,#12901,#12902,#12903,#12904,
#12905,#12906,#12907,#12908,#12909,#12910,#12911,#12912,#12913,#12914,#12915,
#12916,#12917,#12918,#12919,#12920,#12921,#12922,#12923,#12924,#12925,#12926,
#12927,#12928,#12929,#12930,#12931,#12932,#12933,#12934,#12935,#12936,#12937,
#12938,#12939,#12940,#12941,#12942,#12943,#12944,#12945,#12946,#12947,#12948),
 .UNSPECIFIED.,.F.,.F.,(4,3,3,3,3,3,3,3,3,3,3,3,3,3,3,3,3,3,3,3,3,3,3,3,
3,3,3,4),(0.,0.0186005373117356,0.038426811559284,0.0557748015258888,0.0644820892685102,
0.0684533078055671,0.0885097227040427,0.108920617705581,0.125993146102217,
0.133863089681963,0.137292338809663,0.158366921726846,0.177210731292123,
0.197737094100997,0.205654646587328,0.20912841497494,0.23013223615724,0.251623525403939,
0.268065761427934,0.278297179882888,0.284047675336949,0.306316600241872,
0.32297564145348,0.328163936759366,0.333182227701541,0.355703590029263,
0.372952765088304,0.37694081721164),.UNSPECIFIED.);
#1360=B_SPLINE_CURVE_WITH_KNOTS('',3,(#12949,#12950,#12951,#12952,#12953,
#12954,#12955,#12956,#12957,#12958,#12959,#12960,#12961,#12962,#12963,#12964,
#12965,#12966,#12967,#12968,#12969,#12970,#12971,#12972,#12973,#12974,#12975,
#12976,#12977,#12978,#12979,#12980,#12981,#12982,#12983,#12984,#12985,#12986,
#12987,#12988,#12989,#12990,#12991,#12992,#12993,#12994,#12995,#12996,#12997,
#12998,#12999,#13000,#13001,#13002,#13003,#13004,#13005,#13006,#13007,#13008,
#13009,#13010,#13011,#13012,#13013,#13014,#13015,#13016,#13017,#13018,#13019,
#13020,#13021,#13022,#13023,#13024,#13025,#13026,#13027,#13028,#13029,#13030,
#13031,#13032,#13033),.UNSPECIFIED.,.F.,.F.,(4,3,3,3,3,3,3,3,3,3,3,3,3,
3,3,3,3,3,3,3,3,3,3,3,3,3,3,3,4),(0.,0.0219686380514027,0.0445463713382339,
0.0636242129908502,0.0720974506611356,0.0767548640568597,0.0810487326131753,
0.102995305281134,0.124770865263899,0.142870425087715,0.150424220061154,
0.153922409603196,0.157567540562184,0.178337432135944,0.197169104559165,
0.219441601244671,0.224346216685054,0.229396798808629,0.250061927461599,
0.270722751034184,0.285678784130498,0.296896032726582,0.300623767000752,
0.320395152261939,0.334310880229888,0.338776462161233,0.357799701520601,
0.375349078043213,0.378621596831437),.UNSPECIFIED.);
#1361=B_SPLINE_CURVE_WITH_KNOTS('',3,(#13034,#13035,#13036,#13037,#13038,
#13039,#13040,#13041,#13042,#13043,#13044,#13045,#13046,#13047,#13048,#13049,
#13050,#13051,#13052,#13053,#13054,#13055,#13056,#13057,#13058,#13059,#13060,
#13061,#13062,#13063,#13064,#13065,#13066,#13067,#13068,#13069,#13070,#13071,
#13072,#13073,#13074,#13075,#13076,#13077,#13078,#13079,#13080,#13081,#13082,
#13083,#13084,#13085,#13086,#13087,#13088,#13089,#13090,#13091,#13092,#13093,
#13094,#13095,#13096,#13097,#13098,#13099,#13100,#13101,#13102,#13103,#13104,
#13105,#13106,#13107,#13108,#13109,#13110,#13111,#13112,#13113,#13114,#13115),
 .UNSPECIFIED.,.F.,.F.,(4,3,3,3,3,3,3,3,3,3,3,3,3,3,3,3,3,3,3,3,3,3,3,3,
3,3,3,4),(0.,0.0186005115768008,0.038426789041218,0.055774781822583,0.06448205517952,
0.0684532987383391,0.088509695468686,0.108920582912668,0.125993120007535,
0.133863048637895,0.137292316222759,0.158366902021944,0.177210731292138,
0.197737107427825,0.205654654143849,0.209128420488014,0.230132257400709,
0.251623554805102,0.268065755057508,0.278297165271629,0.284047679418564,
0.306316605227149,0.322975645192443,0.328163945080186,0.333182231795999,
0.355703594193589,0.372952765088323,0.376940817211659),.UNSPECIFIED.);
#1362=B_SPLINE_CURVE_WITH_KNOTS('',3,(#13116,#13117,#13118,#13119,#13120,
#13121,#13122,#13123,#13124,#13125,#13126,#13127,#13128,#13129,#13130,#13131,
#13132,#13133,#13134,#13135,#13136,#13137,#13138,#13139,#13140,#13141,#13142,
#13143,#13144,#13145,#13146,#13147,#13148,#13149,#13150,#13151,#13152,#13153,
#13154,#13155,#13156,#13157,#13158,#13159,#13160,#13161,#13162,#13163,#13164,
#13165,#13166,#13167,#13168,#13169,#13170,#13171,#13172,#13173,#13174,#13175,
#13176,#13177,#13178,#13179,#13180,#13181,#13182,#13183,#13184,#13185,#13186,
#13187,#13188,#13189,#13190,#13191,#13192,#13193,#13194,#13195,#13196,#13197,
#13198,#13199,#13200),.UNSPECIFIED.,.F.,.F.,(4,3,3,3,3,3,3,3,3,3,3,3,3,
3,3,3,3,3,3,3,3,3,3,3,3,3,3,3,4),(0.,0.0219686109476892,0.0445463419311616,
0.0636241872596606,0.072097442945625,0.0767548477970364,0.0810487282633608,
0.102995301796811,0.124770870320527,0.142870428880184,0.150424219224462,
0.15392240302136,0.157567538243027,0.178337438267784,0.197169104559153,
0.219441601244657,0.224346219340572,0.229396798953165,0.250061926675953,
0.270722751817935,0.285678812243067,0.296896080015907,0.300623780338084,
0.320395176613474,0.334310920099279,0.338776500225901,0.357799756613675,
0.375349078043179,0.378621596831404),.UNSPECIFIED.);
#1363=B_SPLINE_CURVE_WITH_KNOTS('',3,(#13201,#13202,#13203,#13204,#13205,
#13206,#13207,#13208,#13209,#13210,#13211,#13212,#13213,#13214,#13215,#13216,
#13217,#13218,#13219,#13220,#13221,#13222,#13223,#13224,#13225,#13226,#13227,
#13228,#13229,#13230,#13231,#13232,#13233,#13234,#13235,#13236,#13237,#13238,
#13239,#13240,#13241,#13242,#13243,#13244,#13245,#13246,#13247,#13248,#13249,
#13250,#13251,#13252,#13253,#13254,#13255,#13256,#13257,#13258,#13259,#13260,
#13261,#13262,#13263,#13264,#13265,#13266,#13267,#13268,#13269,#13270,#13271,
#13272,#13273,#13274,#13275,#13276,#13277,#13278,#13279,#13280,#13281,#13282),
 .UNSPECIFIED.,.F.,.F.,(4,3,3,3,3,3,3,3,3,3,3,3,3,3,3,3,3,3,3,3,3,3,3,3,
3,3,3,4),(0.,0.0186005239390001,0.0384267998581411,0.0557747912873894,0.0644820715548053,
0.0684533030913493,0.0885097085463574,0.108920599618628,0.125993132537003,
0.133863068345662,0.137292327044492,0.158366911460439,0.177210731292128,
0.197737101028813,0.205654650516969,0.209128417840175,0.230132247197424,
0.251623540683617,0.268065758119471,0.278297172296056,0.284047677474677,
0.306316602850204,0.322975643409731,0.328163941106245,0.333182229833608,
0.355703592197711,0.372952765088311,0.376940817211644),.UNSPECIFIED.);
#1364=B_SPLINE_CURVE_WITH_KNOTS('',3,(#13284,#13285,#13286,#13287,#13288,
#13289,#13290,#13291,#13292,#13293,#13294),.UNSPECIFIED.,.F.,.F.,(4,1,1,
1,1,1,1,1,4),(15.7079632679489,15.8519824338419,16.8495830412382,17.8471836486345,
18.8447842560308,19.8423848634271,20.8399854708235,21.8375860782198,21.9911485751285),
 .UNSPECIFIED.);
#1365=B_SPLINE_CURVE_WITH_KNOTS('',3,(#13295,#13296,#13297,#13298,#13299,
#13300,#13301,#13302,#13303,#13304),.UNSPECIFIED.,.F.,.F.,(4,1,1,1,1,1,
1,4),(15.7079632679489,16.3933422275695,17.3909428349659,18.3885434423622,
19.3861440497585,20.3837446571548,21.3813452645511,21.9911485751285),
 .UNSPECIFIED.);
#1366=B_SPLINE_CURVE_WITH_KNOTS('',3,(#13613,#13614,#13615,#13616,#13617,
#13618,#13619,#13620,#13621,#13622,#13623,#13624,#13625,#13626,#13627,#13628,
#13629,#13630,#13631,#13632,#13633,#13634,#13635,#13636,#13637,#13638,#13639,
#13640,#13641,#13642,#13643,#13644,#13645,#13646,#13647,#13648,#13649,#13650,
#13651,#13652,#13653,#13654,#13655,#13656,#13657,#13658,#13659,#13660,#13661,
#13662,#13663,#13664,#13665,#13666,#13667,#13668,#13669,#13670,#13671,#13672,
#13673,#13674,#13675,#13676,#13677,#13678,#13679,#13680,#13681,#13682,#13683,
#13684,#13685,#13686,#13687,#13688,#13689,#13690,#13691,#13692,#13693,#13694,
#13695,#13696,#13697,#13698,#13699,#13700),.UNSPECIFIED.,.F.,.F.,(4,3,3,
3,3,3,3,3,3,3,3,3,3,3,3,3,3,3,3,3,3,3,3,3,3,3,3,3,3,4),(-0.378621596831427,
-0.359794625220292,-0.347847845255257,-0.339608528850609,-0.335317716276224,
-0.315442613111551,-0.301115286145566,-0.297116173616389,-0.293205026311676,
-0.272800449719613,-0.252103127039742,-0.239283344625725,-0.22876814535061,
-0.224492807264877,-0.203188357883528,-0.200823997383671,-0.180338493313755,
-0.158296751019492,-0.154234157832905,-0.15079163756267,-0.12940956273182,
-0.107575843179879,-0.0856092627735954,-0.0801786890662741,-0.0759363558949484,
-0.0533889736446962,-0.0308167632838699,-0.00875885575216316,-0.00400455495965028,
0.),.UNSPECIFIED.);
#1367=B_SPLINE_CURVE_WITH_KNOTS('',3,(#13701,#13702,#13703,#13704,#13705,
#13706,#13707,#13708,#13709,#13710,#13711,#13712,#13713,#13714,#13715,#13716,
#13717,#13718,#13719,#13720,#13721,#13722,#13723,#13724,#13725),
 .UNSPECIFIED.,.F.,.F.,(4,3,3,3,3,3,3,3,4),(-10.1295685708718,-9.97600607396309,
-8.97840546656678,-7.98080485917047,-6.98320425177416,-5.98560364437785,
-4.98800303698155,-3.99040242958523,-3.84638326369224),.UNSPECIFIED.);
#1368=B_SPLINE_CURVE_WITH_KNOTS('',3,(#14034,#14035,#14036,#14037,#14038,
#14039,#14040,#14041,#14042,#14043,#14044,#14045,#14046,#14047,#14048,#14049,
#14050,#14051,#14052,#14053,#14054,#14055),.UNSPECIFIED.,.F.,.F.,(4,3,3,
3,3,3,3,4),(7.59300756235153,7.98080485917047,8.97840546656678,9.9760060739631,
10.9736066813594,11.9712072887557,12.968807896152,13.8761928695311),
 .UNSPECIFIED.);
#1369=B_SPLINE_CURVE_WITH_KNOTS('',3,(#14056,#14057,#14058,#14059,#14060,
#14061,#14062,#14063,#14064,#14065,#14066,#14067,#14068,#14069,#14070,#14071,
#14072,#14073,#14074,#14075,#14076,#14077,#14078,#14079,#14080,#14081,#14082,
#14083,#14084,#14085,#14086,#14087,#14088,#14089,#14090,#14091,#14092,#14093,
#14094,#14095,#14096,#14097,#14098,#14099,#14100,#14101,#14102,#14103,#14104,
#14105,#14106,#14107,#14108,#14109,#14110,#14111,#14112,#14113,#14114,#14115,
#14116,#14117,#14118,#14119,#14120,#14121,#14122,#14123,#14124,#14125,#14126,
#14127,#14128,#14129,#14130,#14131,#14132,#14133,#14134,#14135,#14136,#14137,
#14138,#14139,#14140),.UNSPECIFIED.,.F.,.F.,(4,3,3,3,3,3,3,3,3,3,3,3,3,
3,3,3,3,3,3,3,3,3,3,3,3,3,3,3,4),(-0.376940817211658,-0.354632440305215,
-0.332909553305663,-0.328060937224979,-0.305812345362663,-0.29019197023093,
-0.284249595905682,-0.278601400527098,-0.25691851401837,-0.23570175863681,
-0.214950075630617,-0.208208587756039,-0.204399742947041,-0.183824497720044,
-0.180849344308799,-0.159866544391984,-0.140290797984564,-0.135946620453725,
-0.132579106908657,-0.11211959722078,-0.0917553180086424,-0.0718283063725309,
-0.0676047765030496,-0.0636551755593219,-0.0440979496009447,-0.0249134276262131,
-0.00635286745037528,-0.00326057313262046,0.),.UNSPECIFIED.);
#1370=B_SPLINE_CURVE_WITH_KNOTS('',3,(#14142,#14143,#14144,#14145,#14146,
#14147,#14148,#14149,#14150,#14151,#14152),.UNSPECIFIED.,.F.,.F.,(4,1,1,
1,1,1,1,1,4),(15.7079632679489,15.8519824338419,16.8495830412382,17.8471836486345,
18.8447842560308,19.8423848634271,20.8399854708235,21.8375860782198,21.9911485751285),
 .UNSPECIFIED.);
#1371=B_SPLINE_CURVE_WITH_KNOTS('',3,(#14153,#14154,#14155,#14156,#14157,
#14158,#14159,#14160,#14161,#14162),.UNSPECIFIED.,.F.,.F.,(4,1,1,1,1,1,
1,4),(15.7079632679489,16.3933422275695,17.3909428349659,18.3885434423622,
19.3861440497585,20.3837446571548,21.3813452645511,21.9911485751285),
 .UNSPECIFIED.);
#1372=B_SPLINE_CURVE_WITH_KNOTS('',3,(#14471,#14472,#14473,#14474,#14475,
#14476,#14477,#14478,#14479,#14480,#14481,#14482,#14483,#14484,#14485,#14486,
#14487,#14488,#14489,#14490,#14491,#14492,#14493,#14494,#14495,#14496,#14497,
#14498,#14499,#14500,#14501,#14502,#14503,#14504,#14505,#14506,#14507,#14508,
#14509,#14510,#14511,#14512,#14513,#14514,#14515,#14516,#14517,#14518,#14519,
#14520,#14521,#14522,#14523,#14524,#14525,#14526,#14527,#14528,#14529,#14530,
#14531,#14532,#14533,#14534,#14535,#14536,#14537,#14538,#14539,#14540,#14541,
#14542,#14543,#14544,#14545,#14546,#14547,#14548,#14549,#14550,#14551,#14552,
#14553,#14554,#14555,#14556,#14557,#14558),.UNSPECIFIED.,.F.,.F.,(4,3,3,
3,3,3,3,3,3,3,3,3,3,3,3,3,3,3,3,3,3,3,3,3,3,3,3,3,3,4),(-0.378621596831439,
-0.35979459391274,-0.347847765628199,-0.339607786177388,-0.335317210572095,
-0.315442075259891,-0.301114815525364,-0.297115056007226,-0.293204827194635,
-0.272800226631742,-0.25210290804161,-0.239283180377127,-0.228767902917728,
-0.22449272396701,-0.203188276512031,-0.200823997383678,-0.180338515496785,
-0.158296770429644,-0.154234295176689,-0.150791667121598,-0.129409610366437,
-0.107575898692758,-0.0856093183754116,-0.0801787858574953,-0.0759363909673205,
-0.0533890123327845,-0.0308168013567995,-0.00875889812582652,-0.00400455495965099,
0.),.UNSPECIFIED.);
#1373=B_SPLINE_CURVE_WITH_KNOTS('',3,(#14559,#14560,#14561,#14562,#14563,
#14564,#14565,#14566,#14567,#14568,#14569,#14570,#14571,#14572,#14573,#14574,
#14575,#14576,#14577,#14578,#14579,#14580,#14581,#14582,#14583),
 .UNSPECIFIED.,.F.,.F.,(4,3,3,3,3,3,3,3,4),(-10.1295685708718,-9.97600607396309,
-8.97840546656678,-7.98080485917047,-6.98320425177416,-5.98560364437785,
-4.98800303698155,-3.99040242958524,-3.84638326369225),.UNSPECIFIED.);
#1374=B_SPLINE_CURVE_WITH_KNOTS('',3,(#14892,#14893,#14894,#14895,#14896,
#14897,#14898,#14899,#14900,#14901,#14902,#14903,#14904,#14905,#14906,#14907,
#14908,#14909,#14910,#14911,#14912,#14913),.UNSPECIFIED.,.F.,.F.,(4,3,3,
3,3,3,3,4),(7.59300756235153,7.98080485917047,8.97840546656678,9.9760060739631,
10.9736066813594,11.9712072887557,12.968807896152,13.8761928695311),
 .UNSPECIFIED.);
#1375=B_SPLINE_CURVE_WITH_KNOTS('',3,(#14914,#14915,#14916,#14917,#14918,
#14919,#14920,#14921,#14922,#14923,#14924,#14925,#14926,#14927,#14928,#14929,
#14930,#14931,#14932,#14933,#14934,#14935,#14936,#14937,#14938,#14939,#14940,
#14941,#14942,#14943,#14944,#14945,#14946,#14947,#14948,#14949,#14950,#14951,
#14952,#14953,#14954,#14955,#14956,#14957,#14958,#14959,#14960,#14961,#14962,
#14963,#14964,#14965,#14966,#14967,#14968,#14969,#14970,#14971,#14972,#14973,
#14974,#14975,#14976,#14977,#14978,#14979,#14980,#14981,#14982,#14983,#14984,
#14985,#14986,#14987,#14988,#14989,#14990,#14991,#14992,#14993,#14994,#14995,
#14996,#14997,#14998),.UNSPECIFIED.,.F.,.F.,(4,3,3,3,3,3,3,3,3,3,3,3,3,
3,3,3,3,3,3,3,3,3,3,3,3,3,3,3,4),(-0.376940817211635,-0.354632447762244,
-0.332909559830562,-0.32806094484179,-0.305812352748728,-0.290191976693736,
-0.284249610255867,-0.278601399566055,-0.256918511682903,-0.235701752980436,
-0.214950067791438,-0.208208592568691,-0.204399742168023,-0.183824493720622,
-0.180849344308789,-0.159866544328361,-0.140290797928894,-0.135946614308445,
-0.132579101815663,-0.112119592526046,-0.0917553121288918,-0.0718282958900664,
-0.0676047475926938,-0.0636551656772768,-0.0440979371043374,-0.0249134096995733,
-0.00635284078267037,-0.00326057313262106,0.),.UNSPECIFIED.);
#1376=B_SPLINE_CURVE_WITH_KNOTS('',3,(#15000,#15001,#15002,#15003,#15004,
#15005,#15006,#15007,#15008,#15009,#15010),.UNSPECIFIED.,.F.,.F.,(4,1,1,
1,1,1,1,1,4),(15.7079632679489,15.8519824338419,16.8495830412382,17.8471836486345,
18.8447842560309,19.8423848634272,20.8399854708235,21.8375860782198,21.9911485751285),
 .UNSPECIFIED.);
#1377=B_SPLINE_CURVE_WITH_KNOTS('',3,(#15011,#15012,#15013,#15014,#15015,
#15016,#15017,#15018,#15019,#15020),.UNSPECIFIED.,.F.,.F.,(4,1,1,1,1,1,
1,4),(15.7079632679489,16.3933422275696,17.3909428349659,18.3885434423622,
19.3861440497585,20.3837446571548,21.3813452645511,21.9911485751285),
 .UNSPECIFIED.);
#1378=B_SPLINE_CURVE_WITH_KNOTS('',3,(#15329,#15330,#15331,#15332,#15333,
#15334,#15335,#15336,#15337,#15338,#15339,#15340,#15341,#15342,#15343,#15344,
#15345,#15346,#15347,#15348,#15349,#15350,#15351,#15352,#15353,#15354,#15355,
#15356,#15357,#15358,#15359,#15360,#15361,#15362,#15363,#15364,#15365,#15366,
#15367,#15368,#15369,#15370,#15371,#15372,#15373,#15374,#15375,#15376,#15377,
#15378,#15379,#15380,#15381,#15382,#15383,#15384,#15385,#15386,#15387,#15388,
#15389,#15390,#15391,#15392,#15393,#15394,#15395,#15396,#15397,#15398,#15399,
#15400,#15401,#15402,#15403,#15404,#15405,#15406,#15407,#15408,#15409,#15410,
#15411,#15412,#15413,#15414,#15415,#15416),.UNSPECIFIED.,.F.,.F.,(4,3,3,
3,3,3,3,3,3,3,3,3,3,3,3,3,3,3,3,3,3,3,3,3,3,3,3,3,3,4),(-0.378621596831402,
-0.359794615761403,-0.347847821197377,-0.339608304483908,-0.335317563605001,
-0.315442450729176,-0.301115144060986,-0.297115836250077,-0.293204966248274,
-0.272800382415427,-0.252103060970179,-0.23928329507355,-0.228768072211328,
-0.224492782138973,-0.203188333339894,-0.200823997383662,-0.180338500015385,
-0.158296756883418,-0.154234199332552,-0.150791646494627,-0.129409577124881,
-0.107575859953488,-0.0856092795738859,-0.0801787183117794,-0.0759363664912861,
-0.0533889853334927,-0.0308167747861896,-0.00875886855324413,-0.00400455495965136,
0.),.UNSPECIFIED.);
#1379=B_SPLINE_CURVE_WITH_KNOTS('',3,(#15417,#15418,#15419,#15420,#15421,
#15422,#15423,#15424,#15425,#15426,#15427,#15428,#15429,#15430,#15431,#15432,
#15433,#15434,#15435,#15436,#15437,#15438,#15439,#15440,#15441),
 .UNSPECIFIED.,.F.,.F.,(4,3,3,3,3,3,3,3,4),(-10.1295685708718,-9.97600607396309,
-8.97840546656678,-7.98080485917047,-6.98320425177416,-5.98560364437786,
-4.98800303698154,-3.99040242958524,-3.84638326369224),.UNSPECIFIED.);
#1380=B_SPLINE_CURVE_WITH_KNOTS('',3,(#15750,#15751,#15752,#15753,#15754,
#15755,#15756,#15757,#15758,#15759,#15760,#15761,#15762,#15763,#15764,#15765,
#15766,#15767,#15768,#15769,#15770,#15771),.UNSPECIFIED.,.F.,.F.,(4,3,3,
3,3,3,3,4),(7.59300756235153,7.98080485917048,8.97840546656678,9.9760060739631,
10.9736066813594,11.9712072887557,12.968807896152,13.8761928695311),
 .UNSPECIFIED.);
#1381=B_SPLINE_CURVE_WITH_KNOTS('',3,(#15772,#15773,#15774,#15775,#15776,
#15777,#15778,#15779,#15780,#15781,#15782,#15783,#15784,#15785,#15786,#15787,
#15788,#15789,#15790,#15791,#15792,#15793,#15794,#15795,#15796,#15797,#15798,
#15799,#15800,#15801,#15802),.UNSPECIFIED.,.F.,.F.,(4,3,3,3,3,3,3,3,3,3,
4),(0.050378130562488,0.0706766774202748,0.0909513952302104,0.110830379637232,
0.119055313841064,0.122780653122509,0.126719562075065,0.146060569004475,
0.164791269949457,0.170467332858295,0.173733289126884),.UNSPECIFIED.);
#1382=B_SPLINE_CURVE_WITH_KNOTS('',3,(#15803,#15804,#15805,#15806,#15807,
#15808,#15809,#15810,#15811,#15812,#15813,#15814,#15815,#15816,#15817,#15818,
#15819,#15820,#15821,#15822,#15823,#15824,#15825,#15826,#15827,#15828,#15829,
#15830,#15831,#15832,#15833,#15834,#15835,#15836,#15837,#15838,#15839,#15840,
#15841,#15842,#15843,#15844,#15845,#15846,#15847,#15848,#15849,#15850,#15851,
#15852,#15853,#15854,#15855,#15856,#15857,#15858,#15859,#15860),
 .UNSPECIFIED.,.F.,.F.,(4,3,3,3,3,3,3,3,3,3,3,3,3,3,3,3,3,3,3,4),(-0.376940817211632,
-0.354632432238001,-0.332909546246849,-0.328060928965978,-0.305812337354451,
-0.290191963223743,-0.284249580349225,-0.278601401578559,-0.256918516557476,
-0.235701764768698,-0.214950084124798,-0.20820858254272,-0.204399743801857,
-0.183824502058691,-0.18084934430879,-0.159816080827987,-0.141544175656564,
-0.136361698528752,-0.132490636717292,-0.123272270485141),.UNSPECIFIED.);
#1529=LINE('',#8358,#1985);
#1530=LINE('',#8397,#1986);
#1531=LINE('',#8445,#1987);
#1532=LINE('',#8493,#1988);
#1533=LINE('',#8544,#1989);
#1534=LINE('',#8592,#1990);
#1535=LINE('',#8640,#1991);
#1536=LINE('',#8691,#1992);
#1537=LINE('',#8742,#1993);
#1538=LINE('',#8790,#1994);
#1539=LINE('',#8841,#1995);
#1540=LINE('',#8880,#1996);
#1541=LINE('',#8919,#1997);
#1542=LINE('',#8967,#1998);
#1543=LINE('',#9015,#1999);
#1544=LINE('',#9066,#2000);
#1545=LINE('',#9114,#2001);
#1546=LINE('',#9162,#2002);
#1547=LINE('',#9213,#2003);
#1548=LINE('',#9264,#2004);
#1549=LINE('',#9312,#2005);
#1550=LINE('',#9363,#2006);
#1551=LINE('',#9402,#2007);
#1552=LINE('',#9441,#2008);
#1553=LINE('',#9489,#2009);
#1554=LINE('',#9537,#2010);
#1555=LINE('',#9588,#2011);
#1556=LINE('',#9636,#2012);
#1557=LINE('',#9684,#2013);
#1558=LINE('',#9735,#2014);
#1559=LINE('',#9786,#2015);
#1560=LINE('',#9834,#2016);
#1561=LINE('',#9885,#2017);
#1562=LINE('',#9926,#2018);
#1563=LINE('',#9965,#2019);
#1564=LINE('',#10013,#2020);
#1565=LINE('',#10061,#2021);
#1566=LINE('',#10112,#2022);
#1567=LINE('',#10160,#2023);
#1568=LINE('',#10208,#2024);
#1569=LINE('',#10259,#2025);
#1570=LINE('',#10310,#2026);
#1571=LINE('',#10358,#2027);
#1572=LINE('',#10409,#2028);
#1573=LINE('',#10450,#2029);
#1574=LINE('',#10466,#2030);
#1575=LINE('',#10491,#2031);
#1576=LINE('',#10516,#2032);
#1577=LINE('',#10540,#2033);
#1578=LINE('',#10565,#2034);
#1579=LINE('',#10589,#2035);
#1580=LINE('',#10614,#2036);
#1581=LINE('',#10638,#2037);
#1582=LINE('',#10663,#2038);
#1583=LINE('',#10688,#2039);
#1584=LINE('',#10712,#2040);
#1585=LINE('',#10729,#2041);
#1586=LINE('',#10745,#2042);
#1587=LINE('',#10770,#2043);
#1588=LINE('',#10795,#2044);
#1589=LINE('',#10819,#2045);
#1590=LINE('',#10844,#2046);
#1591=LINE('',#10868,#2047);
#1592=LINE('',#10893,#2048);
#1593=LINE('',#10917,#2049);
#1594=LINE('',#10942,#2050);
#1595=LINE('',#10967,#2051);
#1596=LINE('',#10991,#2052);
#1597=LINE('',#11008,#2053);
#1598=LINE('',#11024,#2054);
#1599=LINE('',#11049,#2055);
#1600=LINE('',#11074,#2056);
#1601=LINE('',#11098,#2057);
#1602=LINE('',#11123,#2058);
#1603=LINE('',#11147,#2059);
#1604=LINE('',#11172,#2060);
#1605=LINE('',#11196,#2061);
#1606=LINE('',#11221,#2062);
#1607=LINE('',#11246,#2063);
#1608=LINE('',#11270,#2064);
#1609=LINE('',#11287,#2065);
#1610=LINE('',#11303,#2066);
#1611=LINE('',#11328,#2067);
#1612=LINE('',#11353,#2068);
#1613=LINE('',#11377,#2069);
#1614=LINE('',#11402,#2070);
#1615=LINE('',#11426,#2071);
#1616=LINE('',#11451,#2072);
#1617=LINE('',#11475,#2073);
#1618=LINE('',#11500,#2074);
#1619=LINE('',#11525,#2075);
#1620=LINE('',#11549,#2076);
#1621=LINE('',#11566,#2077);
#1622=LINE('',#11570,#2078);
#1623=LINE('',#11574,#2079);
#1624=LINE('',#11577,#2080);
#1625=LINE('',#11580,#2081);
#1626=LINE('',#11583,#2082);
#1627=LINE('',#11586,#2083);
#1628=LINE('',#11589,#2084);
#1629=LINE('',#11592,#2085);
#1630=LINE('',#11594,#2086);
#1631=LINE('',#11597,#2087);
#1632=LINE('',#11598,#2088);
#1633=LINE('',#11601,#2089);
#1634=LINE('',#11603,#2090);
#1635=LINE('',#11605,#2091);
#1636=LINE('',#11607,#2092);
#1637=LINE('',#11608,#2093);
#1638=LINE('',#11611,#2094);
#1639=LINE('',#11612,#2095);
#1640=LINE('',#11613,#2096);
#1641=LINE('',#11616,#2097);
#1642=LINE('',#11617,#2098);
#1643=LINE('',#11621,#2099);
#1644=LINE('',#11625,#2100);
#1645=LINE('',#11627,#2101);
#1646=LINE('',#11629,#2102);
#1647=LINE('',#11635,#2103);
#1648=LINE('',#11636,#2104);
#1649=LINE('',#11662,#2105);
#1650=LINE('',#11667,#2106);
#1651=LINE('',#11689,#2107);
#1652=LINE('',#11691,#2108);
#1653=LINE('',#11694,#2109);
#1654=LINE('',#11696,#2110);
#1655=LINE('',#11697,#2111);
#1656=LINE('',#11700,#2112);
#1657=LINE('',#11701,#2113);
#1658=LINE('',#11716,#2114);
#1659=LINE('',#11720,#2115);
#1660=LINE('',#12748,#2116);
#1661=LINE('',#12750,#2117);
#1662=LINE('',#12752,#2118);
#1663=LINE('',#12754,#2119);
#1664=LINE('',#12756,#2120);
#1665=LINE('',#12757,#2121);
#1666=LINE('',#12760,#2122);
#1667=LINE('',#12762,#2123);
#1668=LINE('',#12764,#2124);
#1669=LINE('',#12765,#2125);
#1670=LINE('',#12768,#2126);
#1671=LINE('',#12770,#2127);
#1672=LINE('',#12772,#2128);
#1673=LINE('',#12773,#2129);
#1674=LINE('',#12776,#2130);
#1675=LINE('',#12778,#2131);
#1676=LINE('',#12780,#2132);
#1677=LINE('',#12781,#2133);
#1678=LINE('',#15863,#2134);
#1679=LINE('',#15865,#2135);
#1680=LINE('',#15866,#2136);
#1681=LINE('',#15869,#2137);
#1682=LINE('',#15871,#2138);
#1683=LINE('',#15873,#2139);
#1684=LINE('',#15874,#2140);
#1685=LINE('',#15877,#2141);
#1686=LINE('',#15879,#2142);
#1687=LINE('',#15881,#2143);
#1688=LINE('',#15882,#2144);
#1689=LINE('',#15885,#2145);
#1690=LINE('',#15887,#2146);
#1691=LINE('',#15889,#2147);
#1692=LINE('',#15890,#2148);
#1693=LINE('',#15894,#2149);
#1694=LINE('',#15901,#2150);
#1695=LINE('',#15902,#2151);
#1696=LINE('',#15904,#2152);
#1697=LINE('',#15906,#2153);
#1698=LINE('',#15909,#2154);
#1699=LINE('',#15910,#2155);
#1700=LINE('',#15912,#2156);
#1701=LINE('',#15914,#2157);
#1702=LINE('',#15917,#2158);
#1703=LINE('',#15918,#2159);
#1704=LINE('',#15920,#2160);
#1705=LINE('',#15922,#2161);
#1706=LINE('',#15926,#2162);
#1707=LINE('',#15927,#2163);
#1708=LINE('',#15930,#2164);
#1709=LINE('',#15932,#2165);
#1710=LINE('',#15934,#2166);
#1711=LINE('',#15936,#2167);
#1712=LINE('',#15938,#2168);
#1713=LINE('',#15939,#2169);
#1714=LINE('',#15941,#2170);
#1715=LINE('',#15944,#2171);
#1716=LINE('',#15946,#2172);
#1717=LINE('',#15948,#2173);
#1718=LINE('',#15949,#2174);
#1719=LINE('',#15951,#2175);
#1720=LINE('',#15953,#2176);
#1721=LINE('',#15956,#2177);
#1722=LINE('',#15958,#2178);
#1985=VECTOR('',#6973,2.);
#1986=VECTOR('',#6978,2.);
#1987=VECTOR('',#6981,2.);
#1988=VECTOR('',#6984,2.);
#1989=VECTOR('',#6987,2.);
#1990=VECTOR('',#6990,2.);
#1991=VECTOR('',#6993,2.);
#1992=VECTOR('',#6996,2.);
#1993=VECTOR('',#6999,2.);
#1994=VECTOR('',#7002,2.);
#1995=VECTOR('',#7005,2.);
#1996=VECTOR('',#7010,2.);
#1997=VECTOR('',#7015,2.);
#1998=VECTOR('',#7018,2.);
#1999=VECTOR('',#7021,2.);
#2000=VECTOR('',#7024,2.);
#2001=VECTOR('',#7027,2.);
#2002=VECTOR('',#7030,2.);
#2003=VECTOR('',#7033,2.);
#2004=VECTOR('',#7036,2.);
#2005=VECTOR('',#7039,2.);
#2006=VECTOR('',#7042,2.);
#2007=VECTOR('',#7047,2.);
#2008=VECTOR('',#7052,2.);
#2009=VECTOR('',#7055,2.);
#2010=VECTOR('',#7058,2.);
#2011=VECTOR('',#7061,2.);
#2012=VECTOR('',#7064,2.);
#2013=VECTOR('',#7067,2.);
#2014=VECTOR('',#7070,2.);
#2015=VECTOR('',#7073,2.);
#2016=VECTOR('',#7076,2.);
#2017=VECTOR('',#7079,2.);
#2018=VECTOR('',#7086,2.);
#2019=VECTOR('',#7091,2.);
#2020=VECTOR('',#7094,2.);
#2021=VECTOR('',#7097,2.);
#2022=VECTOR('',#7100,2.);
#2023=VECTOR('',#7103,2.);
#2024=VECTOR('',#7106,2.);
#2025=VECTOR('',#7109,2.);
#2026=VECTOR('',#7112,2.);
#2027=VECTOR('',#7115,2.);
#2028=VECTOR('',#7118,2.);
#2029=VECTOR('',#7125,2.05475);
#2030=VECTOR('',#7130,2.05475);
#2031=VECTOR('',#7133,2.05475);
#2032=VECTOR('',#7136,2.05475);
#2033=VECTOR('',#7139,2.05475);
#2034=VECTOR('',#7142,2.05475);
#2035=VECTOR('',#7145,2.05475);
#2036=VECTOR('',#7148,2.05475);
#2037=VECTOR('',#7151,2.05475);
#2038=VECTOR('',#7154,2.05475);
#2039=VECTOR('',#7157,2.05475);
#2040=VECTOR('',#7160,2.05475);
#2041=VECTOR('',#7165,2.05475);
#2042=VECTOR('',#7170,2.05475);
#2043=VECTOR('',#7173,2.05475);
#2044=VECTOR('',#7176,2.05475);
#2045=VECTOR('',#7179,2.05475);
#2046=VECTOR('',#7182,2.05475);
#2047=VECTOR('',#7185,2.05475);
#2048=VECTOR('',#7188,2.05475);
#2049=VECTOR('',#7191,2.05475);
#2050=VECTOR('',#7194,2.05475);
#2051=VECTOR('',#7197,2.05475);
#2052=VECTOR('',#7200,2.05475);
#2053=VECTOR('',#7205,2.05475);
#2054=VECTOR('',#7210,2.05475);
#2055=VECTOR('',#7213,2.05475);
#2056=VECTOR('',#7216,2.05475);
#2057=VECTOR('',#7219,2.05475);
#2058=VECTOR('',#7222,2.05475);
#2059=VECTOR('',#7225,2.05475);
#2060=VECTOR('',#7228,2.05475);
#2061=VECTOR('',#7231,2.05475);
#2062=VECTOR('',#7234,2.05475);
#2063=VECTOR('',#7237,2.05475);
#2064=VECTOR('',#7240,2.05475);
#2065=VECTOR('',#7245,2.05475);
#2066=VECTOR('',#7250,2.05475);
#2067=VECTOR('',#7253,2.05475);
#2068=VECTOR('',#7256,2.05475);
#2069=VECTOR('',#7259,2.05475);
#2070=VECTOR('',#7262,2.05475);
#2071=VECTOR('',#7265,2.05475);
#2072=VECTOR('',#7268,2.05475);
#2073=VECTOR('',#7271,2.05475);
#2074=VECTOR('',#7274,2.05475);
#2075=VECTOR('',#7277,2.05475);
#2076=VECTOR('',#7280,2.05475);
#2077=VECTOR('',#7285,10.);
#2078=VECTOR('',#7288,10.);
#2079=VECTOR('',#7293,10.);
#2080=VECTOR('',#7296,10.);
#2081=VECTOR('',#7299,10.);
#2082=VECTOR('',#7302,10.);
#2083=VECTOR('',#7305,10.);
#2084=VECTOR('',#7308,10.);
#2085=VECTOR('',#7311,10.);
#2086=VECTOR('',#7312,10.);
#2087=VECTOR('',#7317,10.);
#2088=VECTOR('',#7318,10.);
#2089=VECTOR('',#7321,10.);
#2090=VECTOR('',#7322,10.);
#2091=VECTOR('',#7323,10.);
#2092=VECTOR('',#7324,10.);
#2093=VECTOR('',#7325,10.);
#2094=VECTOR('',#7328,10.);
#2095=VECTOR('',#7329,10.);
#2096=VECTOR('',#7330,10.);
#2097=VECTOR('',#7333,10.);
#2098=VECTOR('',#7334,10.);
#2099=VECTOR('',#7337,10.);
#2100=VECTOR('',#7340,10.);
#2101=VECTOR('',#7341,10.);
#2102=VECTOR('',#7342,10.);
#2103=VECTOR('',#7347,10.);
#2104=VECTOR('',#7348,10.);
#2105=VECTOR('',#7353,10.);
#2106=VECTOR('',#7360,10.);
#2107=VECTOR('',#7365,10.);
#2108=VECTOR('',#7368,10.);
#2109=VECTOR('',#7371,10.);
#2110=VECTOR('',#7372,10.);
#2111=VECTOR('',#7373,10.);
#2112=VECTOR('',#7376,10.);
#2113=VECTOR('',#7377,10.);
#2114=VECTOR('',#7396,3.5);
#2115=VECTOR('',#7401,3.5);
#2116=VECTOR('',#7408,10.);
#2117=VECTOR('',#7409,10.);
#2118=VECTOR('',#7410,10.);
#2119=VECTOR('',#7411,10.);
#2120=VECTOR('',#7412,10.);
#2121=VECTOR('',#7413,10.);
#2122=VECTOR('',#7414,10.);
#2123=VECTOR('',#7415,10.);
#2124=VECTOR('',#7416,10.);
#2125=VECTOR('',#7417,10.);
#2126=VECTOR('',#7418,10.);
#2127=VECTOR('',#7419,10.);
#2128=VECTOR('',#7420,10.);
#2129=VECTOR('',#7421,10.);
#2130=VECTOR('',#7422,10.);
#2131=VECTOR('',#7423,10.);
#2132=VECTOR('',#7424,10.);
#2133=VECTOR('',#7425,10.);
#2134=VECTOR('',#7434,10.);
#2135=VECTOR('',#7435,10.);
#2136=VECTOR('',#7436,10.);
#2137=VECTOR('',#7437,10.);
#2138=VECTOR('',#7438,10.);
#2139=VECTOR('',#7439,10.);
#2140=VECTOR('',#7440,10.);
#2141=VECTOR('',#7441,10.);
#2142=VECTOR('',#7442,10.);
#2143=VECTOR('',#7443,10.);
#2144=VECTOR('',#7444,10.);
#2145=VECTOR('',#7445,10.);
#2146=VECTOR('',#7446,10.);
#2147=VECTOR('',#7447,10.);
#2148=VECTOR('',#7448,10.);
#2149=VECTOR('',#7455,10.);
#2150=VECTOR('',#7468,10.);
#2151=VECTOR('',#7469,10.);
#2152=VECTOR('',#7472,10.);
#2153=VECTOR('',#7475,10.);
#2154=VECTOR('',#7480,10.);
#2155=VECTOR('',#7481,10.);
#2156=VECTOR('',#7484,10.);
#2157=VECTOR('',#7487,10.);
#2158=VECTOR('',#7492,10.);
#2159=VECTOR('',#7493,10.);
#2160=VECTOR('',#7496,10.);
#2161=VECTOR('',#7499,10.);
#2162=VECTOR('',#7504,10.);
#2163=VECTOR('',#7505,10.);
#2164=VECTOR('',#7506,10.);
#2165=VECTOR('',#7507,10.);
#2166=VECTOR('',#7508,10.);
#2167=VECTOR('',#7509,10.);
#2168=VECTOR('',#7510,10.);
#2169=VECTOR('',#7511,10.);
#2170=VECTOR('',#7514,10.);
#2171=VECTOR('',#7519,10.);
#2172=VECTOR('',#7522,10.);
#2173=VECTOR('',#7525,10.);
#2174=VECTOR('',#7526,10.);
#2175=VECTOR('',#7529,10.);
#2176=VECTOR('',#7532,10.);
#2177=VECTOR('',#7537,10.);
#2178=VECTOR('',#7540,10.);
#2441=VERTEX_POINT('',#8356);
#2442=VERTEX_POINT('',#8357);
#2443=VERTEX_POINT('',#8359);
#2444=VERTEX_POINT('',#8373);
#2445=VERTEX_POINT('',#8395);
#2446=VERTEX_POINT('',#8396);
#2447=VERTEX_POINT('',#8443);
#2448=VERTEX_POINT('',#8444);
#2449=VERTEX_POINT('',#8491);
#2450=VERTEX_POINT('',#8492);
#2451=VERTEX_POINT('',#8542);
#2452=VERTEX_POINT('',#8543);
#2453=VERTEX_POINT('',#8590);
#2454=VERTEX_POINT('',#8591);
#2455=VERTEX_POINT('',#8638);
#2456=VERTEX_POINT('',#8639);
#2457=VERTEX_POINT('',#8689);
#2458=VERTEX_POINT('',#8690);
#2459=VERTEX_POINT('',#8740);
#2460=VERTEX_POINT('',#8741);
#2461=VERTEX_POINT('',#8788);
#2462=VERTEX_POINT('',#8789);
#2463=VERTEX_POINT('',#8839);
#2464=VERTEX_POINT('',#8840);
#2465=VERTEX_POINT('',#8842);
#2466=VERTEX_POINT('',#8856);
#2467=VERTEX_POINT('',#8878);
#2468=VERTEX_POINT('',#8879);
#2469=VERTEX_POINT('',#8881);
#2470=VERTEX_POINT('',#8895);
#2471=VERTEX_POINT('',#8917);
#2472=VERTEX_POINT('',#8918);
#2473=VERTEX_POINT('',#8965);
#2474=VERTEX_POINT('',#8966);
#2475=VERTEX_POINT('',#9013);
#2476=VERTEX_POINT('',#9014);
#2477=VERTEX_POINT('',#9064);
#2478=VERTEX_POINT('',#9065);
#2479=VERTEX_POINT('',#9112);
#2480=VERTEX_POINT('',#9113);
#2481=VERTEX_POINT('',#9160);
#2482=VERTEX_POINT('',#9161);
#2483=VERTEX_POINT('',#9211);
#2484=VERTEX_POINT('',#9212);
#2485=VERTEX_POINT('',#9262);
#2486=VERTEX_POINT('',#9263);
#2487=VERTEX_POINT('',#9310);
#2488=VERTEX_POINT('',#9311);
#2489=VERTEX_POINT('',#9361);
#2490=VERTEX_POINT('',#9362);
#2491=VERTEX_POINT('',#9364);
#2492=VERTEX_POINT('',#9378);
#2493=VERTEX_POINT('',#9400);
#2494=VERTEX_POINT('',#9401);
#2495=VERTEX_POINT('',#9403);
#2496=VERTEX_POINT('',#9417);
#2497=VERTEX_POINT('',#9439);
#2498=VERTEX_POINT('',#9440);
#2499=VERTEX_POINT('',#9487);
#2500=VERTEX_POINT('',#9488);
#2501=VERTEX_POINT('',#9535);
#2502=VERTEX_POINT('',#9536);
#2503=VERTEX_POINT('',#9586);
#2504=VERTEX_POINT('',#9587);
#2505=VERTEX_POINT('',#9634);
#2506=VERTEX_POINT('',#9635);
#2507=VERTEX_POINT('',#9682);
#2508=VERTEX_POINT('',#9683);
#2509=VERTEX_POINT('',#9733);
#2510=VERTEX_POINT('',#9734);
#2511=VERTEX_POINT('',#9784);
#2512=VERTEX_POINT('',#9785);
#2513=VERTEX_POINT('',#9832);
#2514=VERTEX_POINT('',#9833);
#2515=VERTEX_POINT('',#9883);
#2516=VERTEX_POINT('',#9884);
#2517=VERTEX_POINT('',#9886);
#2518=VERTEX_POINT('',#9900);
#2519=VERTEX_POINT('',#9902);
#2520=VERTEX_POINT('',#9924);
#2521=VERTEX_POINT('',#9925);
#2522=VERTEX_POINT('',#9927);
#2523=VERTEX_POINT('',#9941);
#2524=VERTEX_POINT('',#9963);
#2525=VERTEX_POINT('',#9964);
#2526=VERTEX_POINT('',#10011);
#2527=VERTEX_POINT('',#10012);
#2528=VERTEX_POINT('',#10059);
#2529=VERTEX_POINT('',#10060);
#2530=VERTEX_POINT('',#10110);
#2531=VERTEX_POINT('',#10111);
#2532=VERTEX_POINT('',#10158);
#2533=VERTEX_POINT('',#10159);
#2534=VERTEX_POINT('',#10206);
#2535=VERTEX_POINT('',#10207);
#2536=VERTEX_POINT('',#10257);
#2537=VERTEX_POINT('',#10258);
#2538=VERTEX_POINT('',#10308);
#2539=VERTEX_POINT('',#10309);
#2540=VERTEX_POINT('',#10356);
#2541=VERTEX_POINT('',#10357);
#2542=VERTEX_POINT('',#10407);
#2543=VERTEX_POINT('',#10408);
#2544=VERTEX_POINT('',#10410);
#2545=VERTEX_POINT('',#10424);
#2546=VERTEX_POINT('',#10426);
#2547=VERTEX_POINT('',#10448);
#2548=VERTEX_POINT('',#10449);
#2549=VERTEX_POINT('',#10451);
#2550=VERTEX_POINT('',#10456);
#2551=VERTEX_POINT('',#10464);
#2552=VERTEX_POINT('',#10465);
#2553=VERTEX_POINT('',#10489);
#2554=VERTEX_POINT('',#10490);
#2555=VERTEX_POINT('',#10514);
#2556=VERTEX_POINT('',#10515);
#2557=VERTEX_POINT('',#10538);
#2558=VERTEX_POINT('',#10539);
#2559=VERTEX_POINT('',#10563);
#2560=VERTEX_POINT('',#10564);
#2561=VERTEX_POINT('',#10587);
#2562=VERTEX_POINT('',#10588);
#2563=VERTEX_POINT('',#10612);
#2564=VERTEX_POINT('',#10613);
#2565=VERTEX_POINT('',#10636);
#2566=VERTEX_POINT('',#10637);
#2567=VERTEX_POINT('',#10661);
#2568=VERTEX_POINT('',#10662);
#2569=VERTEX_POINT('',#10686);
#2570=VERTEX_POINT('',#10687);
#2571=VERTEX_POINT('',#10710);
#2572=VERTEX_POINT('',#10711);
#2573=VERTEX_POINT('',#10713);
#2574=VERTEX_POINT('',#10719);
#2575=VERTEX_POINT('',#10727);
#2576=VERTEX_POINT('',#10728);
#2577=VERTEX_POINT('',#10730);
#2578=VERTEX_POINT('',#10735);
#2579=VERTEX_POINT('',#10743);
#2580=VERTEX_POINT('',#10744);
#2581=VERTEX_POINT('',#10768);
#2582=VERTEX_POINT('',#10769);
#2583=VERTEX_POINT('',#10793);
#2584=VERTEX_POINT('',#10794);
#2585=VERTEX_POINT('',#10817);
#2586=VERTEX_POINT('',#10818);
#2587=VERTEX_POINT('',#10842);
#2588=VERTEX_POINT('',#10843);
#2589=VERTEX_POINT('',#10866);
#2590=VERTEX_POINT('',#10867);
#2591=VERTEX_POINT('',#10891);
#2592=VERTEX_POINT('',#10892);
#2593=VERTEX_POINT('',#10915);
#2594=VERTEX_POINT('',#10916);
#2595=VERTEX_POINT('',#10940);
#2596=VERTEX_POINT('',#10941);
#2597=VERTEX_POINT('',#10965);
#2598=VERTEX_POINT('',#10966);
#2599=VERTEX_POINT('',#10989);
#2600=VERTEX_POINT('',#10990);
#2601=VERTEX_POINT('',#10992);
#2602=VERTEX_POINT('',#10998);
#2603=VERTEX_POINT('',#11006);
#2604=VERTEX_POINT('',#11007);
#2605=VERTEX_POINT('',#11009);
#2606=VERTEX_POINT('',#11014);
#2607=VERTEX_POINT('',#11022);
#2608=VERTEX_POINT('',#11023);
#2609=VERTEX_POINT('',#11047);
#2610=VERTEX_POINT('',#11048);
#2611=VERTEX_POINT('',#11072);
#2612=VERTEX_POINT('',#11073);
#2613=VERTEX_POINT('',#11096);
#2614=VERTEX_POINT('',#11097);
#2615=VERTEX_POINT('',#11121);
#2616=VERTEX_POINT('',#11122);
#2617=VERTEX_POINT('',#11145);
#2618=VERTEX_POINT('',#11146);
#2619=VERTEX_POINT('',#11170);
#2620=VERTEX_POINT('',#11171);
#2621=VERTEX_POINT('',#11194);
#2622=VERTEX_POINT('',#11195);
#2623=VERTEX_POINT('',#11219);
#2624=VERTEX_POINT('',#11220);
#2625=VERTEX_POINT('',#11244);
#2626=VERTEX_POINT('',#11245);
#2627=VERTEX_POINT('',#11268);
#2628=VERTEX_POINT('',#11269);
#2629=VERTEX_POINT('',#11271);
#2630=VERTEX_POINT('',#11277);
#2631=VERTEX_POINT('',#11285);
#2632=VERTEX_POINT('',#11286);
#2633=VERTEX_POINT('',#11288);
#2634=VERTEX_POINT('',#11293);
#2635=VERTEX_POINT('',#11301);
#2636=VERTEX_POINT('',#11302);
#2637=VERTEX_POINT('',#11326);
#2638=VERTEX_POINT('',#11327);
#2639=VERTEX_POINT('',#11351);
#2640=VERTEX_POINT('',#11352);
#2641=VERTEX_POINT('',#11375);
#2642=VERTEX_POINT('',#11376);
#2643=VERTEX_POINT('',#11400);
#2644=VERTEX_POINT('',#11401);
#2645=VERTEX_POINT('',#11424);
#2646=VERTEX_POINT('',#11425);
#2647=VERTEX_POINT('',#11449);
#2648=VERTEX_POINT('',#11450);
#2649=VERTEX_POINT('',#11473);
#2650=VERTEX_POINT('',#11474);
#2651=VERTEX_POINT('',#11498);
#2652=VERTEX_POINT('',#11499);
#2653=VERTEX_POINT('',#11523);
#2654=VERTEX_POINT('',#11524);
#2655=VERTEX_POINT('',#11547);
#2656=VERTEX_POINT('',#11548);
#2657=VERTEX_POINT('',#11550);
#2658=VERTEX_POINT('',#11556);
#2659=VERTEX_POINT('',#11564);
#2660=VERTEX_POINT('',#11565);
#2661=VERTEX_POINT('',#11567);
#2662=VERTEX_POINT('',#11569);
#2663=VERTEX_POINT('',#11573);
#2664=VERTEX_POINT('',#11575);
#2665=VERTEX_POINT('',#11579);
#2666=VERTEX_POINT('',#11581);
#2667=VERTEX_POINT('',#11585);
#2668=VERTEX_POINT('',#11587);
#2669=VERTEX_POINT('',#11591);
#2670=VERTEX_POINT('',#11593);
#2671=VERTEX_POINT('',#11600);
#2672=VERTEX_POINT('',#11602);
#2673=VERTEX_POINT('',#11604);
#2674=VERTEX_POINT('',#11606);
#2675=VERTEX_POINT('',#11610);
#2676=VERTEX_POINT('',#11615);
#2677=VERTEX_POINT('',#11619);
#2678=VERTEX_POINT('',#11620);
#2679=VERTEX_POINT('',#11622);
#2680=VERTEX_POINT('',#11624);
#2681=VERTEX_POINT('',#11626);
#2682=VERTEX_POINT('',#11628);
#2683=VERTEX_POINT('',#11630);
#2684=VERTEX_POINT('',#11632);
#2685=VERTEX_POINT('',#11634);
#2686=VERTEX_POINT('',#11638);
#2687=VERTEX_POINT('',#11659);
#2688=VERTEX_POINT('',#11661);
#2689=VERTEX_POINT('',#11665);
#2690=VERTEX_POINT('',#11687);
#2691=VERTEX_POINT('',#11693);
#2692=VERTEX_POINT('',#11695);
#2693=VERTEX_POINT('',#11699);
#2694=VERTEX_POINT('',#11703);
#2695=VERTEX_POINT('',#11705);
#2696=VERTEX_POINT('',#11709);
#2697=VERTEX_POINT('',#11711);
#2698=VERTEX_POINT('',#11715);
#2699=VERTEX_POINT('',#11719);
#2700=VERTEX_POINT('',#12746);
#2701=VERTEX_POINT('',#12747);
#2702=VERTEX_POINT('',#12749);
#2703=VERTEX_POINT('',#12751);
#2704=VERTEX_POINT('',#12753);
#2705=VERTEX_POINT('',#12755);
#2706=VERTEX_POINT('',#12758);
#2707=VERTEX_POINT('',#12759);
#2708=VERTEX_POINT('',#12761);
#2709=VERTEX_POINT('',#12763);
#2710=VERTEX_POINT('',#12766);
#2711=VERTEX_POINT('',#12767);
#2712=VERTEX_POINT('',#12769);
#2713=VERTEX_POINT('',#12771);
#2714=VERTEX_POINT('',#12774);
#2715=VERTEX_POINT('',#12775);
#2716=VERTEX_POINT('',#12777);
#2717=VERTEX_POINT('',#12779);
#2718=VERTEX_POINT('',#15862);
#2719=VERTEX_POINT('',#15864);
#2720=VERTEX_POINT('',#15867);
#2721=VERTEX_POINT('',#15868);
#2722=VERTEX_POINT('',#15870);
#2723=VERTEX_POINT('',#15872);
#2724=VERTEX_POINT('',#15875);
#2725=VERTEX_POINT('',#15876);
#2726=VERTEX_POINT('',#15878);
#2727=VERTEX_POINT('',#15880);
#2728=VERTEX_POINT('',#15883);
#2729=VERTEX_POINT('',#15884);
#2730=VERTEX_POINT('',#15886);
#2731=VERTEX_POINT('',#15888);
#2732=VERTEX_POINT('',#15925);
#2733=VERTEX_POINT('',#15928);
#2734=VERTEX_POINT('',#15929);
#2735=VERTEX_POINT('',#15931);
#2736=VERTEX_POINT('',#15933);
#2737=VERTEX_POINT('',#15935);
#2738=VERTEX_POINT('',#15937);
#3047=EDGE_CURVE('',#2441,#2442,#1529,.T.);
#3048=EDGE_CURVE('',#2442,#2443,#1162,.T.);
#3049=EDGE_CURVE('',#2444,#2443,#1067,.F.);
#3050=EDGE_CURVE('',#2444,#2441,#1163,.T.);
#3051=EDGE_CURVE('',#2445,#2446,#1530,.T.);
#3052=EDGE_CURVE('',#2446,#2442,#1164,.T.);
#3053=EDGE_CURVE('',#2441,#2445,#1165,.T.);
#3054=EDGE_CURVE('',#2447,#2448,#1531,.T.);
#3055=EDGE_CURVE('',#2448,#2446,#1166,.T.);
#3056=EDGE_CURVE('',#2445,#2447,#1167,.T.);
#3057=EDGE_CURVE('',#2449,#2450,#1532,.T.);
#3058=EDGE_CURVE('',#2450,#2448,#1168,.T.);
#3059=EDGE_CURVE('',#2447,#2449,#1169,.T.);
#3060=EDGE_CURVE('',#2451,#2452,#1533,.T.);
#3061=EDGE_CURVE('',#2452,#2450,#1170,.T.);
#3062=EDGE_CURVE('',#2449,#2451,#1171,.T.);
#3063=EDGE_CURVE('',#2453,#2454,#1534,.T.);
#3064=EDGE_CURVE('',#2454,#2452,#1172,.T.);
#3065=EDGE_CURVE('',#2451,#2453,#1173,.T.);
#3066=EDGE_CURVE('',#2455,#2456,#1535,.T.);
#3067=EDGE_CURVE('',#2456,#2454,#1174,.T.);
#3068=EDGE_CURVE('',#2453,#2455,#1175,.T.);
#3069=EDGE_CURVE('',#2457,#2458,#1536,.T.);
#3070=EDGE_CURVE('',#2458,#2456,#1176,.T.);
#3071=EDGE_CURVE('',#2455,#2457,#1177,.T.);
#3072=EDGE_CURVE('',#2459,#2460,#1537,.T.);
#3073=EDGE_CURVE('',#2460,#2458,#1178,.T.);
#3074=EDGE_CURVE('',#2457,#2459,#1179,.T.);
#3075=EDGE_CURVE('',#2461,#2462,#1538,.T.);
#3076=EDGE_CURVE('',#2462,#2460,#1180,.T.);
#3077=EDGE_CURVE('',#2459,#2461,#1181,.T.);
#3078=EDGE_CURVE('',#2463,#2464,#1539,.T.);
#3079=EDGE_CURVE('',#2463,#2465,#1182,.T.);
#3080=EDGE_CURVE('',#2465,#2466,#1068,.F.);
#3081=EDGE_CURVE('',#2466,#2464,#1183,.T.);
#3082=EDGE_CURVE('',#2467,#2468,#1540,.T.);
#3083=EDGE_CURVE('',#2468,#2469,#1184,.T.);
#3084=EDGE_CURVE('',#2470,#2469,#1069,.F.);
#3085=EDGE_CURVE('',#2470,#2467,#1185,.T.);
#3086=EDGE_CURVE('',#2471,#2472,#1541,.T.);
#3087=EDGE_CURVE('',#2472,#2468,#1186,.T.);
#3088=EDGE_CURVE('',#2467,#2471,#1187,.T.);
#3089=EDGE_CURVE('',#2473,#2474,#1542,.T.);
#3090=EDGE_CURVE('',#2474,#2472,#1188,.T.);
#3091=EDGE_CURVE('',#2471,#2473,#1189,.T.);
#3092=EDGE_CURVE('',#2475,#2476,#1543,.T.);
#3093=EDGE_CURVE('',#2476,#2474,#1190,.T.);
#3094=EDGE_CURVE('',#2473,#2475,#1191,.T.);
#3095=EDGE_CURVE('',#2477,#2478,#1544,.T.);
#3096=EDGE_CURVE('',#2478,#2476,#1192,.T.);
#3097=EDGE_CURVE('',#2475,#2477,#1193,.T.);
#3098=EDGE_CURVE('',#2479,#2480,#1545,.T.);
#3099=EDGE_CURVE('',#2480,#2478,#1194,.T.);
#3100=EDGE_CURVE('',#2477,#2479,#1195,.T.);
#3101=EDGE_CURVE('',#2481,#2482,#1546,.T.);
#3102=EDGE_CURVE('',#2482,#2480,#1196,.T.);
#3103=EDGE_CURVE('',#2479,#2481,#1197,.T.);
#3104=EDGE_CURVE('',#2483,#2484,#1547,.T.);
#3105=EDGE_CURVE('',#2484,#2482,#1198,.T.);
#3106=EDGE_CURVE('',#2481,#2483,#1199,.T.);
#3107=EDGE_CURVE('',#2485,#2486,#1548,.T.);
#3108=EDGE_CURVE('',#2486,#2484,#1200,.T.);
#3109=EDGE_CURVE('',#2483,#2485,#1201,.T.);
#3110=EDGE_CURVE('',#2487,#2488,#1549,.T.);
#3111=EDGE_CURVE('',#2488,#2486,#1202,.T.);
#3112=EDGE_CURVE('',#2485,#2487,#1203,.T.);
#3113=EDGE_CURVE('',#2489,#2490,#1550,.T.);
#3114=EDGE_CURVE('',#2489,#2491,#1204,.T.);
#3115=EDGE_CURVE('',#2491,#2492,#1070,.F.);
#3116=EDGE_CURVE('',#2492,#2490,#1205,.T.);
#3117=EDGE_CURVE('',#2493,#2494,#1551,.T.);
#3118=EDGE_CURVE('',#2494,#2495,#1206,.T.);
#3119=EDGE_CURVE('',#2496,#2495,#1071,.F.);
#3120=EDGE_CURVE('',#2496,#2493,#1207,.T.);
#3121=EDGE_CURVE('',#2497,#2498,#1552,.T.);
#3122=EDGE_CURVE('',#2498,#2494,#1208,.T.);
#3123=EDGE_CURVE('',#2493,#2497,#1209,.T.);
#3124=EDGE_CURVE('',#2499,#2500,#1553,.T.);
#3125=EDGE_CURVE('',#2500,#2498,#1210,.T.);
#3126=EDGE_CURVE('',#2497,#2499,#1211,.T.);
#3127=EDGE_CURVE('',#2501,#2502,#1554,.T.);
#3128=EDGE_CURVE('',#2502,#2500,#1212,.T.);
#3129=EDGE_CURVE('',#2499,#2501,#1213,.T.);
#3130=EDGE_CURVE('',#2503,#2504,#1555,.T.);
#3131=EDGE_CURVE('',#2504,#2502,#1214,.T.);
#3132=EDGE_CURVE('',#2501,#2503,#1215,.T.);
#3133=EDGE_CURVE('',#2505,#2506,#1556,.T.);
#3134=EDGE_CURVE('',#2506,#2504,#1216,.T.);
#3135=EDGE_CURVE('',#2503,#2505,#1217,.T.);
#3136=EDGE_CURVE('',#2507,#2508,#1557,.T.);
#3137=EDGE_CURVE('',#2508,#2506,#1218,.T.);
#3138=EDGE_CURVE('',#2505,#2507,#1219,.T.);
#3139=EDGE_CURVE('',#2509,#2510,#1558,.T.);
#3140=EDGE_CURVE('',#2510,#2508,#1220,.T.);
#3141=EDGE_CURVE('',#2507,#2509,#1221,.T.);
#3142=EDGE_CURVE('',#2511,#2512,#1559,.T.);
#3143=EDGE_CURVE('',#2512,#2510,#1222,.T.);
#3144=EDGE_CURVE('',#2509,#2511,#1223,.T.);
#3145=EDGE_CURVE('',#2513,#2514,#1560,.T.);
#3146=EDGE_CURVE('',#2514,#2512,#1224,.T.);
#3147=EDGE_CURVE('',#2511,#2513,#1225,.T.);
#3148=EDGE_CURVE('',#2515,#2516,#1561,.T.);
#3149=EDGE_CURVE('',#2515,#2517,#1226,.T.);
#3150=EDGE_CURVE('',#2518,#2517,#1072,.T.);
#3151=EDGE_CURVE('',#2518,#2519,#1073,.F.);
#3152=EDGE_CURVE('',#2519,#2516,#1227,.T.);
#3153=EDGE_CURVE('',#2520,#2521,#1562,.T.);
#3154=EDGE_CURVE('',#2521,#2522,#1228,.T.);
#3155=EDGE_CURVE('',#2523,#2522,#1074,.F.);
#3156=EDGE_CURVE('',#2523,#2520,#1229,.T.);
#3157=EDGE_CURVE('',#2524,#2525,#1563,.T.);
#3158=EDGE_CURVE('',#2525,#2521,#1230,.T.);
#3159=EDGE_CURVE('',#2520,#2524,#1231,.T.);
#3160=EDGE_CURVE('',#2526,#2527,#1564,.T.);
#3161=EDGE_CURVE('',#2527,#2525,#1232,.T.);
#3162=EDGE_CURVE('',#2524,#2526,#1233,.T.);
#3163=EDGE_CURVE('',#2528,#2529,#1565,.T.);
#3164=EDGE_CURVE('',#2529,#2527,#1234,.T.);
#3165=EDGE_CURVE('',#2526,#2528,#1235,.T.);
#3166=EDGE_CURVE('',#2530,#2531,#1566,.T.);
#3167=EDGE_CURVE('',#2531,#2529,#1236,.T.);
#3168=EDGE_CURVE('',#2528,#2530,#1237,.T.);
#3169=EDGE_CURVE('',#2532,#2533,#1567,.T.);
#3170=EDGE_CURVE('',#2533,#2531,#1238,.T.);
#3171=EDGE_CURVE('',#2530,#2532,#1239,.T.);
#3172=EDGE_CURVE('',#2534,#2535,#1568,.T.);
#3173=EDGE_CURVE('',#2535,#2533,#1240,.T.);
#3174=EDGE_CURVE('',#2532,#2534,#1241,.T.);
#3175=EDGE_CURVE('',#2536,#2537,#1569,.T.);
#3176=EDGE_CURVE('',#2537,#2535,#1242,.T.);
#3177=EDGE_CURVE('',#2534,#2536,#1243,.T.);
#3178=EDGE_CURVE('',#2538,#2539,#1570,.T.);
#3179=EDGE_CURVE('',#2539,#2537,#1244,.T.);
#3180=EDGE_CURVE('',#2536,#2538,#1245,.T.);
#3181=EDGE_CURVE('',#2540,#2541,#1571,.T.);
#3182=EDGE_CURVE('',#2541,#2539,#1246,.T.);
#3183=EDGE_CURVE('',#2538,#2540,#1247,.T.);
#3184=EDGE_CURVE('',#2542,#2543,#1572,.T.);
#3185=EDGE_CURVE('',#2542,#2544,#1248,.T.);
#3186=EDGE_CURVE('',#2544,#2545,#1075,.F.);
#3187=EDGE_CURVE('',#2546,#2545,#1076,.T.);
#3188=EDGE_CURVE('',#2546,#2543,#1249,.T.);
#3189=EDGE_CURVE('',#2547,#2548,#1573,.T.);
#3190=EDGE_CURVE('',#2548,#2549,#1250,.T.);
#3191=EDGE_CURVE('',#2550,#2549,#1077,.T.);
#3192=EDGE_CURVE('',#2547,#2550,#1251,.T.);
#3193=EDGE_CURVE('',#2551,#2552,#1574,.T.);
#3194=EDGE_CURVE('',#2552,#2548,#1252,.T.);
#3195=EDGE_CURVE('',#2551,#2547,#1253,.T.);
#3196=EDGE_CURVE('',#2553,#2554,#1575,.T.);
#3197=EDGE_CURVE('',#2554,#2552,#1254,.T.);
#3198=EDGE_CURVE('',#2553,#2551,#1255,.T.);
#3199=EDGE_CURVE('',#2555,#2556,#1576,.T.);
#3200=EDGE_CURVE('',#2556,#2554,#1256,.T.);
#3201=EDGE_CURVE('',#2555,#2553,#1257,.T.);
#3202=EDGE_CURVE('',#2557,#2558,#1577,.T.);
#3203=EDGE_CURVE('',#2558,#2556,#1258,.T.);
#3204=EDGE_CURVE('',#2557,#2555,#1259,.T.);
#3205=EDGE_CURVE('',#2559,#2560,#1578,.T.);
#3206=EDGE_CURVE('',#2560,#2558,#1260,.T.);
#3207=EDGE_CURVE('',#2559,#2557,#1261,.T.);
#3208=EDGE_CURVE('',#2561,#2562,#1579,.T.);
#3209=EDGE_CURVE('',#2562,#2560,#1262,.T.);
#3210=EDGE_CURVE('',#2561,#2559,#1263,.T.);
#3211=EDGE_CURVE('',#2563,#2564,#1580,.T.);
#3212=EDGE_CURVE('',#2564,#2562,#1264,.T.);
#3213=EDGE_CURVE('',#2563,#2561,#1265,.T.);
#3214=EDGE_CURVE('',#2565,#2566,#1581,.T.);
#3215=EDGE_CURVE('',#2566,#2564,#1266,.T.);
#3216=EDGE_CURVE('',#2565,#2563,#1267,.T.);
#3217=EDGE_CURVE('',#2567,#2568,#1582,.T.);
#3218=EDGE_CURVE('',#2568,#2566,#1268,.T.);
#3219=EDGE_CURVE('',#2567,#2565,#1269,.T.);
#3220=EDGE_CURVE('',#2569,#2570,#1583,.T.);
#3221=EDGE_CURVE('',#2570,#2568,#1270,.T.);
#3222=EDGE_CURVE('',#2569,#2567,#1271,.T.);
#3223=EDGE_CURVE('',#2571,#2572,#1584,.T.);
#3224=EDGE_CURVE('',#2573,#2571,#1272,.T.);
#3225=EDGE_CURVE('',#2574,#2573,#1078,.T.);
#3226=EDGE_CURVE('',#2574,#2572,#1273,.T.);
#3227=EDGE_CURVE('',#2575,#2576,#1585,.T.);
#3228=EDGE_CURVE('',#2576,#2577,#1274,.T.);
#3229=EDGE_CURVE('',#2578,#2577,#1079,.T.);
#3230=EDGE_CURVE('',#2575,#2578,#1275,.T.);
#3231=EDGE_CURVE('',#2579,#2580,#1586,.T.);
#3232=EDGE_CURVE('',#2580,#2576,#1276,.T.);
#3233=EDGE_CURVE('',#2579,#2575,#1277,.T.);
#3234=EDGE_CURVE('',#2581,#2582,#1587,.T.);
#3235=EDGE_CURVE('',#2582,#2580,#1278,.T.);
#3236=EDGE_CURVE('',#2581,#2579,#1279,.T.);
#3237=EDGE_CURVE('',#2583,#2584,#1588,.T.);
#3238=EDGE_CURVE('',#2584,#2582,#1280,.T.);
#3239=EDGE_CURVE('',#2583,#2581,#1281,.T.);
#3240=EDGE_CURVE('',#2585,#2586,#1589,.T.);
#3241=EDGE_CURVE('',#2586,#2584,#1282,.T.);
#3242=EDGE_CURVE('',#2585,#2583,#1283,.T.);
#3243=EDGE_CURVE('',#2587,#2588,#1590,.T.);
#3244=EDGE_CURVE('',#2588,#2586,#1284,.T.);
#3245=EDGE_CURVE('',#2587,#2585,#1285,.T.);
#3246=EDGE_CURVE('',#2589,#2590,#1591,.T.);
#3247=EDGE_CURVE('',#2590,#2588,#1286,.T.);
#3248=EDGE_CURVE('',#2589,#2587,#1287,.T.);
#3249=EDGE_CURVE('',#2591,#2592,#1592,.T.);
#3250=EDGE_CURVE('',#2592,#2590,#1288,.T.);
#3251=EDGE_CURVE('',#2591,#2589,#1289,.T.);
#3252=EDGE_CURVE('',#2593,#2594,#1593,.T.);
#3253=EDGE_CURVE('',#2594,#2592,#1290,.T.);
#3254=EDGE_CURVE('',#2593,#2591,#1291,.T.);
#3255=EDGE_CURVE('',#2595,#2596,#1594,.T.);
#3256=EDGE_CURVE('',#2596,#2594,#1292,.T.);
#3257=EDGE_CURVE('',#2595,#2593,#1293,.T.);
#3258=EDGE_CURVE('',#2597,#2598,#1595,.T.);
#3259=EDGE_CURVE('',#2598,#2596,#1294,.T.);
#3260=EDGE_CURVE('',#2597,#2595,#1295,.T.);
#3261=EDGE_CURVE('',#2599,#2600,#1596,.T.);
#3262=EDGE_CURVE('',#2601,#2599,#1296,.T.);
#3263=EDGE_CURVE('',#2602,#2601,#1080,.T.);
#3264=EDGE_CURVE('',#2602,#2600,#1297,.T.);
#3265=EDGE_CURVE('',#2603,#2604,#1597,.T.);
#3266=EDGE_CURVE('',#2604,#2605,#1298,.T.);
#3267=EDGE_CURVE('',#2606,#2605,#1081,.T.);
#3268=EDGE_CURVE('',#2603,#2606,#1299,.T.);
#3269=EDGE_CURVE('',#2607,#2608,#1598,.T.);
#3270=EDGE_CURVE('',#2608,#2604,#1300,.T.);
#3271=EDGE_CURVE('',#2607,#2603,#1301,.T.);
#3272=EDGE_CURVE('',#2609,#2610,#1599,.T.);
#3273=EDGE_CURVE('',#2610,#2608,#1302,.T.);
#3274=EDGE_CURVE('',#2609,#2607,#1303,.T.);
#3275=EDGE_CURVE('',#2611,#2612,#1600,.T.);
#3276=EDGE_CURVE('',#2612,#2610,#1304,.T.);
#3277=EDGE_CURVE('',#2611,#2609,#1305,.T.);
#3278=EDGE_CURVE('',#2613,#2614,#1601,.T.);
#3279=EDGE_CURVE('',#2614,#2612,#1306,.T.);
#3280=EDGE_CURVE('',#2613,#2611,#1307,.T.);
#3281=EDGE_CURVE('',#2615,#2616,#1602,.T.);
#3282=EDGE_CURVE('',#2616,#2614,#1308,.T.);
#3283=EDGE_CURVE('',#2615,#2613,#1309,.T.);
#3284=EDGE_CURVE('',#2617,#2618,#1603,.T.);
#3285=EDGE_CURVE('',#2618,#2616,#1310,.T.);
#3286=EDGE_CURVE('',#2617,#2615,#1311,.T.);
#3287=EDGE_CURVE('',#2619,#2620,#1604,.T.);
#3288=EDGE_CURVE('',#2620,#2618,#1312,.T.);
#3289=EDGE_CURVE('',#2619,#2617,#1313,.T.);
#3290=EDGE_CURVE('',#2621,#2622,#1605,.T.);
#3291=EDGE_CURVE('',#2622,#2620,#1314,.T.);
#3292=EDGE_CURVE('',#2621,#2619,#1315,.T.);
#3293=EDGE_CURVE('',#2623,#2624,#1606,.T.);
#3294=EDGE_CURVE('',#2624,#2622,#1316,.T.);
#3295=EDGE_CURVE('',#2623,#2621,#1317,.T.);
#3296=EDGE_CURVE('',#2625,#2626,#1607,.T.);
#3297=EDGE_CURVE('',#2626,#2624,#1318,.T.);
#3298=EDGE_CURVE('',#2625,#2623,#1319,.T.);
#3299=EDGE_CURVE('',#2627,#2628,#1608,.T.);
#3300=EDGE_CURVE('',#2629,#2627,#1320,.T.);
#3301=EDGE_CURVE('',#2630,#2629,#1082,.T.);
#3302=EDGE_CURVE('',#2630,#2628,#1321,.T.);
#3303=EDGE_CURVE('',#2631,#2632,#1609,.T.);
#3304=EDGE_CURVE('',#2632,#2633,#1322,.T.);
#3305=EDGE_CURVE('',#2634,#2633,#1083,.T.);
#3306=EDGE_CURVE('',#2631,#2634,#1323,.T.);
#3307=EDGE_CURVE('',#2635,#2636,#1610,.T.);
#3308=EDGE_CURVE('',#2636,#2632,#1324,.T.);
#3309=EDGE_CURVE('',#2635,#2631,#1325,.T.);
#3310=EDGE_CURVE('',#2637,#2638,#1611,.T.);
#3311=EDGE_CURVE('',#2638,#2636,#1326,.T.);
#3312=EDGE_CURVE('',#2637,#2635,#1327,.T.);
#3313=EDGE_CURVE('',#2639,#2640,#1612,.T.);
#3314=EDGE_CURVE('',#2640,#2638,#1328,.T.);
#3315=EDGE_CURVE('',#2639,#2637,#1329,.T.);
#3316=EDGE_CURVE('',#2641,#2642,#1613,.T.);
#3317=EDGE_CURVE('',#2642,#2640,#1330,.T.);
#3318=EDGE_CURVE('',#2641,#2639,#1331,.T.);
#3319=EDGE_CURVE('',#2643,#2644,#1614,.T.);
#3320=EDGE_CURVE('',#2644,#2642,#1332,.T.);
#3321=EDGE_CURVE('',#2643,#2641,#1333,.T.);
#3322=EDGE_CURVE('',#2645,#2646,#1615,.T.);
#3323=EDGE_CURVE('',#2646,#2644,#1334,.T.);
#3324=EDGE_CURVE('',#2645,#2643,#1335,.T.);
#3325=EDGE_CURVE('',#2647,#2648,#1616,.T.);
#3326=EDGE_CURVE('',#2648,#2646,#1336,.T.);
#3327=EDGE_CURVE('',#2647,#2645,#1337,.T.);
#3328=EDGE_CURVE('',#2649,#2650,#1617,.T.);
#3329=EDGE_CURVE('',#2650,#2648,#1338,.T.);
#3330=EDGE_CURVE('',#2649,#2647,#1339,.T.);
#3331=EDGE_CURVE('',#2651,#2652,#1618,.T.);
#3332=EDGE_CURVE('',#2652,#2650,#1340,.T.);
#3333=EDGE_CURVE('',#2651,#2649,#1341,.T.);
#3334=EDGE_CURVE('',#2653,#2654,#1619,.T.);
#3335=EDGE_CURVE('',#2654,#2652,#1342,.T.);
#3336=EDGE_CURVE('',#2653,#2651,#1343,.T.);
#3337=EDGE_CURVE('',#2655,#2656,#1620,.T.);
#3338=EDGE_CURVE('',#2657,#2655,#1344,.T.);
#3339=EDGE_CURVE('',#2658,#2657,#1084,.T.);
#3340=EDGE_CURVE('',#2658,#2656,#1345,.T.);
#3341=EDGE_CURVE('',#2659,#2660,#1621,.T.);
#3342=EDGE_CURVE('',#2660,#2661,#313,.T.);
#3343=EDGE_CURVE('',#2661,#2662,#1622,.T.);
#3344=EDGE_CURVE('',#2659,#2662,#314,.T.);
#3345=EDGE_CURVE('',#2660,#2663,#1623,.T.);
#3346=EDGE_CURVE('',#2663,#2664,#315,.T.);
#3347=EDGE_CURVE('',#2664,#2661,#1624,.T.);
#3348=EDGE_CURVE('',#2663,#2665,#1625,.T.);
#3349=EDGE_CURVE('',#2665,#2666,#316,.T.);
#3350=EDGE_CURVE('',#2666,#2664,#1626,.T.);
#3351=EDGE_CURVE('',#2665,#2667,#1627,.T.);
#3352=EDGE_CURVE('',#2667,#2668,#317,.T.);
#3353=EDGE_CURVE('',#2668,#2666,#1628,.T.);
#3354=EDGE_CURVE('',#2669,#2668,#1629,.T.);
#3355=EDGE_CURVE('',#2667,#2670,#1630,.T.);
#3356=EDGE_CURVE('',#2670,#2669,#318,.T.);
#3357=EDGE_CURVE('',#2662,#2669,#1631,.T.);
#3358=EDGE_CURVE('',#2670,#2659,#1632,.T.);
#3359=EDGE_CURVE('',#2671,#2669,#1633,.T.);
#3360=EDGE_CURVE('',#2672,#2671,#1634,.T.);
#3361=EDGE_CURVE('',#2673,#2672,#1635,.T.);
#3362=EDGE_CURVE('',#2674,#2673,#1636,.T.);
#3363=EDGE_CURVE('',#2674,#2668,#1637,.T.);
#3364=EDGE_CURVE('',#2675,#2662,#1638,.T.);
#3365=EDGE_CURVE('',#2545,#2675,#1639,.T.);
#3366=EDGE_CURVE('',#2671,#2545,#1640,.T.);
#3367=EDGE_CURVE('',#2676,#2661,#1641,.T.);
#3368=EDGE_CURVE('',#2675,#2676,#1642,.T.);
#3369=EDGE_CURVE('',#2677,#2678,#1643,.T.);
#3370=EDGE_CURVE('',#2679,#2677,#1085,.T.);
#3371=EDGE_CURVE('',#2680,#2679,#1644,.T.);
#3372=EDGE_CURVE('',#2681,#2680,#1645,.T.);
#3373=EDGE_CURVE('',#2682,#2681,#1646,.T.);
#3374=EDGE_CURVE('',#2683,#2682,#1086,.T.);
#3375=EDGE_CURVE('',#2684,#2683,#1087,.T.);
#3376=EDGE_CURVE('',#2685,#2684,#1647,.T.);
#3377=EDGE_CURVE('',#2678,#2685,#1648,.T.);
#3378=EDGE_CURVE('',#2679,#2686,#1346,.T.);
#3379=EDGE_CURVE('',#2686,#2677,#1347,.T.);
#3380=EDGE_CURVE('',#2678,#2687,#319,.T.);
#3381=EDGE_CURVE('',#2687,#2688,#1649,.T.);
#3382=EDGE_CURVE('',#2680,#2688,#320,.T.);
#3383=EDGE_CURVE('',#2685,#2689,#321,.T.);
#3384=EDGE_CURVE('',#2689,#2687,#1650,.T.);
#3385=EDGE_CURVE('',#2684,#2682,#1348,.T.);
#3386=EDGE_CURVE('',#2681,#2690,#322,.T.);
#3387=EDGE_CURVE('',#2690,#2689,#1651,.T.);
#3388=EDGE_CURVE('',#2688,#2690,#1652,.T.);
#3389=EDGE_CURVE('',#2691,#2688,#1653,.T.);
#3390=EDGE_CURVE('',#2691,#2692,#1654,.T.);
#3391=EDGE_CURVE('',#2692,#2690,#1655,.T.);
#3392=EDGE_CURVE('',#2693,#2687,#1656,.T.);
#3393=EDGE_CURVE('',#2693,#2691,#1657,.T.);
#3394=EDGE_CURVE('',#2686,#2694,#1088,.T.);
#3395=EDGE_CURVE('',#2694,#2695,#1089,.T.);
#3396=EDGE_CURVE('',#2695,#2694,#1090,.T.);
#3397=EDGE_CURVE('',#2683,#2696,#1091,.T.);
#3398=EDGE_CURVE('',#2696,#2697,#1092,.T.);
#3399=EDGE_CURVE('',#2697,#2696,#1093,.T.);
#3400=EDGE_CURVE('',#2695,#2698,#1658,.T.);
#3401=EDGE_CURVE('',#2698,#2698,#1094,.T.);
#3402=EDGE_CURVE('',#2697,#2699,#1659,.T.);
#3403=EDGE_CURVE('',#2699,#2699,#1095,.T.);
#3404=EDGE_CURVE('',#2656,#2654,#1349,.T.);
#3405=EDGE_CURVE('',#2655,#2653,#1350,.T.);
#3406=EDGE_CURVE('',#2633,#2496,#1351,.T.);
#3407=EDGE_CURVE('',#2673,#2658,#1352,.T.);
#3408=EDGE_CURVE('',#2517,#2673,#1353,.T.);
#3409=EDGE_CURVE('',#2513,#2515,#1354,.T.);
#3410=EDGE_CURVE('',#2495,#2634,#1355,.T.);
#3411=EDGE_CURVE('',#2516,#2514,#1356,.T.);
#3412=EDGE_CURVE('',#2657,#2519,#1357,.T.);
#3413=EDGE_CURVE('',#2700,#2701,#1660,.T.);
#3414=EDGE_CURVE('',#2702,#2700,#1661,.T.);
#3415=EDGE_CURVE('',#2703,#2702,#1662,.T.);
#3416=EDGE_CURVE('',#2704,#2703,#1663,.T.);
#3417=EDGE_CURVE('',#2705,#2704,#1664,.T.);
#3418=EDGE_CURVE('',#2701,#2705,#1665,.T.);
#3419=EDGE_CURVE('',#2706,#2707,#1666,.T.);
#3420=EDGE_CURVE('',#2707,#2708,#1667,.T.);
#3421=EDGE_CURVE('',#2708,#2709,#1668,.T.);
#3422=EDGE_CURVE('',#2709,#2706,#1669,.T.);
#3423=EDGE_CURVE('',#2710,#2711,#1670,.T.);
#3424=EDGE_CURVE('',#2711,#2712,#1671,.T.);
#3425=EDGE_CURVE('',#2712,#2713,#1672,.T.);
#3426=EDGE_CURVE('',#2713,#2710,#1673,.T.);
#3427=EDGE_CURVE('',#2714,#2715,#1674,.T.);
#3428=EDGE_CURVE('',#2715,#2716,#1675,.T.);
#3429=EDGE_CURVE('',#2716,#2717,#1676,.T.);
#3430=EDGE_CURVE('',#2717,#2714,#1677,.T.);
#3431=EDGE_CURVE('',#2549,#2523,#1358,.T.);
#3432=EDGE_CURVE('',#2522,#2550,#1359,.T.);
#3433=EDGE_CURVE('',#2577,#2470,#1360,.T.);
#3434=EDGE_CURVE('',#2469,#2578,#1361,.T.);
#3435=EDGE_CURVE('',#2605,#2444,#1362,.T.);
#3436=EDGE_CURVE('',#2443,#2606,#1363,.T.);
#3437=EDGE_CURVE('',#2628,#2626,#1364,.T.);
#3438=EDGE_CURVE('',#2627,#2625,#1365,.T.);
#3439=EDGE_CURVE('',#2465,#2630,#1366,.T.);
#3440=EDGE_CURVE('',#2461,#2463,#1367,.T.);
#3441=EDGE_CURVE('',#2464,#2462,#1368,.T.);
#3442=EDGE_CURVE('',#2629,#2466,#1369,.T.);
#3443=EDGE_CURVE('',#2600,#2598,#1370,.T.);
#3444=EDGE_CURVE('',#2599,#2597,#1371,.T.);
#3445=EDGE_CURVE('',#2491,#2602,#1372,.T.);
#3446=EDGE_CURVE('',#2487,#2489,#1373,.T.);
#3447=EDGE_CURVE('',#2490,#2488,#1374,.T.);
#3448=EDGE_CURVE('',#2601,#2492,#1375,.T.);
#3449=EDGE_CURVE('',#2572,#2570,#1376,.T.);
#3450=EDGE_CURVE('',#2571,#2569,#1377,.T.);
#3451=EDGE_CURVE('',#2544,#2574,#1378,.T.);
#3452=EDGE_CURVE('',#2540,#2542,#1379,.T.);
#3453=EDGE_CURVE('',#2543,#2541,#1380,.T.);
#3454=EDGE_CURVE('',#2672,#2546,#1381,.T.);
#3455=EDGE_CURVE('',#2573,#2672,#1382,.T.);
#3456=EDGE_CURVE('',#2676,#2718,#1678,.T.);
#3457=EDGE_CURVE('',#2718,#2719,#1679,.T.);
#3458=EDGE_CURVE('',#2719,#2518,#1680,.T.);
#3459=EDGE_CURVE('',#2720,#2721,#1681,.T.);
#3460=EDGE_CURVE('',#2721,#2722,#1682,.T.);
#3461=EDGE_CURVE('',#2722,#2723,#1683,.T.);
#3462=EDGE_CURVE('',#2723,#2720,#1684,.T.);
#3463=EDGE_CURVE('',#2724,#2725,#1685,.T.);
#3464=EDGE_CURVE('',#2725,#2726,#1686,.T.);
#3465=EDGE_CURVE('',#2726,#2727,#1687,.T.);
#3466=EDGE_CURVE('',#2727,#2724,#1688,.T.);
#3467=EDGE_CURVE('',#2728,#2729,#1689,.T.);
#3468=EDGE_CURVE('',#2729,#2730,#1690,.T.);
#3469=EDGE_CURVE('',#2730,#2731,#1691,.T.);
#3470=EDGE_CURVE('',#2731,#2728,#1692,.T.);
#3471=EDGE_CURVE('',#2518,#2674,#1693,.T.);
#3472=EDGE_CURVE('',#2728,#2707,#1694,.T.);
#3473=EDGE_CURVE('',#2729,#2706,#1695,.T.);
#3474=EDGE_CURVE('',#2731,#2708,#1696,.T.);
#3475=EDGE_CURVE('',#2730,#2709,#1697,.T.);
#3476=EDGE_CURVE('',#2724,#2711,#1698,.T.);
#3477=EDGE_CURVE('',#2725,#2710,#1699,.T.);
#3478=EDGE_CURVE('',#2727,#2712,#1700,.T.);
#3479=EDGE_CURVE('',#2726,#2713,#1701,.T.);
#3480=EDGE_CURVE('',#2720,#2715,#1702,.T.);
#3481=EDGE_CURVE('',#2721,#2714,#1703,.T.);
#3482=EDGE_CURVE('',#2723,#2716,#1704,.T.);
#3483=EDGE_CURVE('',#2722,#2717,#1705,.T.);
#3484=EDGE_CURVE('',#2692,#2732,#1706,.T.);
#3485=EDGE_CURVE('',#2732,#2693,#1707,.T.);
#3486=EDGE_CURVE('',#2733,#2734,#1708,.T.);
#3487=EDGE_CURVE('',#2735,#2733,#1709,.T.);
#3488=EDGE_CURVE('',#2736,#2735,#1710,.T.);
#3489=EDGE_CURVE('',#2737,#2736,#1711,.T.);
#3490=EDGE_CURVE('',#2738,#2737,#1712,.T.);
#3491=EDGE_CURVE('',#2734,#2738,#1713,.T.);
#3492=EDGE_CURVE('',#2732,#2689,#1714,.T.);
#3493=EDGE_CURVE('',#2718,#2664,#1715,.T.);
#3494=EDGE_CURVE('',#2719,#2666,#1716,.T.);
#3495=EDGE_CURVE('',#2705,#2736,#1717,.T.);
#3496=EDGE_CURVE('',#2704,#2737,#1718,.T.);
#3497=EDGE_CURVE('',#2701,#2735,#1719,.T.);
#3498=EDGE_CURVE('',#2700,#2733,#1720,.T.);
#3499=EDGE_CURVE('',#2702,#2734,#1721,.T.);
#3500=EDGE_CURVE('',#2703,#2738,#1722,.T.);
#3975=ORIENTED_EDGE('',*,*,#3047,.T.);
#3976=ORIENTED_EDGE('',*,*,#3048,.T.);
#3977=ORIENTED_EDGE('',*,*,#3049,.F.);
#3978=ORIENTED_EDGE('',*,*,#3050,.T.);
#3979=ORIENTED_EDGE('',*,*,#3051,.T.);
#3980=ORIENTED_EDGE('',*,*,#3052,.T.);
#3981=ORIENTED_EDGE('',*,*,#3047,.F.);
#3982=ORIENTED_EDGE('',*,*,#3053,.T.);
#3983=ORIENTED_EDGE('',*,*,#3054,.T.);
#3984=ORIENTED_EDGE('',*,*,#3055,.T.);
#3985=ORIENTED_EDGE('',*,*,#3051,.F.);
#3986=ORIENTED_EDGE('',*,*,#3056,.T.);
#3987=ORIENTED_EDGE('',*,*,#3057,.T.);
#3988=ORIENTED_EDGE('',*,*,#3058,.T.);
#3989=ORIENTED_EDGE('',*,*,#3054,.F.);
#3990=ORIENTED_EDGE('',*,*,#3059,.T.);
#3991=ORIENTED_EDGE('',*,*,#3060,.T.);
#3992=ORIENTED_EDGE('',*,*,#3061,.T.);
#3993=ORIENTED_EDGE('',*,*,#3057,.F.);
#3994=ORIENTED_EDGE('',*,*,#3062,.T.);
#3995=ORIENTED_EDGE('',*,*,#3063,.T.);
#3996=ORIENTED_EDGE('',*,*,#3064,.T.);
#3997=ORIENTED_EDGE('',*,*,#3060,.F.);
#3998=ORIENTED_EDGE('',*,*,#3065,.T.);
#3999=ORIENTED_EDGE('',*,*,#3066,.T.);
#4000=ORIENTED_EDGE('',*,*,#3067,.T.);
#4001=ORIENTED_EDGE('',*,*,#3063,.F.);
#4002=ORIENTED_EDGE('',*,*,#3068,.T.);
#4003=ORIENTED_EDGE('',*,*,#3069,.T.);
#4004=ORIENTED_EDGE('',*,*,#3070,.T.);
#4005=ORIENTED_EDGE('',*,*,#3066,.F.);
#4006=ORIENTED_EDGE('',*,*,#3071,.T.);
#4007=ORIENTED_EDGE('',*,*,#3072,.T.);
#4008=ORIENTED_EDGE('',*,*,#3073,.T.);
#4009=ORIENTED_EDGE('',*,*,#3069,.F.);
#4010=ORIENTED_EDGE('',*,*,#3074,.T.);
#4011=ORIENTED_EDGE('',*,*,#3075,.T.);
#4012=ORIENTED_EDGE('',*,*,#3076,.T.);
#4013=ORIENTED_EDGE('',*,*,#3072,.F.);
#4014=ORIENTED_EDGE('',*,*,#3077,.T.);
#4015=ORIENTED_EDGE('',*,*,#3078,.F.);
#4016=ORIENTED_EDGE('',*,*,#3079,.T.);
#4017=ORIENTED_EDGE('',*,*,#3080,.T.);
#4018=ORIENTED_EDGE('',*,*,#3081,.T.);
#4019=ORIENTED_EDGE('',*,*,#3082,.T.);
#4020=ORIENTED_EDGE('',*,*,#3083,.T.);
#4021=ORIENTED_EDGE('',*,*,#3084,.F.);
#4022=ORIENTED_EDGE('',*,*,#3085,.T.);
#4023=ORIENTED_EDGE('',*,*,#3086,.T.);
#4024=ORIENTED_EDGE('',*,*,#3087,.T.);
#4025=ORIENTED_EDGE('',*,*,#3082,.F.);
#4026=ORIENTED_EDGE('',*,*,#3088,.T.);
#4027=ORIENTED_EDGE('',*,*,#3089,.T.);
#4028=ORIENTED_EDGE('',*,*,#3090,.T.);
#4029=ORIENTED_EDGE('',*,*,#3086,.F.);
#4030=ORIENTED_EDGE('',*,*,#3091,.T.);
#4031=ORIENTED_EDGE('',*,*,#3092,.T.);
#4032=ORIENTED_EDGE('',*,*,#3093,.T.);
#4033=ORIENTED_EDGE('',*,*,#3089,.F.);
#4034=ORIENTED_EDGE('',*,*,#3094,.T.);
#4035=ORIENTED_EDGE('',*,*,#3095,.T.);
#4036=ORIENTED_EDGE('',*,*,#3096,.T.);
#4037=ORIENTED_EDGE('',*,*,#3092,.F.);
#4038=ORIENTED_EDGE('',*,*,#3097,.T.);
#4039=ORIENTED_EDGE('',*,*,#3098,.T.);
#4040=ORIENTED_EDGE('',*,*,#3099,.T.);
#4041=ORIENTED_EDGE('',*,*,#3095,.F.);
#4042=ORIENTED_EDGE('',*,*,#3100,.T.);
#4043=ORIENTED_EDGE('',*,*,#3101,.T.);
#4044=ORIENTED_EDGE('',*,*,#3102,.T.);
#4045=ORIENTED_EDGE('',*,*,#3098,.F.);
#4046=ORIENTED_EDGE('',*,*,#3103,.T.);
#4047=ORIENTED_EDGE('',*,*,#3104,.T.);
#4048=ORIENTED_EDGE('',*,*,#3105,.T.);
#4049=ORIENTED_EDGE('',*,*,#3101,.F.);
#4050=ORIENTED_EDGE('',*,*,#3106,.T.);
#4051=ORIENTED_EDGE('',*,*,#3107,.T.);
#4052=ORIENTED_EDGE('',*,*,#3108,.T.);
#4053=ORIENTED_EDGE('',*,*,#3104,.F.);
#4054=ORIENTED_EDGE('',*,*,#3109,.T.);
#4055=ORIENTED_EDGE('',*,*,#3110,.T.);
#4056=ORIENTED_EDGE('',*,*,#3111,.T.);
#4057=ORIENTED_EDGE('',*,*,#3107,.F.);
#4058=ORIENTED_EDGE('',*,*,#3112,.T.);
#4059=ORIENTED_EDGE('',*,*,#3113,.F.);
#4060=ORIENTED_EDGE('',*,*,#3114,.T.);
#4061=ORIENTED_EDGE('',*,*,#3115,.T.);
#4062=ORIENTED_EDGE('',*,*,#3116,.T.);
#4063=ORIENTED_EDGE('',*,*,#3117,.T.);
#4064=ORIENTED_EDGE('',*,*,#3118,.T.);
#4065=ORIENTED_EDGE('',*,*,#3119,.F.);
#4066=ORIENTED_EDGE('',*,*,#3120,.T.);
#4067=ORIENTED_EDGE('',*,*,#3121,.T.);
#4068=ORIENTED_EDGE('',*,*,#3122,.T.);
#4069=ORIENTED_EDGE('',*,*,#3117,.F.);
#4070=ORIENTED_EDGE('',*,*,#3123,.T.);
#4071=ORIENTED_EDGE('',*,*,#3124,.T.);
#4072=ORIENTED_EDGE('',*,*,#3125,.T.);
#4073=ORIENTED_EDGE('',*,*,#3121,.F.);
#4074=ORIENTED_EDGE('',*,*,#3126,.T.);
#4075=ORIENTED_EDGE('',*,*,#3127,.T.);
#4076=ORIENTED_EDGE('',*,*,#3128,.T.);
#4077=ORIENTED_EDGE('',*,*,#3124,.F.);
#4078=ORIENTED_EDGE('',*,*,#3129,.T.);
#4079=ORIENTED_EDGE('',*,*,#3130,.T.);
#4080=ORIENTED_EDGE('',*,*,#3131,.T.);
#4081=ORIENTED_EDGE('',*,*,#3127,.F.);
#4082=ORIENTED_EDGE('',*,*,#3132,.T.);
#4083=ORIENTED_EDGE('',*,*,#3133,.T.);
#4084=ORIENTED_EDGE('',*,*,#3134,.T.);
#4085=ORIENTED_EDGE('',*,*,#3130,.F.);
#4086=ORIENTED_EDGE('',*,*,#3135,.T.);
#4087=ORIENTED_EDGE('',*,*,#3136,.T.);
#4088=ORIENTED_EDGE('',*,*,#3137,.T.);
#4089=ORIENTED_EDGE('',*,*,#3133,.F.);
#4090=ORIENTED_EDGE('',*,*,#3138,.T.);
#4091=ORIENTED_EDGE('',*,*,#3139,.T.);
#4092=ORIENTED_EDGE('',*,*,#3140,.T.);
#4093=ORIENTED_EDGE('',*,*,#3136,.F.);
#4094=ORIENTED_EDGE('',*,*,#3141,.T.);
#4095=ORIENTED_EDGE('',*,*,#3142,.T.);
#4096=ORIENTED_EDGE('',*,*,#3143,.T.);
#4097=ORIENTED_EDGE('',*,*,#3139,.F.);
#4098=ORIENTED_EDGE('',*,*,#3144,.T.);
#4099=ORIENTED_EDGE('',*,*,#3145,.T.);
#4100=ORIENTED_EDGE('',*,*,#3146,.T.);
#4101=ORIENTED_EDGE('',*,*,#3142,.F.);
#4102=ORIENTED_EDGE('',*,*,#3147,.T.);
#4103=ORIENTED_EDGE('',*,*,#3148,.F.);
#4104=ORIENTED_EDGE('',*,*,#3149,.T.);
#4105=ORIENTED_EDGE('',*,*,#3150,.F.);
#4106=ORIENTED_EDGE('',*,*,#3151,.T.);
#4107=ORIENTED_EDGE('',*,*,#3152,.T.);
#4108=ORIENTED_EDGE('',*,*,#3153,.T.);
#4109=ORIENTED_EDGE('',*,*,#3154,.T.);
#4110=ORIENTED_EDGE('',*,*,#3155,.F.);
#4111=ORIENTED_EDGE('',*,*,#3156,.T.);
#4112=ORIENTED_EDGE('',*,*,#3157,.T.);
#4113=ORIENTED_EDGE('',*,*,#3158,.T.);
#4114=ORIENTED_EDGE('',*,*,#3153,.F.);
#4115=ORIENTED_EDGE('',*,*,#3159,.T.);
#4116=ORIENTED_EDGE('',*,*,#3160,.T.);
#4117=ORIENTED_EDGE('',*,*,#3161,.T.);
#4118=ORIENTED_EDGE('',*,*,#3157,.F.);
#4119=ORIENTED_EDGE('',*,*,#3162,.T.);
#4120=ORIENTED_EDGE('',*,*,#3163,.T.);
#4121=ORIENTED_EDGE('',*,*,#3164,.T.);
#4122=ORIENTED_EDGE('',*,*,#3160,.F.);
#4123=ORIENTED_EDGE('',*,*,#3165,.T.);
#4124=ORIENTED_EDGE('',*,*,#3166,.T.);
#4125=ORIENTED_EDGE('',*,*,#3167,.T.);
#4126=ORIENTED_EDGE('',*,*,#3163,.F.);
#4127=ORIENTED_EDGE('',*,*,#3168,.T.);
#4128=ORIENTED_EDGE('',*,*,#3169,.T.);
#4129=ORIENTED_EDGE('',*,*,#3170,.T.);
#4130=ORIENTED_EDGE('',*,*,#3166,.F.);
#4131=ORIENTED_EDGE('',*,*,#3171,.T.);
#4132=ORIENTED_EDGE('',*,*,#3172,.T.);
#4133=ORIENTED_EDGE('',*,*,#3173,.T.);
#4134=ORIENTED_EDGE('',*,*,#3169,.F.);
#4135=ORIENTED_EDGE('',*,*,#3174,.T.);
#4136=ORIENTED_EDGE('',*,*,#3175,.T.);
#4137=ORIENTED_EDGE('',*,*,#3176,.T.);
#4138=ORIENTED_EDGE('',*,*,#3172,.F.);
#4139=ORIENTED_EDGE('',*,*,#3177,.T.);
#4140=ORIENTED_EDGE('',*,*,#3178,.T.);
#4141=ORIENTED_EDGE('',*,*,#3179,.T.);
#4142=ORIENTED_EDGE('',*,*,#3175,.F.);
#4143=ORIENTED_EDGE('',*,*,#3180,.T.);
#4144=ORIENTED_EDGE('',*,*,#3181,.T.);
#4145=ORIENTED_EDGE('',*,*,#3182,.T.);
#4146=ORIENTED_EDGE('',*,*,#3178,.F.);
#4147=ORIENTED_EDGE('',*,*,#3183,.T.);
#4148=ORIENTED_EDGE('',*,*,#3184,.F.);
#4149=ORIENTED_EDGE('',*,*,#3185,.T.);
#4150=ORIENTED_EDGE('',*,*,#3186,.T.);
#4151=ORIENTED_EDGE('',*,*,#3187,.F.);
#4152=ORIENTED_EDGE('',*,*,#3188,.T.);
#4153=ORIENTED_EDGE('',*,*,#3189,.T.);
#4154=ORIENTED_EDGE('',*,*,#3190,.T.);
#4155=ORIENTED_EDGE('',*,*,#3191,.F.);
#4156=ORIENTED_EDGE('',*,*,#3192,.F.);
#4157=ORIENTED_EDGE('',*,*,#3193,.T.);
#4158=ORIENTED_EDGE('',*,*,#3194,.T.);
#4159=ORIENTED_EDGE('',*,*,#3189,.F.);
#4160=ORIENTED_EDGE('',*,*,#3195,.F.);
#4161=ORIENTED_EDGE('',*,*,#3196,.T.);
#4162=ORIENTED_EDGE('',*,*,#3197,.T.);
#4163=ORIENTED_EDGE('',*,*,#3193,.F.);
#4164=ORIENTED_EDGE('',*,*,#3198,.F.);
#4165=ORIENTED_EDGE('',*,*,#3199,.T.);
#4166=ORIENTED_EDGE('',*,*,#3200,.T.);
#4167=ORIENTED_EDGE('',*,*,#3196,.F.);
#4168=ORIENTED_EDGE('',*,*,#3201,.F.);
#4169=ORIENTED_EDGE('',*,*,#3202,.T.);
#4170=ORIENTED_EDGE('',*,*,#3203,.T.);
#4171=ORIENTED_EDGE('',*,*,#3199,.F.);
#4172=ORIENTED_EDGE('',*,*,#3204,.F.);
#4173=ORIENTED_EDGE('',*,*,#3205,.T.);
#4174=ORIENTED_EDGE('',*,*,#3206,.T.);
#4175=ORIENTED_EDGE('',*,*,#3202,.F.);
#4176=ORIENTED_EDGE('',*,*,#3207,.F.);
#4177=ORIENTED_EDGE('',*,*,#3208,.T.);
#4178=ORIENTED_EDGE('',*,*,#3209,.T.);
#4179=ORIENTED_EDGE('',*,*,#3205,.F.);
#4180=ORIENTED_EDGE('',*,*,#3210,.F.);
#4181=ORIENTED_EDGE('',*,*,#3211,.T.);
#4182=ORIENTED_EDGE('',*,*,#3212,.T.);
#4183=ORIENTED_EDGE('',*,*,#3208,.F.);
#4184=ORIENTED_EDGE('',*,*,#3213,.F.);
#4185=ORIENTED_EDGE('',*,*,#3214,.T.);
#4186=ORIENTED_EDGE('',*,*,#3215,.T.);
#4187=ORIENTED_EDGE('',*,*,#3211,.F.);
#4188=ORIENTED_EDGE('',*,*,#3216,.F.);
#4189=ORIENTED_EDGE('',*,*,#3217,.T.);
#4190=ORIENTED_EDGE('',*,*,#3218,.T.);
#4191=ORIENTED_EDGE('',*,*,#3214,.F.);
#4192=ORIENTED_EDGE('',*,*,#3219,.F.);
#4193=ORIENTED_EDGE('',*,*,#3220,.T.);
#4194=ORIENTED_EDGE('',*,*,#3221,.T.);
#4195=ORIENTED_EDGE('',*,*,#3217,.F.);
#4196=ORIENTED_EDGE('',*,*,#3222,.F.);
#4197=ORIENTED_EDGE('',*,*,#3223,.F.);
#4198=ORIENTED_EDGE('',*,*,#3224,.F.);
#4199=ORIENTED_EDGE('',*,*,#3225,.F.);
#4200=ORIENTED_EDGE('',*,*,#3226,.T.);
#4201=ORIENTED_EDGE('',*,*,#3227,.T.);
#4202=ORIENTED_EDGE('',*,*,#3228,.T.);
#4203=ORIENTED_EDGE('',*,*,#3229,.F.);
#4204=ORIENTED_EDGE('',*,*,#3230,.F.);
#4205=ORIENTED_EDGE('',*,*,#3231,.T.);
#4206=ORIENTED_EDGE('',*,*,#3232,.T.);
#4207=ORIENTED_EDGE('',*,*,#3227,.F.);
#4208=ORIENTED_EDGE('',*,*,#3233,.F.);
#4209=ORIENTED_EDGE('',*,*,#3234,.T.);
#4210=ORIENTED_EDGE('',*,*,#3235,.T.);
#4211=ORIENTED_EDGE('',*,*,#3231,.F.);
#4212=ORIENTED_EDGE('',*,*,#3236,.F.);
#4213=ORIENTED_EDGE('',*,*,#3237,.T.);
#4214=ORIENTED_EDGE('',*,*,#3238,.T.);
#4215=ORIENTED_EDGE('',*,*,#3234,.F.);
#4216=ORIENTED_EDGE('',*,*,#3239,.F.);
#4217=ORIENTED_EDGE('',*,*,#3240,.T.);
#4218=ORIENTED_EDGE('',*,*,#3241,.T.);
#4219=ORIENTED_EDGE('',*,*,#3237,.F.);
#4220=ORIENTED_EDGE('',*,*,#3242,.F.);
#4221=ORIENTED_EDGE('',*,*,#3243,.T.);
#4222=ORIENTED_EDGE('',*,*,#3244,.T.);
#4223=ORIENTED_EDGE('',*,*,#3240,.F.);
#4224=ORIENTED_EDGE('',*,*,#3245,.F.);
#4225=ORIENTED_EDGE('',*,*,#3246,.T.);
#4226=ORIENTED_EDGE('',*,*,#3247,.T.);
#4227=ORIENTED_EDGE('',*,*,#3243,.F.);
#4228=ORIENTED_EDGE('',*,*,#3248,.F.);
#4229=ORIENTED_EDGE('',*,*,#3249,.T.);
#4230=ORIENTED_EDGE('',*,*,#3250,.T.);
#4231=ORIENTED_EDGE('',*,*,#3246,.F.);
#4232=ORIENTED_EDGE('',*,*,#3251,.F.);
#4233=ORIENTED_EDGE('',*,*,#3252,.T.);
#4234=ORIENTED_EDGE('',*,*,#3253,.T.);
#4235=ORIENTED_EDGE('',*,*,#3249,.F.);
#4236=ORIENTED_EDGE('',*,*,#3254,.F.);
#4237=ORIENTED_EDGE('',*,*,#3255,.T.);
#4238=ORIENTED_EDGE('',*,*,#3256,.T.);
#4239=ORIENTED_EDGE('',*,*,#3252,.F.);
#4240=ORIENTED_EDGE('',*,*,#3257,.F.);
#4241=ORIENTED_EDGE('',*,*,#3258,.T.);
#4242=ORIENTED_EDGE('',*,*,#3259,.T.);
#4243=ORIENTED_EDGE('',*,*,#3255,.F.);
#4244=ORIENTED_EDGE('',*,*,#3260,.F.);
#4245=ORIENTED_EDGE('',*,*,#3261,.F.);
#4246=ORIENTED_EDGE('',*,*,#3262,.F.);
#4247=ORIENTED_EDGE('',*,*,#3263,.F.);
#4248=ORIENTED_EDGE('',*,*,#3264,.T.);
#4249=ORIENTED_EDGE('',*,*,#3265,.T.);
#4250=ORIENTED_EDGE('',*,*,#3266,.T.);
#4251=ORIENTED_EDGE('',*,*,#3267,.F.);
#4252=ORIENTED_EDGE('',*,*,#3268,.F.);
#4253=ORIENTED_EDGE('',*,*,#3269,.T.);
#4254=ORIENTED_EDGE('',*,*,#3270,.T.);
#4255=ORIENTED_EDGE('',*,*,#3265,.F.);
#4256=ORIENTED_EDGE('',*,*,#3271,.F.);
#4257=ORIENTED_EDGE('',*,*,#3272,.T.);
#4258=ORIENTED_EDGE('',*,*,#3273,.T.);
#4259=ORIENTED_EDGE('',*,*,#3269,.F.);
#4260=ORIENTED_EDGE('',*,*,#3274,.F.);
#4261=ORIENTED_EDGE('',*,*,#3275,.T.);
#4262=ORIENTED_EDGE('',*,*,#3276,.T.);
#4263=ORIENTED_EDGE('',*,*,#3272,.F.);
#4264=ORIENTED_EDGE('',*,*,#3277,.F.);
#4265=ORIENTED_EDGE('',*,*,#3278,.T.);
#4266=ORIENTED_EDGE('',*,*,#3279,.T.);
#4267=ORIENTED_EDGE('',*,*,#3275,.F.);
#4268=ORIENTED_EDGE('',*,*,#3280,.F.);
#4269=ORIENTED_EDGE('',*,*,#3281,.T.);
#4270=ORIENTED_EDGE('',*,*,#3282,.T.);
#4271=ORIENTED_EDGE('',*,*,#3278,.F.);
#4272=ORIENTED_EDGE('',*,*,#3283,.F.);
#4273=ORIENTED_EDGE('',*,*,#3284,.T.);
#4274=ORIENTED_EDGE('',*,*,#3285,.T.);
#4275=ORIENTED_EDGE('',*,*,#3281,.F.);
#4276=ORIENTED_EDGE('',*,*,#3286,.F.);
#4277=ORIENTED_EDGE('',*,*,#3287,.T.);
#4278=ORIENTED_EDGE('',*,*,#3288,.T.);
#4279=ORIENTED_EDGE('',*,*,#3284,.F.);
#4280=ORIENTED_EDGE('',*,*,#3289,.F.);
#4281=ORIENTED_EDGE('',*,*,#3290,.T.);
#4282=ORIENTED_EDGE('',*,*,#3291,.T.);
#4283=ORIENTED_EDGE('',*,*,#3287,.F.);
#4284=ORIENTED_EDGE('',*,*,#3292,.F.);
#4285=ORIENTED_EDGE('',*,*,#3293,.T.);
#4286=ORIENTED_EDGE('',*,*,#3294,.T.);
#4287=ORIENTED_EDGE('',*,*,#3290,.F.);
#4288=ORIENTED_EDGE('',*,*,#3295,.F.);
#4289=ORIENTED_EDGE('',*,*,#3296,.T.);
#4290=ORIENTED_EDGE('',*,*,#3297,.T.);
#4291=ORIENTED_EDGE('',*,*,#3293,.F.);
#4292=ORIENTED_EDGE('',*,*,#3298,.F.);
#4293=ORIENTED_EDGE('',*,*,#3299,.F.);
#4294=ORIENTED_EDGE('',*,*,#3300,.F.);
#4295=ORIENTED_EDGE('',*,*,#3301,.F.);
#4296=ORIENTED_EDGE('',*,*,#3302,.T.);
#4297=ORIENTED_EDGE('',*,*,#3303,.T.);
#4298=ORIENTED_EDGE('',*,*,#3304,.T.);
#4299=ORIENTED_EDGE('',*,*,#3305,.F.);
#4300=ORIENTED_EDGE('',*,*,#3306,.F.);
#4301=ORIENTED_EDGE('',*,*,#3307,.T.);
#4302=ORIENTED_EDGE('',*,*,#3308,.T.);
#4303=ORIENTED_EDGE('',*,*,#3303,.F.);
#4304=ORIENTED_EDGE('',*,*,#3309,.F.);
#4305=ORIENTED_EDGE('',*,*,#3310,.T.);
#4306=ORIENTED_EDGE('',*,*,#3311,.T.);
#4307=ORIENTED_EDGE('',*,*,#3307,.F.);
#4308=ORIENTED_EDGE('',*,*,#3312,.F.);
#4309=ORIENTED_EDGE('',*,*,#3313,.T.);
#4310=ORIENTED_EDGE('',*,*,#3314,.T.);
#4311=ORIENTED_EDGE('',*,*,#3310,.F.);
#4312=ORIENTED_EDGE('',*,*,#3315,.F.);
#4313=ORIENTED_EDGE('',*,*,#3316,.T.);
#4314=ORIENTED_EDGE('',*,*,#3317,.T.);
#4315=ORIENTED_EDGE('',*,*,#3313,.F.);
#4316=ORIENTED_EDGE('',*,*,#3318,.F.);
#4317=ORIENTED_EDGE('',*,*,#3319,.T.);
#4318=ORIENTED_EDGE('',*,*,#3320,.T.);
#4319=ORIENTED_EDGE('',*,*,#3316,.F.);
#4320=ORIENTED_EDGE('',*,*,#3321,.F.);
#4321=ORIENTED_EDGE('',*,*,#3322,.T.);
#4322=ORIENTED_EDGE('',*,*,#3323,.T.);
#4323=ORIENTED_EDGE('',*,*,#3319,.F.);
#4324=ORIENTED_EDGE('',*,*,#3324,.F.);
#4325=ORIENTED_EDGE('',*,*,#3325,.T.);
#4326=ORIENTED_EDGE('',*,*,#3326,.T.);
#4327=ORIENTED_EDGE('',*,*,#3322,.F.);
#4328=ORIENTED_EDGE('',*,*,#3327,.F.);
#4329=ORIENTED_EDGE('',*,*,#3328,.T.);
#4330=ORIENTED_EDGE('',*,*,#3329,.T.);
#4331=ORIENTED_EDGE('',*,*,#3325,.F.);
#4332=ORIENTED_EDGE('',*,*,#3330,.F.);
#4333=ORIENTED_EDGE('',*,*,#3331,.T.);
#4334=ORIENTED_EDGE('',*,*,#3332,.T.);
#4335=ORIENTED_EDGE('',*,*,#3328,.F.);
#4336=ORIENTED_EDGE('',*,*,#3333,.F.);
#4337=ORIENTED_EDGE('',*,*,#3334,.T.);
#4338=ORIENTED_EDGE('',*,*,#3335,.T.);
#4339=ORIENTED_EDGE('',*,*,#3331,.F.);
#4340=ORIENTED_EDGE('',*,*,#3336,.F.);
#4341=ORIENTED_EDGE('',*,*,#3337,.F.);
#4342=ORIENTED_EDGE('',*,*,#3338,.F.);
#4343=ORIENTED_EDGE('',*,*,#3339,.F.);
#4344=ORIENTED_EDGE('',*,*,#3340,.T.);
#4345=ORIENTED_EDGE('',*,*,#3341,.T.);
#4346=ORIENTED_EDGE('',*,*,#3342,.T.);
#4347=ORIENTED_EDGE('',*,*,#3343,.T.);
#4348=ORIENTED_EDGE('',*,*,#3344,.F.);
#4349=ORIENTED_EDGE('',*,*,#3345,.T.);
#4350=ORIENTED_EDGE('',*,*,#3346,.T.);
#4351=ORIENTED_EDGE('',*,*,#3347,.T.);
#4352=ORIENTED_EDGE('',*,*,#3342,.F.);
#4353=ORIENTED_EDGE('',*,*,#3348,.T.);
#4354=ORIENTED_EDGE('',*,*,#3349,.T.);
#4355=ORIENTED_EDGE('',*,*,#3350,.T.);
#4356=ORIENTED_EDGE('',*,*,#3346,.F.);
#4357=ORIENTED_EDGE('',*,*,#3351,.T.);
#4358=ORIENTED_EDGE('',*,*,#3352,.T.);
#4359=ORIENTED_EDGE('',*,*,#3353,.T.);
#4360=ORIENTED_EDGE('',*,*,#3349,.F.);
#4361=ORIENTED_EDGE('',*,*,#3354,.T.);
#4362=ORIENTED_EDGE('',*,*,#3352,.F.);
#4363=ORIENTED_EDGE('',*,*,#3355,.T.);
#4364=ORIENTED_EDGE('',*,*,#3356,.T.);
#4365=ORIENTED_EDGE('',*,*,#3357,.T.);
#4366=ORIENTED_EDGE('',*,*,#3356,.F.);
#4367=ORIENTED_EDGE('',*,*,#3358,.T.);
#4368=ORIENTED_EDGE('',*,*,#3344,.T.);
#4369=ORIENTED_EDGE('',*,*,#3354,.F.);
#4370=ORIENTED_EDGE('',*,*,#3359,.F.);
#4371=ORIENTED_EDGE('',*,*,#3360,.F.);
#4372=ORIENTED_EDGE('',*,*,#3361,.F.);
#4373=ORIENTED_EDGE('',*,*,#3362,.F.);
#4374=ORIENTED_EDGE('',*,*,#3363,.T.);
#4375=ORIENTED_EDGE('',*,*,#3357,.F.);
#4376=ORIENTED_EDGE('',*,*,#3364,.F.);
#4377=ORIENTED_EDGE('',*,*,#3365,.F.);
#4378=ORIENTED_EDGE('',*,*,#3366,.F.);
#4379=ORIENTED_EDGE('',*,*,#3359,.T.);
#4380=ORIENTED_EDGE('',*,*,#3343,.F.);
#4381=ORIENTED_EDGE('',*,*,#3367,.F.);
#4382=ORIENTED_EDGE('',*,*,#3368,.F.);
#4383=ORIENTED_EDGE('',*,*,#3364,.T.);
#4384=ORIENTED_EDGE('',*,*,#3369,.F.);
#4385=ORIENTED_EDGE('',*,*,#3370,.F.);
#4386=ORIENTED_EDGE('',*,*,#3371,.F.);
#4387=ORIENTED_EDGE('',*,*,#3372,.F.);
#4388=ORIENTED_EDGE('',*,*,#3373,.F.);
#4389=ORIENTED_EDGE('',*,*,#3374,.F.);
#4390=ORIENTED_EDGE('',*,*,#3375,.F.);
#4391=ORIENTED_EDGE('',*,*,#3376,.F.);
#4392=ORIENTED_EDGE('',*,*,#3377,.F.);
#4393=ORIENTED_EDGE('',*,*,#3341,.F.);
#4394=ORIENTED_EDGE('',*,*,#3358,.F.);
#4395=ORIENTED_EDGE('',*,*,#3355,.F.);
#4396=ORIENTED_EDGE('',*,*,#3351,.F.);
#4397=ORIENTED_EDGE('',*,*,#3348,.F.);
#4398=ORIENTED_EDGE('',*,*,#3345,.F.);
#4399=ORIENTED_EDGE('',*,*,#3378,.T.);
#4400=ORIENTED_EDGE('',*,*,#3379,.T.);
#4401=ORIENTED_EDGE('',*,*,#3369,.T.);
#4402=ORIENTED_EDGE('',*,*,#3380,.T.);
#4403=ORIENTED_EDGE('',*,*,#3381,.T.);
#4404=ORIENTED_EDGE('',*,*,#3382,.F.);
#4405=ORIENTED_EDGE('',*,*,#3371,.T.);
#4406=ORIENTED_EDGE('',*,*,#3377,.T.);
#4407=ORIENTED_EDGE('',*,*,#3383,.T.);
#4408=ORIENTED_EDGE('',*,*,#3384,.T.);
#4409=ORIENTED_EDGE('',*,*,#3380,.F.);
#4410=ORIENTED_EDGE('',*,*,#3385,.T.);
#4411=ORIENTED_EDGE('',*,*,#3373,.T.);
#4412=ORIENTED_EDGE('',*,*,#3386,.T.);
#4413=ORIENTED_EDGE('',*,*,#3387,.T.);
#4414=ORIENTED_EDGE('',*,*,#3383,.F.);
#4415=ORIENTED_EDGE('',*,*,#3376,.T.);
#4416=ORIENTED_EDGE('',*,*,#3388,.T.);
#4417=ORIENTED_EDGE('',*,*,#3386,.F.);
#4418=ORIENTED_EDGE('',*,*,#3372,.T.);
#4419=ORIENTED_EDGE('',*,*,#3382,.T.);
#4420=ORIENTED_EDGE('',*,*,#3388,.F.);
#4421=ORIENTED_EDGE('',*,*,#3389,.F.);
#4422=ORIENTED_EDGE('',*,*,#3390,.T.);
#4423=ORIENTED_EDGE('',*,*,#3391,.T.);
#4424=ORIENTED_EDGE('',*,*,#3381,.F.);
#4425=ORIENTED_EDGE('',*,*,#3392,.F.);
#4426=ORIENTED_EDGE('',*,*,#3393,.T.);
#4427=ORIENTED_EDGE('',*,*,#3389,.T.);
#4428=ORIENTED_EDGE('',*,*,#3378,.F.);
#4429=ORIENTED_EDGE('',*,*,#3370,.T.);
#4430=ORIENTED_EDGE('',*,*,#3379,.F.);
#4431=ORIENTED_EDGE('',*,*,#3394,.T.);
#4432=ORIENTED_EDGE('',*,*,#3395,.T.);
#4433=ORIENTED_EDGE('',*,*,#3396,.T.);
#4434=ORIENTED_EDGE('',*,*,#3394,.F.);
#4435=ORIENTED_EDGE('',*,*,#3385,.F.);
#4436=ORIENTED_EDGE('',*,*,#3375,.T.);
#4437=ORIENTED_EDGE('',*,*,#3397,.T.);
#4438=ORIENTED_EDGE('',*,*,#3398,.T.);
#4439=ORIENTED_EDGE('',*,*,#3399,.T.);
#4440=ORIENTED_EDGE('',*,*,#3397,.F.);
#4441=ORIENTED_EDGE('',*,*,#3374,.T.);
#4442=ORIENTED_EDGE('',*,*,#3395,.F.);
#4443=ORIENTED_EDGE('',*,*,#3396,.F.);
#4444=ORIENTED_EDGE('',*,*,#3400,.T.);
#4445=ORIENTED_EDGE('',*,*,#3401,.F.);
#4446=ORIENTED_EDGE('',*,*,#3400,.F.);
#4447=ORIENTED_EDGE('',*,*,#3398,.F.);
#4448=ORIENTED_EDGE('',*,*,#3399,.F.);
#4449=ORIENTED_EDGE('',*,*,#3402,.T.);
#4450=ORIENTED_EDGE('',*,*,#3403,.F.);
#4451=ORIENTED_EDGE('',*,*,#3402,.F.);
#4452=ORIENTED_EDGE('',*,*,#3337,.T.);
#4453=ORIENTED_EDGE('',*,*,#3404,.T.);
#4454=ORIENTED_EDGE('',*,*,#3334,.F.);
#4455=ORIENTED_EDGE('',*,*,#3405,.F.);
#4456=ORIENTED_EDGE('',*,*,#3406,.F.);
#4457=ORIENTED_EDGE('',*,*,#3304,.F.);
#4458=ORIENTED_EDGE('',*,*,#3308,.F.);
#4459=ORIENTED_EDGE('',*,*,#3311,.F.);
#4460=ORIENTED_EDGE('',*,*,#3314,.F.);
#4461=ORIENTED_EDGE('',*,*,#3317,.F.);
#4462=ORIENTED_EDGE('',*,*,#3320,.F.);
#4463=ORIENTED_EDGE('',*,*,#3323,.F.);
#4464=ORIENTED_EDGE('',*,*,#3326,.F.);
#4465=ORIENTED_EDGE('',*,*,#3329,.F.);
#4466=ORIENTED_EDGE('',*,*,#3332,.F.);
#4467=ORIENTED_EDGE('',*,*,#3335,.F.);
#4468=ORIENTED_EDGE('',*,*,#3404,.F.);
#4469=ORIENTED_EDGE('',*,*,#3340,.F.);
#4470=ORIENTED_EDGE('',*,*,#3407,.F.);
#4471=ORIENTED_EDGE('',*,*,#3408,.F.);
#4472=ORIENTED_EDGE('',*,*,#3149,.F.);
#4473=ORIENTED_EDGE('',*,*,#3409,.F.);
#4474=ORIENTED_EDGE('',*,*,#3147,.F.);
#4475=ORIENTED_EDGE('',*,*,#3144,.F.);
#4476=ORIENTED_EDGE('',*,*,#3141,.F.);
#4477=ORIENTED_EDGE('',*,*,#3138,.F.);
#4478=ORIENTED_EDGE('',*,*,#3135,.F.);
#4479=ORIENTED_EDGE('',*,*,#3132,.F.);
#4480=ORIENTED_EDGE('',*,*,#3129,.F.);
#4481=ORIENTED_EDGE('',*,*,#3126,.F.);
#4482=ORIENTED_EDGE('',*,*,#3123,.F.);
#4483=ORIENTED_EDGE('',*,*,#3120,.F.);
#4484=ORIENTED_EDGE('',*,*,#3410,.F.);
#4485=ORIENTED_EDGE('',*,*,#3118,.F.);
#4486=ORIENTED_EDGE('',*,*,#3122,.F.);
#4487=ORIENTED_EDGE('',*,*,#3125,.F.);
#4488=ORIENTED_EDGE('',*,*,#3128,.F.);
#4489=ORIENTED_EDGE('',*,*,#3131,.F.);
#4490=ORIENTED_EDGE('',*,*,#3134,.F.);
#4491=ORIENTED_EDGE('',*,*,#3137,.F.);
#4492=ORIENTED_EDGE('',*,*,#3140,.F.);
#4493=ORIENTED_EDGE('',*,*,#3143,.F.);
#4494=ORIENTED_EDGE('',*,*,#3146,.F.);
#4495=ORIENTED_EDGE('',*,*,#3411,.F.);
#4496=ORIENTED_EDGE('',*,*,#3152,.F.);
#4497=ORIENTED_EDGE('',*,*,#3412,.F.);
#4498=ORIENTED_EDGE('',*,*,#3338,.T.);
#4499=ORIENTED_EDGE('',*,*,#3405,.T.);
#4500=ORIENTED_EDGE('',*,*,#3336,.T.);
#4501=ORIENTED_EDGE('',*,*,#3333,.T.);
#4502=ORIENTED_EDGE('',*,*,#3330,.T.);
#4503=ORIENTED_EDGE('',*,*,#3327,.T.);
#4504=ORIENTED_EDGE('',*,*,#3324,.T.);
#4505=ORIENTED_EDGE('',*,*,#3321,.T.);
#4506=ORIENTED_EDGE('',*,*,#3318,.T.);
#4507=ORIENTED_EDGE('',*,*,#3315,.T.);
#4508=ORIENTED_EDGE('',*,*,#3312,.T.);
#4509=ORIENTED_EDGE('',*,*,#3309,.T.);
#4510=ORIENTED_EDGE('',*,*,#3306,.T.);
#4511=ORIENTED_EDGE('',*,*,#3413,.F.);
#4512=ORIENTED_EDGE('',*,*,#3414,.F.);
#4513=ORIENTED_EDGE('',*,*,#3415,.F.);
#4514=ORIENTED_EDGE('',*,*,#3416,.F.);
#4515=ORIENTED_EDGE('',*,*,#3417,.F.);
#4516=ORIENTED_EDGE('',*,*,#3418,.F.);
#4517=ORIENTED_EDGE('',*,*,#3410,.T.);
#4518=ORIENTED_EDGE('',*,*,#3305,.T.);
#4519=ORIENTED_EDGE('',*,*,#3406,.T.);
#4520=ORIENTED_EDGE('',*,*,#3119,.T.);
#4521=ORIENTED_EDGE('',*,*,#3419,.T.);
#4522=ORIENTED_EDGE('',*,*,#3420,.T.);
#4523=ORIENTED_EDGE('',*,*,#3421,.T.);
#4524=ORIENTED_EDGE('',*,*,#3422,.T.);
#4525=ORIENTED_EDGE('',*,*,#3423,.T.);
#4526=ORIENTED_EDGE('',*,*,#3424,.T.);
#4527=ORIENTED_EDGE('',*,*,#3425,.T.);
#4528=ORIENTED_EDGE('',*,*,#3426,.T.);
#4529=ORIENTED_EDGE('',*,*,#3427,.T.);
#4530=ORIENTED_EDGE('',*,*,#3428,.T.);
#4531=ORIENTED_EDGE('',*,*,#3429,.T.);
#4532=ORIENTED_EDGE('',*,*,#3430,.T.);
#4533=ORIENTED_EDGE('',*,*,#3431,.T.);
#4534=ORIENTED_EDGE('',*,*,#3155,.T.);
#4535=ORIENTED_EDGE('',*,*,#3432,.T.);
#4536=ORIENTED_EDGE('',*,*,#3191,.T.);
#4537=ORIENTED_EDGE('',*,*,#3433,.T.);
#4538=ORIENTED_EDGE('',*,*,#3084,.T.);
#4539=ORIENTED_EDGE('',*,*,#3434,.T.);
#4540=ORIENTED_EDGE('',*,*,#3229,.T.);
#4541=ORIENTED_EDGE('',*,*,#3435,.T.);
#4542=ORIENTED_EDGE('',*,*,#3049,.T.);
#4543=ORIENTED_EDGE('',*,*,#3436,.T.);
#4544=ORIENTED_EDGE('',*,*,#3267,.T.);
#4545=ORIENTED_EDGE('',*,*,#3299,.T.);
#4546=ORIENTED_EDGE('',*,*,#3437,.T.);
#4547=ORIENTED_EDGE('',*,*,#3296,.F.);
#4548=ORIENTED_EDGE('',*,*,#3438,.F.);
#4549=ORIENTED_EDGE('',*,*,#3435,.F.);
#4550=ORIENTED_EDGE('',*,*,#3266,.F.);
#4551=ORIENTED_EDGE('',*,*,#3270,.F.);
#4552=ORIENTED_EDGE('',*,*,#3273,.F.);
#4553=ORIENTED_EDGE('',*,*,#3276,.F.);
#4554=ORIENTED_EDGE('',*,*,#3279,.F.);
#4555=ORIENTED_EDGE('',*,*,#3282,.F.);
#4556=ORIENTED_EDGE('',*,*,#3285,.F.);
#4557=ORIENTED_EDGE('',*,*,#3288,.F.);
#4558=ORIENTED_EDGE('',*,*,#3291,.F.);
#4559=ORIENTED_EDGE('',*,*,#3294,.F.);
#4560=ORIENTED_EDGE('',*,*,#3297,.F.);
#4561=ORIENTED_EDGE('',*,*,#3437,.F.);
#4562=ORIENTED_EDGE('',*,*,#3302,.F.);
#4563=ORIENTED_EDGE('',*,*,#3439,.F.);
#4564=ORIENTED_EDGE('',*,*,#3079,.F.);
#4565=ORIENTED_EDGE('',*,*,#3440,.F.);
#4566=ORIENTED_EDGE('',*,*,#3077,.F.);
#4567=ORIENTED_EDGE('',*,*,#3074,.F.);
#4568=ORIENTED_EDGE('',*,*,#3071,.F.);
#4569=ORIENTED_EDGE('',*,*,#3068,.F.);
#4570=ORIENTED_EDGE('',*,*,#3065,.F.);
#4571=ORIENTED_EDGE('',*,*,#3062,.F.);
#4572=ORIENTED_EDGE('',*,*,#3059,.F.);
#4573=ORIENTED_EDGE('',*,*,#3056,.F.);
#4574=ORIENTED_EDGE('',*,*,#3053,.F.);
#4575=ORIENTED_EDGE('',*,*,#3050,.F.);
#4576=ORIENTED_EDGE('',*,*,#3436,.F.);
#4577=ORIENTED_EDGE('',*,*,#3048,.F.);
#4578=ORIENTED_EDGE('',*,*,#3052,.F.);
#4579=ORIENTED_EDGE('',*,*,#3055,.F.);
#4580=ORIENTED_EDGE('',*,*,#3058,.F.);
#4581=ORIENTED_EDGE('',*,*,#3061,.F.);
#4582=ORIENTED_EDGE('',*,*,#3064,.F.);
#4583=ORIENTED_EDGE('',*,*,#3067,.F.);
#4584=ORIENTED_EDGE('',*,*,#3070,.F.);
#4585=ORIENTED_EDGE('',*,*,#3073,.F.);
#4586=ORIENTED_EDGE('',*,*,#3076,.F.);
#4587=ORIENTED_EDGE('',*,*,#3441,.F.);
#4588=ORIENTED_EDGE('',*,*,#3081,.F.);
#4589=ORIENTED_EDGE('',*,*,#3442,.F.);
#4590=ORIENTED_EDGE('',*,*,#3300,.T.);
#4591=ORIENTED_EDGE('',*,*,#3438,.T.);
#4592=ORIENTED_EDGE('',*,*,#3298,.T.);
#4593=ORIENTED_EDGE('',*,*,#3295,.T.);
#4594=ORIENTED_EDGE('',*,*,#3292,.T.);
#4595=ORIENTED_EDGE('',*,*,#3289,.T.);
#4596=ORIENTED_EDGE('',*,*,#3286,.T.);
#4597=ORIENTED_EDGE('',*,*,#3283,.T.);
#4598=ORIENTED_EDGE('',*,*,#3280,.T.);
#4599=ORIENTED_EDGE('',*,*,#3277,.T.);
#4600=ORIENTED_EDGE('',*,*,#3274,.T.);
#4601=ORIENTED_EDGE('',*,*,#3271,.T.);
#4602=ORIENTED_EDGE('',*,*,#3268,.T.);
#4603=ORIENTED_EDGE('',*,*,#3261,.T.);
#4604=ORIENTED_EDGE('',*,*,#3443,.T.);
#4605=ORIENTED_EDGE('',*,*,#3258,.F.);
#4606=ORIENTED_EDGE('',*,*,#3444,.F.);
#4607=ORIENTED_EDGE('',*,*,#3433,.F.);
#4608=ORIENTED_EDGE('',*,*,#3228,.F.);
#4609=ORIENTED_EDGE('',*,*,#3232,.F.);
#4610=ORIENTED_EDGE('',*,*,#3235,.F.);
#4611=ORIENTED_EDGE('',*,*,#3238,.F.);
#4612=ORIENTED_EDGE('',*,*,#3241,.F.);
#4613=ORIENTED_EDGE('',*,*,#3244,.F.);
#4614=ORIENTED_EDGE('',*,*,#3247,.F.);
#4615=ORIENTED_EDGE('',*,*,#3250,.F.);
#4616=ORIENTED_EDGE('',*,*,#3253,.F.);
#4617=ORIENTED_EDGE('',*,*,#3256,.F.);
#4618=ORIENTED_EDGE('',*,*,#3259,.F.);
#4619=ORIENTED_EDGE('',*,*,#3443,.F.);
#4620=ORIENTED_EDGE('',*,*,#3264,.F.);
#4621=ORIENTED_EDGE('',*,*,#3445,.F.);
#4622=ORIENTED_EDGE('',*,*,#3114,.F.);
#4623=ORIENTED_EDGE('',*,*,#3446,.F.);
#4624=ORIENTED_EDGE('',*,*,#3112,.F.);
#4625=ORIENTED_EDGE('',*,*,#3109,.F.);
#4626=ORIENTED_EDGE('',*,*,#3106,.F.);
#4627=ORIENTED_EDGE('',*,*,#3103,.F.);
#4628=ORIENTED_EDGE('',*,*,#3100,.F.);
#4629=ORIENTED_EDGE('',*,*,#3097,.F.);
#4630=ORIENTED_EDGE('',*,*,#3094,.F.);
#4631=ORIENTED_EDGE('',*,*,#3091,.F.);
#4632=ORIENTED_EDGE('',*,*,#3088,.F.);
#4633=ORIENTED_EDGE('',*,*,#3085,.F.);
#4634=ORIENTED_EDGE('',*,*,#3434,.F.);
#4635=ORIENTED_EDGE('',*,*,#3083,.F.);
#4636=ORIENTED_EDGE('',*,*,#3087,.F.);
#4637=ORIENTED_EDGE('',*,*,#3090,.F.);
#4638=ORIENTED_EDGE('',*,*,#3093,.F.);
#4639=ORIENTED_EDGE('',*,*,#3096,.F.);
#4640=ORIENTED_EDGE('',*,*,#3099,.F.);
#4641=ORIENTED_EDGE('',*,*,#3102,.F.);
#4642=ORIENTED_EDGE('',*,*,#3105,.F.);
#4643=ORIENTED_EDGE('',*,*,#3108,.F.);
#4644=ORIENTED_EDGE('',*,*,#3111,.F.);
#4645=ORIENTED_EDGE('',*,*,#3447,.F.);
#4646=ORIENTED_EDGE('',*,*,#3116,.F.);
#4647=ORIENTED_EDGE('',*,*,#3448,.F.);
#4648=ORIENTED_EDGE('',*,*,#3262,.T.);
#4649=ORIENTED_EDGE('',*,*,#3444,.T.);
#4650=ORIENTED_EDGE('',*,*,#3260,.T.);
#4651=ORIENTED_EDGE('',*,*,#3257,.T.);
#4652=ORIENTED_EDGE('',*,*,#3254,.T.);
#4653=ORIENTED_EDGE('',*,*,#3251,.T.);
#4654=ORIENTED_EDGE('',*,*,#3248,.T.);
#4655=ORIENTED_EDGE('',*,*,#3245,.T.);
#4656=ORIENTED_EDGE('',*,*,#3242,.T.);
#4657=ORIENTED_EDGE('',*,*,#3239,.T.);
#4658=ORIENTED_EDGE('',*,*,#3236,.T.);
#4659=ORIENTED_EDGE('',*,*,#3233,.T.);
#4660=ORIENTED_EDGE('',*,*,#3230,.T.);
#4661=ORIENTED_EDGE('',*,*,#3223,.T.);
#4662=ORIENTED_EDGE('',*,*,#3449,.T.);
#4663=ORIENTED_EDGE('',*,*,#3220,.F.);
#4664=ORIENTED_EDGE('',*,*,#3450,.F.);
#4665=ORIENTED_EDGE('',*,*,#3431,.F.);
#4666=ORIENTED_EDGE('',*,*,#3190,.F.);
#4667=ORIENTED_EDGE('',*,*,#3194,.F.);
#4668=ORIENTED_EDGE('',*,*,#3197,.F.);
#4669=ORIENTED_EDGE('',*,*,#3200,.F.);
#4670=ORIENTED_EDGE('',*,*,#3203,.F.);
#4671=ORIENTED_EDGE('',*,*,#3206,.F.);
#4672=ORIENTED_EDGE('',*,*,#3209,.F.);
#4673=ORIENTED_EDGE('',*,*,#3212,.F.);
#4674=ORIENTED_EDGE('',*,*,#3215,.F.);
#4675=ORIENTED_EDGE('',*,*,#3218,.F.);
#4676=ORIENTED_EDGE('',*,*,#3221,.F.);
#4677=ORIENTED_EDGE('',*,*,#3449,.F.);
#4678=ORIENTED_EDGE('',*,*,#3226,.F.);
#4679=ORIENTED_EDGE('',*,*,#3451,.F.);
#4680=ORIENTED_EDGE('',*,*,#3185,.F.);
#4681=ORIENTED_EDGE('',*,*,#3452,.F.);
#4682=ORIENTED_EDGE('',*,*,#3183,.F.);
#4683=ORIENTED_EDGE('',*,*,#3180,.F.);
#4684=ORIENTED_EDGE('',*,*,#3177,.F.);
#4685=ORIENTED_EDGE('',*,*,#3174,.F.);
#4686=ORIENTED_EDGE('',*,*,#3171,.F.);
#4687=ORIENTED_EDGE('',*,*,#3168,.F.);
#4688=ORIENTED_EDGE('',*,*,#3165,.F.);
#4689=ORIENTED_EDGE('',*,*,#3162,.F.);
#4690=ORIENTED_EDGE('',*,*,#3159,.F.);
#4691=ORIENTED_EDGE('',*,*,#3156,.F.);
#4692=ORIENTED_EDGE('',*,*,#3432,.F.);
#4693=ORIENTED_EDGE('',*,*,#3154,.F.);
#4694=ORIENTED_EDGE('',*,*,#3158,.F.);
#4695=ORIENTED_EDGE('',*,*,#3161,.F.);
#4696=ORIENTED_EDGE('',*,*,#3164,.F.);
#4697=ORIENTED_EDGE('',*,*,#3167,.F.);
#4698=ORIENTED_EDGE('',*,*,#3170,.F.);
#4699=ORIENTED_EDGE('',*,*,#3173,.F.);
#4700=ORIENTED_EDGE('',*,*,#3176,.F.);
#4701=ORIENTED_EDGE('',*,*,#3179,.F.);
#4702=ORIENTED_EDGE('',*,*,#3182,.F.);
#4703=ORIENTED_EDGE('',*,*,#3453,.F.);
#4704=ORIENTED_EDGE('',*,*,#3188,.F.);
#4705=ORIENTED_EDGE('',*,*,#3454,.F.);
#4706=ORIENTED_EDGE('',*,*,#3455,.F.);
#4707=ORIENTED_EDGE('',*,*,#3224,.T.);
#4708=ORIENTED_EDGE('',*,*,#3450,.T.);
#4709=ORIENTED_EDGE('',*,*,#3222,.T.);
#4710=ORIENTED_EDGE('',*,*,#3219,.T.);
#4711=ORIENTED_EDGE('',*,*,#3216,.T.);
#4712=ORIENTED_EDGE('',*,*,#3213,.T.);
#4713=ORIENTED_EDGE('',*,*,#3210,.T.);
#4714=ORIENTED_EDGE('',*,*,#3207,.T.);
#4715=ORIENTED_EDGE('',*,*,#3204,.T.);
#4716=ORIENTED_EDGE('',*,*,#3201,.T.);
#4717=ORIENTED_EDGE('',*,*,#3198,.T.);
#4718=ORIENTED_EDGE('',*,*,#3195,.T.);
#4719=ORIENTED_EDGE('',*,*,#3192,.T.);
#4720=ORIENTED_EDGE('',*,*,#3408,.T.);
#4721=ORIENTED_EDGE('',*,*,#3361,.T.);
#4722=ORIENTED_EDGE('',*,*,#3454,.T.);
#4723=ORIENTED_EDGE('',*,*,#3187,.T.);
#4724=ORIENTED_EDGE('',*,*,#3365,.T.);
#4725=ORIENTED_EDGE('',*,*,#3368,.T.);
#4726=ORIENTED_EDGE('',*,*,#3456,.T.);
#4727=ORIENTED_EDGE('',*,*,#3457,.T.);
#4728=ORIENTED_EDGE('',*,*,#3458,.T.);
#4729=ORIENTED_EDGE('',*,*,#3150,.T.);
#4730=ORIENTED_EDGE('',*,*,#3459,.T.);
#4731=ORIENTED_EDGE('',*,*,#3460,.T.);
#4732=ORIENTED_EDGE('',*,*,#3461,.T.);
#4733=ORIENTED_EDGE('',*,*,#3462,.T.);
#4734=ORIENTED_EDGE('',*,*,#3463,.T.);
#4735=ORIENTED_EDGE('',*,*,#3464,.T.);
#4736=ORIENTED_EDGE('',*,*,#3465,.T.);
#4737=ORIENTED_EDGE('',*,*,#3466,.T.);
#4738=ORIENTED_EDGE('',*,*,#3467,.T.);
#4739=ORIENTED_EDGE('',*,*,#3468,.T.);
#4740=ORIENTED_EDGE('',*,*,#3469,.T.);
#4741=ORIENTED_EDGE('',*,*,#3470,.T.);
#4742=ORIENTED_EDGE('',*,*,#3366,.T.);
#4743=ORIENTED_EDGE('',*,*,#3186,.F.);
#4744=ORIENTED_EDGE('',*,*,#3451,.T.);
#4745=ORIENTED_EDGE('',*,*,#3225,.T.);
#4746=ORIENTED_EDGE('',*,*,#3455,.T.);
#4747=ORIENTED_EDGE('',*,*,#3360,.T.);
#4748=ORIENTED_EDGE('',*,*,#3184,.T.);
#4749=ORIENTED_EDGE('',*,*,#3453,.T.);
#4750=ORIENTED_EDGE('',*,*,#3181,.F.);
#4751=ORIENTED_EDGE('',*,*,#3452,.T.);
#4752=ORIENTED_EDGE('',*,*,#3362,.T.);
#4753=ORIENTED_EDGE('',*,*,#3407,.T.);
#4754=ORIENTED_EDGE('',*,*,#3339,.T.);
#4755=ORIENTED_EDGE('',*,*,#3412,.T.);
#4756=ORIENTED_EDGE('',*,*,#3151,.F.);
#4757=ORIENTED_EDGE('',*,*,#3471,.T.);
#4758=ORIENTED_EDGE('',*,*,#3148,.T.);
#4759=ORIENTED_EDGE('',*,*,#3411,.T.);
#4760=ORIENTED_EDGE('',*,*,#3145,.F.);
#4761=ORIENTED_EDGE('',*,*,#3409,.T.);
#4762=ORIENTED_EDGE('',*,*,#3113,.T.);
#4763=ORIENTED_EDGE('',*,*,#3447,.T.);
#4764=ORIENTED_EDGE('',*,*,#3110,.F.);
#4765=ORIENTED_EDGE('',*,*,#3446,.T.);
#4766=ORIENTED_EDGE('',*,*,#3445,.T.);
#4767=ORIENTED_EDGE('',*,*,#3263,.T.);
#4768=ORIENTED_EDGE('',*,*,#3448,.T.);
#4769=ORIENTED_EDGE('',*,*,#3115,.F.);
#4770=ORIENTED_EDGE('',*,*,#3078,.T.);
#4771=ORIENTED_EDGE('',*,*,#3441,.T.);
#4772=ORIENTED_EDGE('',*,*,#3075,.F.);
#4773=ORIENTED_EDGE('',*,*,#3440,.T.);
#4774=ORIENTED_EDGE('',*,*,#3439,.T.);
#4775=ORIENTED_EDGE('',*,*,#3301,.T.);
#4776=ORIENTED_EDGE('',*,*,#3442,.T.);
#4777=ORIENTED_EDGE('',*,*,#3080,.F.);
#4778=ORIENTED_EDGE('',*,*,#3467,.F.);
#4779=ORIENTED_EDGE('',*,*,#3472,.T.);
#4780=ORIENTED_EDGE('',*,*,#3419,.F.);
#4781=ORIENTED_EDGE('',*,*,#3473,.F.);
#4782=ORIENTED_EDGE('',*,*,#3470,.F.);
#4783=ORIENTED_EDGE('',*,*,#3474,.T.);
#4784=ORIENTED_EDGE('',*,*,#3420,.F.);
#4785=ORIENTED_EDGE('',*,*,#3472,.F.);
#4786=ORIENTED_EDGE('',*,*,#3469,.F.);
#4787=ORIENTED_EDGE('',*,*,#3475,.T.);
#4788=ORIENTED_EDGE('',*,*,#3421,.F.);
#4789=ORIENTED_EDGE('',*,*,#3474,.F.);
#4790=ORIENTED_EDGE('',*,*,#3468,.F.);
#4791=ORIENTED_EDGE('',*,*,#3473,.T.);
#4792=ORIENTED_EDGE('',*,*,#3422,.F.);
#4793=ORIENTED_EDGE('',*,*,#3475,.F.);
#4794=ORIENTED_EDGE('',*,*,#3463,.F.);
#4795=ORIENTED_EDGE('',*,*,#3476,.T.);
#4796=ORIENTED_EDGE('',*,*,#3423,.F.);
#4797=ORIENTED_EDGE('',*,*,#3477,.F.);
#4798=ORIENTED_EDGE('',*,*,#3466,.F.);
#4799=ORIENTED_EDGE('',*,*,#3478,.T.);
#4800=ORIENTED_EDGE('',*,*,#3424,.F.);
#4801=ORIENTED_EDGE('',*,*,#3476,.F.);
#4802=ORIENTED_EDGE('',*,*,#3465,.F.);
#4803=ORIENTED_EDGE('',*,*,#3479,.T.);
#4804=ORIENTED_EDGE('',*,*,#3425,.F.);
#4805=ORIENTED_EDGE('',*,*,#3478,.F.);
#4806=ORIENTED_EDGE('',*,*,#3464,.F.);
#4807=ORIENTED_EDGE('',*,*,#3477,.T.);
#4808=ORIENTED_EDGE('',*,*,#3426,.F.);
#4809=ORIENTED_EDGE('',*,*,#3479,.F.);
#4810=ORIENTED_EDGE('',*,*,#3459,.F.);
#4811=ORIENTED_EDGE('',*,*,#3480,.T.);
#4812=ORIENTED_EDGE('',*,*,#3427,.F.);
#4813=ORIENTED_EDGE('',*,*,#3481,.F.);
#4814=ORIENTED_EDGE('',*,*,#3462,.F.);
#4815=ORIENTED_EDGE('',*,*,#3482,.T.);
#4816=ORIENTED_EDGE('',*,*,#3428,.F.);
#4817=ORIENTED_EDGE('',*,*,#3480,.F.);
#4818=ORIENTED_EDGE('',*,*,#3461,.F.);
#4819=ORIENTED_EDGE('',*,*,#3483,.T.);
#4820=ORIENTED_EDGE('',*,*,#3429,.F.);
#4821=ORIENTED_EDGE('',*,*,#3482,.F.);
#4822=ORIENTED_EDGE('',*,*,#3460,.F.);
#4823=ORIENTED_EDGE('',*,*,#3481,.T.);
#4824=ORIENTED_EDGE('',*,*,#3430,.F.);
#4825=ORIENTED_EDGE('',*,*,#3483,.F.);
#4826=ORIENTED_EDGE('',*,*,#3484,.F.);
#4827=ORIENTED_EDGE('',*,*,#3390,.F.);
#4828=ORIENTED_EDGE('',*,*,#3393,.F.);
#4829=ORIENTED_EDGE('',*,*,#3485,.F.);
#4830=ORIENTED_EDGE('',*,*,#3403,.T.);
#4831=ORIENTED_EDGE('',*,*,#3401,.T.);
#4832=ORIENTED_EDGE('',*,*,#3486,.F.);
#4833=ORIENTED_EDGE('',*,*,#3487,.F.);
#4834=ORIENTED_EDGE('',*,*,#3488,.F.);
#4835=ORIENTED_EDGE('',*,*,#3489,.F.);
#4836=ORIENTED_EDGE('',*,*,#3490,.F.);
#4837=ORIENTED_EDGE('',*,*,#3491,.F.);
#4838=ORIENTED_EDGE('',*,*,#3384,.F.);
#4839=ORIENTED_EDGE('',*,*,#3492,.F.);
#4840=ORIENTED_EDGE('',*,*,#3485,.T.);
#4841=ORIENTED_EDGE('',*,*,#3392,.T.);
#4842=ORIENTED_EDGE('',*,*,#3387,.F.);
#4843=ORIENTED_EDGE('',*,*,#3391,.F.);
#4844=ORIENTED_EDGE('',*,*,#3484,.T.);
#4845=ORIENTED_EDGE('',*,*,#3492,.T.);
#4846=ORIENTED_EDGE('',*,*,#3347,.F.);
#4847=ORIENTED_EDGE('',*,*,#3493,.F.);
#4848=ORIENTED_EDGE('',*,*,#3456,.F.);
#4849=ORIENTED_EDGE('',*,*,#3367,.T.);
#4850=ORIENTED_EDGE('',*,*,#3350,.F.);
#4851=ORIENTED_EDGE('',*,*,#3494,.F.);
#4852=ORIENTED_EDGE('',*,*,#3457,.F.);
#4853=ORIENTED_EDGE('',*,*,#3493,.T.);
#4854=ORIENTED_EDGE('',*,*,#3489,.T.);
#4855=ORIENTED_EDGE('',*,*,#3495,.F.);
#4856=ORIENTED_EDGE('',*,*,#3417,.T.);
#4857=ORIENTED_EDGE('',*,*,#3496,.T.);
#4858=ORIENTED_EDGE('',*,*,#3488,.T.);
#4859=ORIENTED_EDGE('',*,*,#3497,.F.);
#4860=ORIENTED_EDGE('',*,*,#3418,.T.);
#4861=ORIENTED_EDGE('',*,*,#3495,.T.);
#4862=ORIENTED_EDGE('',*,*,#3487,.T.);
#4863=ORIENTED_EDGE('',*,*,#3498,.F.);
#4864=ORIENTED_EDGE('',*,*,#3413,.T.);
#4865=ORIENTED_EDGE('',*,*,#3497,.T.);
#4866=ORIENTED_EDGE('',*,*,#3353,.F.);
#4867=ORIENTED_EDGE('',*,*,#3363,.F.);
#4868=ORIENTED_EDGE('',*,*,#3471,.F.);
#4869=ORIENTED_EDGE('',*,*,#3458,.F.);
#4870=ORIENTED_EDGE('',*,*,#3494,.T.);
#4871=ORIENTED_EDGE('',*,*,#3486,.T.);
#4872=ORIENTED_EDGE('',*,*,#3499,.F.);
#4873=ORIENTED_EDGE('',*,*,#3414,.T.);
#4874=ORIENTED_EDGE('',*,*,#3498,.T.);
#4875=ORIENTED_EDGE('',*,*,#3491,.T.);
#4876=ORIENTED_EDGE('',*,*,#3500,.F.);
#4877=ORIENTED_EDGE('',*,*,#3415,.T.);
#4878=ORIENTED_EDGE('',*,*,#3499,.T.);
#4879=ORIENTED_EDGE('',*,*,#3490,.T.);
#4880=ORIENTED_EDGE('',*,*,#3496,.F.);
#4881=ORIENTED_EDGE('',*,*,#3416,.T.);
#4882=ORIENTED_EDGE('',*,*,#3500,.T.);
#5831=CYLINDRICAL_SURFACE('',#6504,1.666);
#5832=CYLINDRICAL_SURFACE('',#6506,1.666);
#5833=CYLINDRICAL_SURFACE('',#6507,1.666);
#5834=CYLINDRICAL_SURFACE('',#6508,1.666);
#5835=CYLINDRICAL_SURFACE('',#6509,1.666);
#5836=CYLINDRICAL_SURFACE('',#6510,1.666);
#5837=CYLINDRICAL_SURFACE('',#6511,1.666);
#5838=CYLINDRICAL_SURFACE('',#6512,1.666);
#5839=CYLINDRICAL_SURFACE('',#6513,1.666);
#5840=CYLINDRICAL_SURFACE('',#6514,1.666);
#5841=CYLINDRICAL_SURFACE('',#6515,1.666);
#5842=CYLINDRICAL_SURFACE('',#6517,1.666);
#5843=CYLINDRICAL_SURFACE('',#6519,1.666);
#5844=CYLINDRICAL_SURFACE('',#6520,1.666);
#5845=CYLINDRICAL_SURFACE('',#6521,1.666);
#5846=CYLINDRICAL_SURFACE('',#6522,1.666);
#5847=CYLINDRICAL_SURFACE('',#6523,1.666);
#5848=CYLINDRICAL_SURFACE('',#6524,1.666);
#5849=CYLINDRICAL_SURFACE('',#6525,1.666);
#5850=CYLINDRICAL_SURFACE('',#6526,1.666);
#5851=CYLINDRICAL_SURFACE('',#6527,1.666);
#5852=CYLINDRICAL_SURFACE('',#6528,1.666);
#5853=CYLINDRICAL_SURFACE('',#6530,1.666);
#5854=CYLINDRICAL_SURFACE('',#6532,1.666);
#5855=CYLINDRICAL_SURFACE('',#6533,1.666);
#5856=CYLINDRICAL_SURFACE('',#6534,1.666);
#5857=CYLINDRICAL_SURFACE('',#6535,1.666);
#5858=CYLINDRICAL_SURFACE('',#6536,1.666);
#5859=CYLINDRICAL_SURFACE('',#6537,1.666);
#5860=CYLINDRICAL_SURFACE('',#6538,1.666);
#5861=CYLINDRICAL_SURFACE('',#6539,1.666);
#5862=CYLINDRICAL_SURFACE('',#6540,1.666);
#5863=CYLINDRICAL_SURFACE('',#6541,1.666);
#5864=CYLINDRICAL_SURFACE('',#6544,1.666);
#5865=CYLINDRICAL_SURFACE('',#6546,1.666);
#5866=CYLINDRICAL_SURFACE('',#6547,1.666);
#5867=CYLINDRICAL_SURFACE('',#6548,1.666);
#5868=CYLINDRICAL_SURFACE('',#6549,1.666);
#5869=CYLINDRICAL_SURFACE('',#6550,1.666);
#5870=CYLINDRICAL_SURFACE('',#6551,1.666);
#5871=CYLINDRICAL_SURFACE('',#6552,1.666);
#5872=CYLINDRICAL_SURFACE('',#6553,1.666);
#5873=CYLINDRICAL_SURFACE('',#6554,1.666);
#5874=CYLINDRICAL_SURFACE('',#6555,1.666);
#5875=CYLINDRICAL_SURFACE('',#6558,2.05475);
#5876=CYLINDRICAL_SURFACE('',#6560,2.05475);
#5877=CYLINDRICAL_SURFACE('',#6561,2.05475);
#5878=CYLINDRICAL_SURFACE('',#6562,2.05475);
#5879=CYLINDRICAL_SURFACE('',#6563,2.05475);
#5880=CYLINDRICAL_SURFACE('',#6564,2.05475);
#5881=CYLINDRICAL_SURFACE('',#6565,2.05475);
#5882=CYLINDRICAL_SURFACE('',#6566,2.05475);
#5883=CYLINDRICAL_SURFACE('',#6567,2.05475);
#5884=CYLINDRICAL_SURFACE('',#6568,2.05475);
#5885=CYLINDRICAL_SURFACE('',#6569,2.05475);
#5886=CYLINDRICAL_SURFACE('',#6570,2.05475);
#5887=CYLINDRICAL_SURFACE('',#6572,2.05475);
#5888=CYLINDRICAL_SURFACE('',#6574,2.05475);
#5889=CYLINDRICAL_SURFACE('',#6575,2.05475);
#5890=CYLINDRICAL_SURFACE('',#6576,2.05475);
#5891=CYLINDRICAL_SURFACE('',#6577,2.05475);
#5892=CYLINDRICAL_SURFACE('',#6578,2.05475);
#5893=CYLINDRICAL_SURFACE('',#6579,2.05475);
#5894=CYLINDRICAL_SURFACE('',#6580,2.05475);
#5895=CYLINDRICAL_SURFACE('',#6581,2.05475);
#5896=CYLINDRICAL_SURFACE('',#6582,2.05475);
#5897=CYLINDRICAL_SURFACE('',#6583,2.05475);
#5898=CYLINDRICAL_SURFACE('',#6584,2.05475);
#5899=CYLINDRICAL_SURFACE('',#6586,2.05475);
#5900=CYLINDRICAL_SURFACE('',#6588,2.05475);
#5901=CYLINDRICAL_SURFACE('',#6589,2.05475);
#5902=CYLINDRICAL_SURFACE('',#6590,2.05475);
#5903=CYLINDRICAL_SURFACE('',#6591,2.05475);
#5904=CYLINDRICAL_SURFACE('',#6592,2.05475);
#5905=CYLINDRICAL_SURFACE('',#6593,2.05475);
#5906=CYLINDRICAL_SURFACE('',#6594,2.05475);
#5907=CYLINDRICAL_SURFACE('',#6595,2.05475);
#5908=CYLINDRICAL_SURFACE('',#6596,2.05475);
#5909=CYLINDRICAL_SURFACE('',#6597,2.05475);
#5910=CYLINDRICAL_SURFACE('',#6598,2.05475);
#5911=CYLINDRICAL_SURFACE('',#6600,2.05475);
#5912=CYLINDRICAL_SURFACE('',#6602,2.05475);
#5913=CYLINDRICAL_SURFACE('',#6603,2.05475);
#5914=CYLINDRICAL_SURFACE('',#6604,2.05475);
#5915=CYLINDRICAL_SURFACE('',#6605,2.05475);
#5916=CYLINDRICAL_SURFACE('',#6606,2.05475);
#5917=CYLINDRICAL_SURFACE('',#6607,2.05475);
#5918=CYLINDRICAL_SURFACE('',#6608,2.05475);
#5919=CYLINDRICAL_SURFACE('',#6609,2.05475);
#5920=CYLINDRICAL_SURFACE('',#6610,2.05475);
#5921=CYLINDRICAL_SURFACE('',#6611,2.05475);
#5922=CYLINDRICAL_SURFACE('',#6612,2.05475);
#5923=CYLINDRICAL_SURFACE('',#6614,2.);
#5924=CYLINDRICAL_SURFACE('',#6617,2.);
#5925=CYLINDRICAL_SURFACE('',#6619,2.);
#5926=CYLINDRICAL_SURFACE('',#6621,2.);
#5927=CYLINDRICAL_SURFACE('',#6623,2.);
#5928=CYLINDRICAL_SURFACE('',#6625,2.);
#5929=CYLINDRICAL_SURFACE('',#6633,2.);
#5930=CYLINDRICAL_SURFACE('',#6636,2.);
#5931=CYLINDRICAL_SURFACE('',#6638,2.);
#5932=CYLINDRICAL_SURFACE('',#6640,2.);
#5933=CYLINDRICAL_SURFACE('',#6651,3.5);
#5934=CYLINDRICAL_SURFACE('',#6653,3.5);
#5935=CYLINDRICAL_SURFACE('',#6655,2.05475);
#5936=CYLINDRICAL_SURFACE('',#6657,2.05475);
#5937=CYLINDRICAL_SURFACE('',#6658,2.05475);
#5938=CYLINDRICAL_SURFACE('',#6659,2.05475);
#5939=CYLINDRICAL_SURFACE('',#6662,1.666);
#5940=CYLINDRICAL_SURFACE('',#6664,1.666);
#5941=CYLINDRICAL_SURFACE('',#6665,1.666);
#5942=CYLINDRICAL_SURFACE('',#6667,1.666);
#6035=ADVANCED_FACE('',(#323),#5831,.F.);
#6036=ADVANCED_FACE('',(#324),#5832,.F.);
#6037=ADVANCED_FACE('',(#325),#5833,.F.);
#6038=ADVANCED_FACE('',(#326),#5834,.F.);
#6039=ADVANCED_FACE('',(#327),#5835,.F.);
#6040=ADVANCED_FACE('',(#328),#5836,.F.);
#6041=ADVANCED_FACE('',(#329),#5837,.F.);
#6042=ADVANCED_FACE('',(#330),#5838,.F.);
#6043=ADVANCED_FACE('',(#331),#5839,.F.);
#6044=ADVANCED_FACE('',(#332),#5840,.F.);
#6045=ADVANCED_FACE('',(#333),#5841,.F.);
#6046=ADVANCED_FACE('',(#334),#5842,.F.);
#6047=ADVANCED_FACE('',(#335),#5843,.F.);
#6048=ADVANCED_FACE('',(#336),#5844,.F.);
#6049=ADVANCED_FACE('',(#337),#5845,.F.);
#6050=ADVANCED_FACE('',(#338),#5846,.F.);
#6051=ADVANCED_FACE('',(#339),#5847,.F.);
#6052=ADVANCED_FACE('',(#340),#5848,.F.);
#6053=ADVANCED_FACE('',(#341),#5849,.F.);
#6054=ADVANCED_FACE('',(#342),#5850,.F.);
#6055=ADVANCED_FACE('',(#343),#5851,.F.);
#6056=ADVANCED_FACE('',(#344),#5852,.F.);
#6057=ADVANCED_FACE('',(#345),#5853,.F.);
#6058=ADVANCED_FACE('',(#346),#5854,.F.);
#6059=ADVANCED_FACE('',(#347),#5855,.F.);
#6060=ADVANCED_FACE('',(#348),#5856,.F.);
#6061=ADVANCED_FACE('',(#349),#5857,.F.);
#6062=ADVANCED_FACE('',(#350),#5858,.F.);
#6063=ADVANCED_FACE('',(#351),#5859,.F.);
#6064=ADVANCED_FACE('',(#352),#5860,.F.);
#6065=ADVANCED_FACE('',(#353),#5861,.F.);
#6066=ADVANCED_FACE('',(#354),#5862,.F.);
#6067=ADVANCED_FACE('',(#355),#5863,.F.);
#6068=ADVANCED_FACE('',(#356),#5864,.F.);
#6069=ADVANCED_FACE('',(#357),#5865,.F.);
#6070=ADVANCED_FACE('',(#358),#5866,.F.);
#6071=ADVANCED_FACE('',(#359),#5867,.F.);
#6072=ADVANCED_FACE('',(#360),#5868,.F.);
#6073=ADVANCED_FACE('',(#361),#5869,.F.);
#6074=ADVANCED_FACE('',(#362),#5870,.F.);
#6075=ADVANCED_FACE('',(#363),#5871,.F.);
#6076=ADVANCED_FACE('',(#364),#5872,.F.);
#6077=ADVANCED_FACE('',(#365),#5873,.F.);
#6078=ADVANCED_FACE('',(#366),#5874,.F.);
#6079=ADVANCED_FACE('',(#367),#5875,.F.);
#6080=ADVANCED_FACE('',(#368),#5876,.F.);
#6081=ADVANCED_FACE('',(#369),#5877,.F.);
#6082=ADVANCED_FACE('',(#370),#5878,.F.);
#6083=ADVANCED_FACE('',(#371),#5879,.F.);
#6084=ADVANCED_FACE('',(#372),#5880,.F.);
#6085=ADVANCED_FACE('',(#373),#5881,.F.);
#6086=ADVANCED_FACE('',(#374),#5882,.F.);
#6087=ADVANCED_FACE('',(#375),#5883,.F.);
#6088=ADVANCED_FACE('',(#376),#5884,.F.);
#6089=ADVANCED_FACE('',(#377),#5885,.F.);
#6090=ADVANCED_FACE('',(#378),#5886,.F.);
#6091=ADVANCED_FACE('',(#379),#5887,.F.);
#6092=ADVANCED_FACE('',(#380),#5888,.F.);
#6093=ADVANCED_FACE('',(#381),#5889,.F.);
#6094=ADVANCED_FACE('',(#382),#5890,.F.);
#6095=ADVANCED_FACE('',(#383),#5891,.F.);
#6096=ADVANCED_FACE('',(#384),#5892,.F.);
#6097=ADVANCED_FACE('',(#385),#5893,.F.);
#6098=ADVANCED_FACE('',(#386),#5894,.F.);
#6099=ADVANCED_FACE('',(#387),#5895,.F.);
#6100=ADVANCED_FACE('',(#388),#5896,.F.);
#6101=ADVANCED_FACE('',(#389),#5897,.F.);
#6102=ADVANCED_FACE('',(#390),#5898,.F.);
#6103=ADVANCED_FACE('',(#391),#5899,.F.);
#6104=ADVANCED_FACE('',(#392),#5900,.F.);
#6105=ADVANCED_FACE('',(#393),#5901,.F.);
#6106=ADVANCED_FACE('',(#394),#5902,.F.);
#6107=ADVANCED_FACE('',(#395),#5903,.F.);
#6108=ADVANCED_FACE('',(#396),#5904,.F.);
#6109=ADVANCED_FACE('',(#397),#5905,.F.);
#6110=ADVANCED_FACE('',(#398),#5906,.F.);
#6111=ADVANCED_FACE('',(#399),#5907,.F.);
#6112=ADVANCED_FACE('',(#400),#5908,.F.);
#6113=ADVANCED_FACE('',(#401),#5909,.F.);
#6114=ADVANCED_FACE('',(#402),#5910,.F.);
#6115=ADVANCED_FACE('',(#403),#5911,.F.);
#6116=ADVANCED_FACE('',(#404),#5912,.F.);
#6117=ADVANCED_FACE('',(#405),#5913,.F.);
#6118=ADVANCED_FACE('',(#406),#5914,.F.);
#6119=ADVANCED_FACE('',(#407),#5915,.F.);
#6120=ADVANCED_FACE('',(#408),#5916,.F.);
#6121=ADVANCED_FACE('',(#409),#5917,.F.);
#6122=ADVANCED_FACE('',(#410),#5918,.F.);
#6123=ADVANCED_FACE('',(#411),#5919,.F.);
#6124=ADVANCED_FACE('',(#412),#5920,.F.);
#6125=ADVANCED_FACE('',(#413),#5921,.F.);
#6126=ADVANCED_FACE('',(#414),#5922,.F.);
#6127=ADVANCED_FACE('',(#415),#5923,.T.);
#6128=ADVANCED_FACE('',(#416),#5924,.T.);
#6129=ADVANCED_FACE('',(#417),#5925,.T.);
#6130=ADVANCED_FACE('',(#418),#5926,.T.);
#6131=ADVANCED_FACE('',(#419),#5927,.T.);
#6132=ADVANCED_FACE('',(#420),#5928,.T.);
#6133=ADVANCED_FACE('',(#421),#197,.T.);
#6134=ADVANCED_FACE('',(#422),#198,.T.);
#6135=ADVANCED_FACE('',(#423),#199,.T.);
#6136=ADVANCED_FACE('',(#424,#145),#200,.T.);
#6137=ADVANCED_FACE('',(#425),#5929,.T.);
#6138=ADVANCED_FACE('',(#426),#5930,.T.);
#6139=ADVANCED_FACE('',(#427),#5931,.T.);
#6140=ADVANCED_FACE('',(#428),#5932,.T.);
#6141=ADVANCED_FACE('',(#429),#201,.T.);
#6142=ADVANCED_FACE('',(#430),#202,.T.);
#6143=ADVANCED_FACE('',(#431),#143,.T.);
#6144=ADVANCED_FACE('',(#432),#144,.T.);
#6145=ADVANCED_FACE('',(#433),#5933,.F.);
#6146=ADVANCED_FACE('',(#434),#5934,.F.);
#6147=ADVANCED_FACE('',(#435),#5935,.F.);
#6148=ADVANCED_FACE('',(#436),#129,.F.);
#6149=ADVANCED_FACE('',(#437),#130,.F.);
#6150=ADVANCED_FACE('',(#438,#146,#147,#148,#149,#150,#151,#152),#203,.F.);
#6151=ADVANCED_FACE('',(#439),#5936,.F.);
#6152=ADVANCED_FACE('',(#440),#131,.F.);
#6153=ADVANCED_FACE('',(#441),#132,.F.);
#6154=ADVANCED_FACE('',(#442),#5937,.F.);
#6155=ADVANCED_FACE('',(#443),#133,.F.);
#6156=ADVANCED_FACE('',(#444),#134,.F.);
#6157=ADVANCED_FACE('',(#445),#5938,.F.);
#6158=ADVANCED_FACE('',(#446),#135,.F.);
#6159=ADVANCED_FACE('',(#447),#136,.F.);
#6160=ADVANCED_FACE('',(#448,#153,#154,#155),#204,.T.);
#6161=ADVANCED_FACE('',(#449),#205,.F.);
#6162=ADVANCED_FACE('',(#450),#5939,.F.);
#6163=ADVANCED_FACE('',(#451),#206,.F.);
#6164=ADVANCED_FACE('',(#452),#5940,.F.);
#6165=ADVANCED_FACE('',(#453),#5941,.F.);
#6166=ADVANCED_FACE('',(#454),#207,.F.);
#6167=ADVANCED_FACE('',(#455),#5942,.F.);
#6168=ADVANCED_FACE('',(#456),#208,.F.);
#6169=ADVANCED_FACE('',(#457),#209,.F.);
#6170=ADVANCED_FACE('',(#458),#210,.F.);
#6171=ADVANCED_FACE('',(#459),#211,.F.);
#6172=ADVANCED_FACE('',(#460),#212,.F.);
#6173=ADVANCED_FACE('',(#461),#213,.F.);
#6174=ADVANCED_FACE('',(#462),#214,.F.);
#6175=ADVANCED_FACE('',(#463),#215,.F.);
#6176=ADVANCED_FACE('',(#464),#216,.F.);
#6177=ADVANCED_FACE('',(#465),#217,.F.);
#6178=ADVANCED_FACE('',(#466),#218,.F.);
#6179=ADVANCED_FACE('',(#467),#219,.F.);
#6180=ADVANCED_FACE('',(#468),#220,.F.);
#6181=ADVANCED_FACE('',(#469,#156,#157,#158),#221,.F.);
#6182=ADVANCED_FACE('',(#470),#222,.T.);
#6183=ADVANCED_FACE('',(#471),#223,.T.);
#6184=ADVANCED_FACE('',(#472),#224,.T.);
#6185=ADVANCED_FACE('',(#473),#225,.T.);
#6186=ADVANCED_FACE('',(#474),#226,.T.);
#6187=ADVANCED_FACE('',(#475),#227,.T.);
#6188=ADVANCED_FACE('',(#476),#228,.T.);
#6189=ADVANCED_FACE('',(#477),#229,.T.);
#6190=ADVANCED_FACE('',(#478),#230,.T.);
#6191=ADVANCED_FACE('',(#479),#231,.T.);
#6192=ADVANCED_FACE('',(#480),#232,.T.);
#6381=CLOSED_SHELL('',(#6035,#6036,#6037,#6038,#6039,#6040,#6041,#6042,
#6043,#6044,#6045,#6046,#6047,#6048,#6049,#6050,#6051,#6052,#6053,#6054,
#6055,#6056,#6057,#6058,#6059,#6060,#6061,#6062,#6063,#6064,#6065,#6066,
#6067,#6068,#6069,#6070,#6071,#6072,#6073,#6074,#6075,#6076,#6077,#6078,
#6079,#6080,#6081,#6082,#6083,#6084,#6085,#6086,#6087,#6088,#6089,#6090,
#6091,#6092,#6093,#6094,#6095,#6096,#6097,#6098,#6099,#6100,#6101,#6102,
#6103,#6104,#6105,#6106,#6107,#6108,#6109,#6110,#6111,#6112,#6113,#6114,
#6115,#6116,#6117,#6118,#6119,#6120,#6121,#6122,#6123,#6124,#6125,#6126,
#6127,#6128,#6129,#6130,#6131,#6132,#6133,#6134,#6135,#6136,#6137,#6138,
#6139,#6140,#6141,#6142,#6143,#6144,#6145,#6146,#6147,#6148,#6149,#6150,
#6151,#6152,#6153,#6154,#6155,#6156,#6157,#6158,#6159,#6160,#6161,#6162,
#6163,#6164,#6165,#6166,#6167,#6168,#6169,#6170,#6171,#6172,#6173,#6174,
#6175,#6176,#6177,#6178,#6179,#6180,#6181,#6182,#6183,#6184,#6185,#6186,
#6187,#6188,#6189,#6190,#6191,#6192));
#6503=AXIS2_PLACEMENT_3D('',#8354,#6969,#6970);
#6504=AXIS2_PLACEMENT_3D('',#8355,#6971,#6972);
#6505=AXIS2_PLACEMENT_3D('',#8374,#6974,#6975);
#6506=AXIS2_PLACEMENT_3D('',#8394,#6976,#6977);
#6507=AXIS2_PLACEMENT_3D('',#8442,#6979,#6980);
#6508=AXIS2_PLACEMENT_3D('',#8490,#6982,#6983);
#6509=AXIS2_PLACEMENT_3D('',#8541,#6985,#6986);
#6510=AXIS2_PLACEMENT_3D('',#8589,#6988,#6989);
#6511=AXIS2_PLACEMENT_3D('',#8637,#6991,#6992);
#6512=AXIS2_PLACEMENT_3D('',#8688,#6994,#6995);
#6513=AXIS2_PLACEMENT_3D('',#8739,#6997,#6998);
#6514=AXIS2_PLACEMENT_3D('',#8787,#7000,#7001);
#6515=AXIS2_PLACEMENT_3D('',#8838,#7003,#7004);
#6516=AXIS2_PLACEMENT_3D('',#8857,#7006,#7007);
#6517=AXIS2_PLACEMENT_3D('',#8877,#7008,#7009);
#6518=AXIS2_PLACEMENT_3D('',#8896,#7011,#7012);
#6519=AXIS2_PLACEMENT_3D('',#8916,#7013,#7014);
#6520=AXIS2_PLACEMENT_3D('',#8964,#7016,#7017);
#6521=AXIS2_PLACEMENT_3D('',#9012,#7019,#7020);
#6522=AXIS2_PLACEMENT_3D('',#9063,#7022,#7023);
#6523=AXIS2_PLACEMENT_3D('',#9111,#7025,#7026);
#6524=AXIS2_PLACEMENT_3D('',#9159,#7028,#7029);
#6525=AXIS2_PLACEMENT_3D('',#9210,#7031,#7032);
#6526=AXIS2_PLACEMENT_3D('',#9261,#7034,#7035);
#6527=AXIS2_PLACEMENT_3D('',#9309,#7037,#7038);
#6528=AXIS2_PLACEMENT_3D('',#9360,#7040,#7041);
#6529=AXIS2_PLACEMENT_3D('',#9379,#7043,#7044);
#6530=AXIS2_PLACEMENT_3D('',#9399,#7045,#7046);
#6531=AXIS2_PLACEMENT_3D('',#9418,#7048,#7049);
#6532=AXIS2_PLACEMENT_3D('',#9438,#7050,#7051);
#6533=AXIS2_PLACEMENT_3D('',#9486,#7053,#7054);
#6534=AXIS2_PLACEMENT_3D('',#9534,#7056,#7057);
#6535=AXIS2_PLACEMENT_3D('',#9585,#7059,#7060);
#6536=AXIS2_PLACEMENT_3D('',#9633,#7062,#7063);
#6537=AXIS2_PLACEMENT_3D('',#9681,#7065,#7066);
#6538=AXIS2_PLACEMENT_3D('',#9732,#7068,#7069);
#6539=AXIS2_PLACEMENT_3D('',#9783,#7071,#7072);
#6540=AXIS2_PLACEMENT_3D('',#9831,#7074,#7075);
#6541=AXIS2_PLACEMENT_3D('',#9882,#7077,#7078);
#6542=AXIS2_PLACEMENT_3D('',#9901,#7080,#7081);
#6543=AXIS2_PLACEMENT_3D('',#9903,#7082,#7083);
#6544=AXIS2_PLACEMENT_3D('',#9923,#7084,#7085);
#6545=AXIS2_PLACEMENT_3D('',#9942,#7087,#7088);
#6546=AXIS2_PLACEMENT_3D('',#9962,#7089,#7090);
#6547=AXIS2_PLACEMENT_3D('',#10010,#7092,#7093);
#6548=AXIS2_PLACEMENT_3D('',#10058,#7095,#7096);
#6549=AXIS2_PLACEMENT_3D('',#10109,#7098,#7099);
#6550=AXIS2_PLACEMENT_3D('',#10157,#7101,#7102);
#6551=AXIS2_PLACEMENT_3D('',#10205,#7104,#7105);
#6552=AXIS2_PLACEMENT_3D('',#10256,#7107,#7108);
#6553=AXIS2_PLACEMENT_3D('',#10307,#7110,#7111);
#6554=AXIS2_PLACEMENT_3D('',#10355,#7113,#7114);
#6555=AXIS2_PLACEMENT_3D('',#10406,#7116,#7117);
#6556=AXIS2_PLACEMENT_3D('',#10425,#7119,#7120);
#6557=AXIS2_PLACEMENT_3D('',#10427,#7121,#7122);
#6558=AXIS2_PLACEMENT_3D('',#10447,#7123,#7124);
#6559=AXIS2_PLACEMENT_3D('',#10457,#7126,#7127);
#6560=AXIS2_PLACEMENT_3D('',#10463,#7128,#7129);
#6561=AXIS2_PLACEMENT_3D('',#10488,#7131,#7132);
#6562=AXIS2_PLACEMENT_3D('',#10513,#7134,#7135);
#6563=AXIS2_PLACEMENT_3D('',#10537,#7137,#7138);
#6564=AXIS2_PLACEMENT_3D('',#10562,#7140,#7141);
#6565=AXIS2_PLACEMENT_3D('',#10586,#7143,#7144);
#6566=AXIS2_PLACEMENT_3D('',#10611,#7146,#7147);
#6567=AXIS2_PLACEMENT_3D('',#10635,#7149,#7150);
#6568=AXIS2_PLACEMENT_3D('',#10660,#7152,#7153);
#6569=AXIS2_PLACEMENT_3D('',#10685,#7155,#7156);
#6570=AXIS2_PLACEMENT_3D('',#10709,#7158,#7159);
#6571=AXIS2_PLACEMENT_3D('',#10720,#7161,#7162);
#6572=AXIS2_PLACEMENT_3D('',#10726,#7163,#7164);
#6573=AXIS2_PLACEMENT_3D('',#10736,#7166,#7167);
#6574=AXIS2_PLACEMENT_3D('',#10742,#7168,#7169);
#6575=AXIS2_PLACEMENT_3D('',#10767,#7171,#7172);
#6576=AXIS2_PLACEMENT_3D('',#10792,#7174,#7175);
#6577=AXIS2_PLACEMENT_3D('',#10816,#7177,#7178);
#6578=AXIS2_PLACEMENT_3D('',#10841,#7180,#7181);
#6579=AXIS2_PLACEMENT_3D('',#10865,#7183,#7184);
#6580=AXIS2_PLACEMENT_3D('',#10890,#7186,#7187);
#6581=AXIS2_PLACEMENT_3D('',#10914,#7189,#7190);
#6582=AXIS2_PLACEMENT_3D('',#10939,#7192,#7193);
#6583=AXIS2_PLACEMENT_3D('',#10964,#7195,#7196);
#6584=AXIS2_PLACEMENT_3D('',#10988,#7198,#7199);
#6585=AXIS2_PLACEMENT_3D('',#10999,#7201,#7202);
#6586=AXIS2_PLACEMENT_3D('',#11005,#7203,#7204);
#6587=AXIS2_PLACEMENT_3D('',#11015,#7206,#7207);
#6588=AXIS2_PLACEMENT_3D('',#11021,#7208,#7209);
#6589=AXIS2_PLACEMENT_3D('',#11046,#7211,#7212);
#6590=AXIS2_PLACEMENT_3D('',#11071,#7214,#7215);
#6591=AXIS2_PLACEMENT_3D('',#11095,#7217,#7218);
#6592=AXIS2_PLACEMENT_3D('',#11120,#7220,#7221);
#6593=AXIS2_PLACEMENT_3D('',#11144,#7223,#7224);
#6594=AXIS2_PLACEMENT_3D('',#11169,#7226,#7227);
#6595=AXIS2_PLACEMENT_3D('',#11193,#7229,#7230);
#6596=AXIS2_PLACEMENT_3D('',#11218,#7232,#7233);
#6597=AXIS2_PLACEMENT_3D('',#11243,#7235,#7236);
#6598=AXIS2_PLACEMENT_3D('',#11267,#7238,#7239);
#6599=AXIS2_PLACEMENT_3D('',#11278,#7241,#7242);
#6600=AXIS2_PLACEMENT_3D('',#11284,#7243,#7244);
#6601=AXIS2_PLACEMENT_3D('',#11294,#7246,#7247);
#6602=AXIS2_PLACEMENT_3D('',#11300,#7248,#7249);
#6603=AXIS2_PLACEMENT_3D('',#11325,#7251,#7252);
#6604=AXIS2_PLACEMENT_3D('',#11350,#7254,#7255);
#6605=AXIS2_PLACEMENT_3D('',#11374,#7257,#7258);
#6606=AXIS2_PLACEMENT_3D('',#11399,#7260,#7261);
#6607=AXIS2_PLACEMENT_3D('',#11423,#7263,#7264);
#6608=AXIS2_PLACEMENT_3D('',#11448,#7266,#7267);
#6609=AXIS2_PLACEMENT_3D('',#11472,#7269,#7270);
#6610=AXIS2_PLACEMENT_3D('',#11497,#7272,#7273);
#6611=AXIS2_PLACEMENT_3D('',#11522,#7275,#7276);
#6612=AXIS2_PLACEMENT_3D('',#11546,#7278,#7279);
#6613=AXIS2_PLACEMENT_3D('',#11557,#7281,#7282);
#6614=AXIS2_PLACEMENT_3D('',#11563,#7283,#7284);
#6615=AXIS2_PLACEMENT_3D('',#11568,#7286,#7287);
#6616=AXIS2_PLACEMENT_3D('',#11571,#7289,#7290);
#6617=AXIS2_PLACEMENT_3D('',#11572,#7291,#7292);
#6618=AXIS2_PLACEMENT_3D('',#11576,#7294,#7295);
#6619=AXIS2_PLACEMENT_3D('',#11578,#7297,#7298);
#6620=AXIS2_PLACEMENT_3D('',#11582,#7300,#7301);
#6621=AXIS2_PLACEMENT_3D('',#11584,#7303,#7304);
#6622=AXIS2_PLACEMENT_3D('',#11588,#7306,#7307);
#6623=AXIS2_PLACEMENT_3D('',#11590,#7309,#7310);
#6624=AXIS2_PLACEMENT_3D('',#11595,#7313,#7314);
#6625=AXIS2_PLACEMENT_3D('',#11596,#7315,#7316);
#6626=AXIS2_PLACEMENT_3D('',#11599,#7319,#7320);
#6627=AXIS2_PLACEMENT_3D('',#11609,#7326,#7327);
#6628=AXIS2_PLACEMENT_3D('',#11614,#7331,#7332);
#6629=AXIS2_PLACEMENT_3D('',#11618,#7335,#7336);
#6630=AXIS2_PLACEMENT_3D('',#11623,#7338,#7339);
#6631=AXIS2_PLACEMENT_3D('',#11631,#7343,#7344);
#6632=AXIS2_PLACEMENT_3D('',#11633,#7345,#7346);
#6633=AXIS2_PLACEMENT_3D('',#11637,#7349,#7350);
#6634=AXIS2_PLACEMENT_3D('',#11660,#7351,#7352);
#6635=AXIS2_PLACEMENT_3D('',#11663,#7354,#7355);
#6636=AXIS2_PLACEMENT_3D('',#11664,#7356,#7357);
#6637=AXIS2_PLACEMENT_3D('',#11666,#7358,#7359);
#6638=AXIS2_PLACEMENT_3D('',#11668,#7361,#7362);
#6639=AXIS2_PLACEMENT_3D('',#11688,#7363,#7364);
#6640=AXIS2_PLACEMENT_3D('',#11690,#7366,#7367);
#6641=AXIS2_PLACEMENT_3D('',#11692,#7369,#7370);
#6642=AXIS2_PLACEMENT_3D('',#11698,#7374,#7375);
#6643=AXIS2_PLACEMENT_3D('',#11702,#7378,#7379);
#6644=AXIS2_PLACEMENT_3D('',#11704,#7380,#7381);
#6645=AXIS2_PLACEMENT_3D('',#11706,#7382,#7383);
#6646=AXIS2_PLACEMENT_3D('',#11707,#7384,#7385);
#6647=AXIS2_PLACEMENT_3D('',#11708,#7386,#7387);
#6648=AXIS2_PLACEMENT_3D('',#11710,#7388,#7389);
#6649=AXIS2_PLACEMENT_3D('',#11712,#7390,#7391);
#6650=AXIS2_PLACEMENT_3D('',#11713,#7392,#7393);
#6651=AXIS2_PLACEMENT_3D('',#11714,#7394,#7395);
#6652=AXIS2_PLACEMENT_3D('',#11717,#7397,#7398);
#6653=AXIS2_PLACEMENT_3D('',#11718,#7399,#7400);
#6654=AXIS2_PLACEMENT_3D('',#11721,#7402,#7403);
#6655=AXIS2_PLACEMENT_3D('',#11722,#7404,#7405);
#6656=AXIS2_PLACEMENT_3D('',#12745,#7406,#7407);
#6657=AXIS2_PLACEMENT_3D('',#13283,#7426,#7427);
#6658=AXIS2_PLACEMENT_3D('',#14141,#7428,#7429);
#6659=AXIS2_PLACEMENT_3D('',#14999,#7430,#7431);
#6660=AXIS2_PLACEMENT_3D('',#15861,#7432,#7433);
#6661=AXIS2_PLACEMENT_3D('',#15891,#7449,#7450);
#6662=AXIS2_PLACEMENT_3D('',#15892,#7451,#7452);
#6663=AXIS2_PLACEMENT_3D('',#15893,#7453,#7454);
#6664=AXIS2_PLACEMENT_3D('',#15895,#7456,#7457);
#6665=AXIS2_PLACEMENT_3D('',#15896,#7458,#7459);
#6666=AXIS2_PLACEMENT_3D('',#15897,#7460,#7461);
#6667=AXIS2_PLACEMENT_3D('',#15898,#7462,#7463);
#6668=AXIS2_PLACEMENT_3D('',#15899,#7464,#7465);
#6669=AXIS2_PLACEMENT_3D('',#15900,#7466,#7467);
#6670=AXIS2_PLACEMENT_3D('',#15903,#7470,#7471);
#6671=AXIS2_PLACEMENT_3D('',#15905,#7473,#7474);
#6672=AXIS2_PLACEMENT_3D('',#15907,#7476,#7477);
#6673=AXIS2_PLACEMENT_3D('',#15908,#7478,#7479);
#6674=AXIS2_PLACEMENT_3D('',#15911,#7482,#7483);
#6675=AXIS2_PLACEMENT_3D('',#15913,#7485,#7486);
#6676=AXIS2_PLACEMENT_3D('',#15915,#7488,#7489);
#6677=AXIS2_PLACEMENT_3D('',#15916,#7490,#7491);
#6678=AXIS2_PLACEMENT_3D('',#15919,#7494,#7495);
#6679=AXIS2_PLACEMENT_3D('',#15921,#7497,#7498);
#6680=AXIS2_PLACEMENT_3D('',#15923,#7500,#7501);
#6681=AXIS2_PLACEMENT_3D('',#15924,#7502,#7503);
#6682=AXIS2_PLACEMENT_3D('',#15940,#7512,#7513);
#6683=AXIS2_PLACEMENT_3D('',#15942,#7515,#7516);
#6684=AXIS2_PLACEMENT_3D('',#15943,#7517,#7518);
#6685=AXIS2_PLACEMENT_3D('',#15945,#7520,#7521);
#6686=AXIS2_PLACEMENT_3D('',#15947,#7523,#7524);
#6687=AXIS2_PLACEMENT_3D('',#15950,#7527,#7528);
#6688=AXIS2_PLACEMENT_3D('',#15952,#7530,#7531);
#6689=AXIS2_PLACEMENT_3D('',#15954,#7533,#7534);
#6690=AXIS2_PLACEMENT_3D('',#15955,#7535,#7536);
#6691=AXIS2_PLACEMENT_3D('',#15957,#7538,#7539);
#6692=AXIS2_PLACEMENT_3D('',#15959,#7541,#7542);
#6969=DIRECTION('axis',(0.,0.,1.));
#6970=DIRECTION('refdir',(1.,0.,0.));
#6971=DIRECTION('center_axis',(0.,0.,-1.));
#6972=DIRECTION('ref_axis',(1.,0.,0.));
#6973=DIRECTION('',(0.,0.,-1.));
#6974=DIRECTION('center_axis',(0.,0.,-1.));
#6975=DIRECTION('ref_axis',(1.,0.,0.));
#6976=DIRECTION('center_axis',(0.,0.,-1.));
#6977=DIRECTION('ref_axis',(1.,0.,0.));
#6978=DIRECTION('',(0.,0.,-1.));
#6979=DIRECTION('center_axis',(0.,0.,-1.));
#6980=DIRECTION('ref_axis',(1.,0.,0.));
#6981=DIRECTION('',(0.,0.,-1.));
#6982=DIRECTION('center_axis',(0.,0.,-1.));
#6983=DIRECTION('ref_axis',(1.,0.,0.));
#6984=DIRECTION('',(0.,0.,-1.));
#6985=DIRECTION('center_axis',(0.,0.,-1.));
#6986=DIRECTION('ref_axis',(1.,0.,0.));
#6987=DIRECTION('',(0.,0.,-1.));
#6988=DIRECTION('center_axis',(0.,0.,-1.));
#6989=DIRECTION('ref_axis',(1.,0.,0.));
#6990=DIRECTION('',(0.,0.,-1.));
#6991=DIRECTION('center_axis',(0.,0.,-1.));
#6992=DIRECTION('ref_axis',(1.,0.,0.));
#6993=DIRECTION('',(0.,0.,-1.));
#6994=DIRECTION('center_axis',(0.,0.,-1.));
#6995=DIRECTION('ref_axis',(1.,0.,0.));
#6996=DIRECTION('',(0.,0.,-1.));
#6997=DIRECTION('center_axis',(0.,0.,-1.));
#6998=DIRECTION('ref_axis',(1.,0.,0.));
#6999=DIRECTION('',(0.,0.,-1.));
#7000=DIRECTION('center_axis',(0.,0.,-1.));
#7001=DIRECTION('ref_axis',(1.,0.,0.));
#7002=DIRECTION('',(0.,0.,-1.));
#7003=DIRECTION('center_axis',(0.,0.,-1.));
#7004=DIRECTION('ref_axis',(0.938435415243825,-0.345454731355861,0.));
#7005=DIRECTION('',(0.,0.,-1.));
#7006=DIRECTION('center_axis',(0.,0.,-1.));
#7007=DIRECTION('ref_axis',(1.,0.,0.));
#7008=DIRECTION('center_axis',(0.,0.,-1.));
#7009=DIRECTION('ref_axis',(1.,0.,0.));
#7010=DIRECTION('',(0.,0.,-1.));
#7011=DIRECTION('center_axis',(0.,0.,-1.));
#7012=DIRECTION('ref_axis',(1.,0.,0.));
#7013=DIRECTION('center_axis',(0.,0.,-1.));
#7014=DIRECTION('ref_axis',(1.,0.,0.));
#7015=DIRECTION('',(0.,0.,-1.));
#7016=DIRECTION('center_axis',(0.,0.,-1.));
#7017=DIRECTION('ref_axis',(1.,0.,0.));
#7018=DIRECTION('',(0.,0.,-1.));
#7019=DIRECTION('center_axis',(0.,0.,-1.));
#7020=DIRECTION('ref_axis',(1.,0.,0.));
#7021=DIRECTION('',(0.,0.,-1.));
#7022=DIRECTION('center_axis',(0.,0.,-1.));
#7023=DIRECTION('ref_axis',(1.,0.,0.));
#7024=DIRECTION('',(0.,0.,-1.));
#7025=DIRECTION('center_axis',(0.,0.,-1.));
#7026=DIRECTION('ref_axis',(1.,0.,0.));
#7027=DIRECTION('',(0.,0.,-1.));
#7028=DIRECTION('center_axis',(0.,0.,-1.));
#7029=DIRECTION('ref_axis',(1.,0.,0.));
#7030=DIRECTION('',(0.,0.,-1.));
#7031=DIRECTION('center_axis',(0.,0.,-1.));
#7032=DIRECTION('ref_axis',(1.,0.,0.));
#7033=DIRECTION('',(0.,0.,-1.));
#7034=DIRECTION('center_axis',(0.,0.,-1.));
#7035=DIRECTION('ref_axis',(1.,0.,0.));
#7036=DIRECTION('',(0.,0.,-1.));
#7037=DIRECTION('center_axis',(0.,0.,-1.));
#7038=DIRECTION('ref_axis',(1.,0.,0.));
#7039=DIRECTION('',(0.,0.,-1.));
#7040=DIRECTION('center_axis',(0.,0.,-1.));
#7041=DIRECTION('ref_axis',(0.938435444148243,-0.34545465283636,0.));
#7042=DIRECTION('',(0.,0.,-1.));
#7043=DIRECTION('center_axis',(0.,0.,-1.));
#7044=DIRECTION('ref_axis',(1.,0.,0.));
#7045=DIRECTION('center_axis',(0.,0.,-1.));
#7046=DIRECTION('ref_axis',(1.,0.,0.));
#7047=DIRECTION('',(0.,0.,-1.));
#7048=DIRECTION('center_axis',(0.,0.,-1.));
#7049=DIRECTION('ref_axis',(1.,0.,0.));
#7050=DIRECTION('center_axis',(0.,0.,-1.));
#7051=DIRECTION('ref_axis',(1.,0.,0.));
#7052=DIRECTION('',(0.,0.,-1.));
#7053=DIRECTION('center_axis',(0.,0.,-1.));
#7054=DIRECTION('ref_axis',(1.,0.,0.));
#7055=DIRECTION('',(0.,0.,-1.));
#7056=DIRECTION('center_axis',(0.,0.,-1.));
#7057=DIRECTION('ref_axis',(1.,0.,0.));
#7058=DIRECTION('',(0.,0.,-1.));
#7059=DIRECTION('center_axis',(0.,0.,-1.));
#7060=DIRECTION('ref_axis',(1.,0.,0.));
#7061=DIRECTION('',(0.,0.,-1.));
#7062=DIRECTION('center_axis',(0.,0.,-1.));
#7063=DIRECTION('ref_axis',(1.,0.,0.));
#7064=DIRECTION('',(0.,0.,-1.));
#7065=DIRECTION('center_axis',(0.,0.,-1.));
#7066=DIRECTION('ref_axis',(1.,0.,0.));
#7067=DIRECTION('',(0.,0.,-1.));
#7068=DIRECTION('center_axis',(0.,0.,-1.));
#7069=DIRECTION('ref_axis',(1.,0.,0.));
#7070=DIRECTION('',(0.,0.,-1.));
#7071=DIRECTION('center_axis',(0.,0.,-1.));
#7072=DIRECTION('ref_axis',(1.,0.,0.));
#7073=DIRECTION('',(0.,0.,-1.));
#7074=DIRECTION('center_axis',(0.,0.,-1.));
#7075=DIRECTION('ref_axis',(1.,0.,0.));
#7076=DIRECTION('',(0.,0.,-1.));
#7077=DIRECTION('center_axis',(0.,0.,-1.));
#7078=DIRECTION('ref_axis',(0.938435456291759,-0.345454619848221,0.));
#7079=DIRECTION('',(0.,0.,-1.));
#7080=DIRECTION('center_axis',(0.,0.,-1.));
#7081=DIRECTION('ref_axis',(1.,0.,0.));
#7082=DIRECTION('center_axis',(0.,0.,-1.));
#7083=DIRECTION('ref_axis',(1.,0.,0.));
#7084=DIRECTION('center_axis',(0.,0.,-1.));
#7085=DIRECTION('ref_axis',(1.,0.,0.));
#7086=DIRECTION('',(0.,0.,-1.));
#7087=DIRECTION('center_axis',(0.,0.,-1.));
#7088=DIRECTION('ref_axis',(1.,0.,0.));
#7089=DIRECTION('center_axis',(0.,0.,-1.));
#7090=DIRECTION('ref_axis',(1.,0.,0.));
#7091=DIRECTION('',(0.,0.,-1.));
#7092=DIRECTION('center_axis',(0.,0.,-1.));
#7093=DIRECTION('ref_axis',(1.,0.,0.));
#7094=DIRECTION('',(0.,0.,-1.));
#7095=DIRECTION('center_axis',(0.,0.,-1.));
#7096=DIRECTION('ref_axis',(1.,0.,0.));
#7097=DIRECTION('',(0.,0.,-1.));
#7098=DIRECTION('center_axis',(0.,0.,-1.));
#7099=DIRECTION('ref_axis',(1.,0.,0.));
#7100=DIRECTION('',(0.,0.,-1.));
#7101=DIRECTION('center_axis',(0.,0.,-1.));
#7102=DIRECTION('ref_axis',(1.,0.,0.));
#7103=DIRECTION('',(0.,0.,-1.));
#7104=DIRECTION('center_axis',(0.,0.,-1.));
#7105=DIRECTION('ref_axis',(1.,0.,0.));
#7106=DIRECTION('',(0.,0.,-1.));
#7107=DIRECTION('center_axis',(0.,0.,-1.));
#7108=DIRECTION('ref_axis',(1.,0.,0.));
#7109=DIRECTION('',(0.,0.,-1.));
#7110=DIRECTION('center_axis',(0.,0.,-1.));
#7111=DIRECTION('ref_axis',(1.,0.,0.));
#7112=DIRECTION('',(0.,0.,-1.));
#7113=DIRECTION('center_axis',(0.,0.,-1.));
#7114=DIRECTION('ref_axis',(1.,0.,0.));
#7115=DIRECTION('',(0.,0.,-1.));
#7116=DIRECTION('center_axis',(0.,0.,-1.));
#7117=DIRECTION('ref_axis',(0.938435399436813,-0.345454774295956,0.));
#7118=DIRECTION('',(0.,0.,-1.));
#7119=DIRECTION('center_axis',(0.,0.,-1.));
#7120=DIRECTION('ref_axis',(1.,0.,0.));
#7121=DIRECTION('center_axis',(0.,0.,-1.));
#7122=DIRECTION('ref_axis',(1.,0.,0.));
#7123=DIRECTION('center_axis',(0.,0.,-1.));
#7124=DIRECTION('ref_axis',(-0.770520550489697,0.637415156136921,0.));
#7125=DIRECTION('',(1.22464679914735E-16,-5.30860927203279E-30,-1.));
#7126=DIRECTION('center_axis',(0.,0.,1.));
#7127=DIRECTION('ref_axis',(1.,-4.32256196471651E-14,0.));
#7128=DIRECTION('center_axis',(0.,0.,-1.));
#7129=DIRECTION('ref_axis',(1.,-4.32256196471651E-14,0.));
#7130=DIRECTION('',(1.22464679914735E-16,-5.30860927203279E-30,-1.));
#7131=DIRECTION('center_axis',(0.,0.,-1.));
#7132=DIRECTION('ref_axis',(1.,-4.32256196471651E-14,0.));
#7133=DIRECTION('',(1.22464679914735E-16,-5.30860927203279E-30,-1.));
#7134=DIRECTION('center_axis',(0.,0.,-1.));
#7135=DIRECTION('ref_axis',(1.,-4.32256196471651E-14,0.));
#7136=DIRECTION('',(1.22464679914735E-16,-5.30860927203279E-30,-1.));
#7137=DIRECTION('center_axis',(0.,0.,-1.));
#7138=DIRECTION('ref_axis',(1.,-4.32256196471651E-14,0.));
#7139=DIRECTION('',(1.22464679914735E-16,-5.30860927203279E-30,-1.));
#7140=DIRECTION('center_axis',(0.,0.,-1.));
#7141=DIRECTION('ref_axis',(1.,-4.32256196471651E-14,0.));
#7142=DIRECTION('',(1.22464679914735E-16,-5.30860927203279E-30,-1.));
#7143=DIRECTION('center_axis',(0.,0.,-1.));
#7144=DIRECTION('ref_axis',(1.,-4.32256196471651E-14,0.));
#7145=DIRECTION('',(1.22464679914735E-16,-5.30860927203279E-30,-1.));
#7146=DIRECTION('center_axis',(0.,0.,-1.));
#7147=DIRECTION('ref_axis',(1.,-4.32256196471651E-14,0.));
#7148=DIRECTION('',(1.22464679914735E-16,-5.30860927203279E-30,-1.));
#7149=DIRECTION('center_axis',(0.,0.,-1.));
#7150=DIRECTION('ref_axis',(1.,-4.32256196471651E-14,0.));
#7151=DIRECTION('',(1.22464679914735E-16,-5.30860927203279E-30,-1.));
#7152=DIRECTION('center_axis',(0.,0.,-1.));
#7153=DIRECTION('ref_axis',(1.,-4.32256196471651E-14,0.));
#7154=DIRECTION('',(1.22464679914735E-16,-5.30860927203279E-30,-1.));
#7155=DIRECTION('center_axis',(0.,0.,-1.));
#7156=DIRECTION('ref_axis',(1.,-4.32256196471651E-14,0.));
#7157=DIRECTION('',(1.22464679914735E-16,-5.30860927203279E-30,-1.));
#7158=DIRECTION('center_axis',(0.,0.,-1.));
#7159=DIRECTION('ref_axis',(-0.60934875646219,-0.792902322482399,0.));
#7160=DIRECTION('',(1.22464679914735E-16,-5.30860927203279E-30,-1.));
#7161=DIRECTION('center_axis',(0.,0.,-1.));
#7162=DIRECTION('ref_axis',(1.,-4.32256196471651E-14,0.));
#7163=DIRECTION('center_axis',(0.,0.,-1.));
#7164=DIRECTION('ref_axis',(-0.770520310070594,0.637415446760365,0.));
#7165=DIRECTION('',(1.22464679914735E-16,-5.17626898017763E-30,-1.));
#7166=DIRECTION('center_axis',(0.,0.,1.));
#7167=DIRECTION('ref_axis',(1.,-4.2144979155986E-14,0.));
#7168=DIRECTION('center_axis',(0.,0.,-1.));
#7169=DIRECTION('ref_axis',(1.,-4.2144979155986E-14,0.));
#7170=DIRECTION('',(1.22464679914735E-16,-5.17626898017763E-30,-1.));
#7171=DIRECTION('center_axis',(0.,0.,-1.));
#7172=DIRECTION('ref_axis',(1.,-4.2144979155986E-14,0.));
#7173=DIRECTION('',(1.22464679914735E-16,-5.17626898017763E-30,-1.));
#7174=DIRECTION('center_axis',(0.,0.,-1.));
#7175=DIRECTION('ref_axis',(1.,-4.2144979155986E-14,0.));
#7176=DIRECTION('',(1.22464679914735E-16,-5.17626898017763E-30,-1.));
#7177=DIRECTION('center_axis',(0.,0.,-1.));
#7178=DIRECTION('ref_axis',(1.,-4.2144979155986E-14,0.));
#7179=DIRECTION('',(1.22464679914735E-16,-5.17626898017763E-30,-1.));
#7180=DIRECTION('center_axis',(0.,0.,-1.));
#7181=DIRECTION('ref_axis',(1.,-4.2144979155986E-14,0.));
#7182=DIRECTION('',(1.22464679914735E-16,-5.17626898017763E-30,-1.));
#7183=DIRECTION('center_axis',(0.,0.,-1.));
#7184=DIRECTION('ref_axis',(1.,-4.2144979155986E-14,0.));
#7185=DIRECTION('',(1.22464679914735E-16,-5.17626898017763E-30,-1.));
#7186=DIRECTION('center_axis',(0.,0.,-1.));
#7187=DIRECTION('ref_axis',(1.,-4.2144979155986E-14,0.));
#7188=DIRECTION('',(1.22464679914735E-16,-5.17626898017763E-30,-1.));
#7189=DIRECTION('center_axis',(0.,0.,-1.));
#7190=DIRECTION('ref_axis',(1.,-4.2144979155986E-14,0.));
#7191=DIRECTION('',(1.22464679914735E-16,-5.17626898017763E-30,-1.));
#7192=DIRECTION('center_axis',(0.,0.,-1.));
#7193=DIRECTION('ref_axis',(1.,-4.2144979155986E-14,0.));
#7194=DIRECTION('',(1.22464679914735E-16,-5.17626898017763E-30,-1.));
#7195=DIRECTION('center_axis',(0.,0.,-1.));
#7196=DIRECTION('ref_axis',(1.,-4.2144979155986E-14,0.));
#7197=DIRECTION('',(1.22464679914735E-16,-5.17626898017763E-30,-1.));
#7198=DIRECTION('center_axis',(0.,0.,-1.));
#7199=DIRECTION('ref_axis',(-0.609348813471299,-0.792902278670657,0.));
#7200=DIRECTION('',(1.22464679914735E-16,-5.17626898017763E-30,-1.));
#7201=DIRECTION('center_axis',(0.,0.,-1.));
#7202=DIRECTION('ref_axis',(1.,-4.2144979155986E-14,0.));
#7203=DIRECTION('center_axis',(0.,0.,-1.));
#7204=DIRECTION('ref_axis',(-0.770520589723051,0.637415108710832,0.));
#7205=DIRECTION('',(1.22464679914735E-16,-5.37477941796036E-30,-1.));
#7206=DIRECTION('center_axis',(0.,0.,1.));
#7207=DIRECTION('ref_axis',(1.,-4.37659398927547E-14,0.));
#7208=DIRECTION('center_axis',(0.,0.,-1.));
#7209=DIRECTION('ref_axis',(1.,-4.37659398927547E-14,0.));
#7210=DIRECTION('',(1.22464679914735E-16,-5.37477941796036E-30,-1.));
#7211=DIRECTION('center_axis',(0.,0.,-1.));
#7212=DIRECTION('ref_axis',(1.,-4.37659398927547E-14,0.));
#7213=DIRECTION('',(1.22464679914735E-16,-5.37477941796036E-30,-1.));
#7214=DIRECTION('center_axis',(0.,0.,-1.));
#7215=DIRECTION('ref_axis',(1.,-4.37659398927547E-14,0.));
#7216=DIRECTION('',(1.22464679914735E-16,-5.37477941796036E-30,-1.));
#7217=DIRECTION('center_axis',(0.,0.,-1.));
#7218=DIRECTION('ref_axis',(1.,-4.37659398927547E-14,0.));
#7219=DIRECTION('',(1.22464679914735E-16,-5.37477941796036E-30,-1.));
#7220=DIRECTION('center_axis',(0.,0.,-1.));
#7221=DIRECTION('ref_axis',(1.,-4.37659398927547E-14,0.));
#7222=DIRECTION('',(1.22464679914735E-16,-5.37477941796036E-30,-1.));
#7223=DIRECTION('center_axis',(0.,0.,-1.));
#7224=DIRECTION('ref_axis',(1.,-4.37659398927547E-14,0.));
#7225=DIRECTION('',(1.22464679914735E-16,-5.37477941796036E-30,-1.));
#7226=DIRECTION('center_axis',(0.,0.,-1.));
#7227=DIRECTION('ref_axis',(1.,-4.37659398927547E-14,0.));
#7228=DIRECTION('',(1.22464679914735E-16,-5.37477941796036E-30,-1.));
#7229=DIRECTION('center_axis',(0.,0.,-1.));
#7230=DIRECTION('ref_axis',(1.,-4.37659398927547E-14,0.));
#7231=DIRECTION('',(1.22464679914735E-16,-5.37477941796036E-30,-1.));
#7232=DIRECTION('center_axis',(0.,0.,-1.));
#7233=DIRECTION('ref_axis',(1.,-4.37659398927547E-14,0.));
#7234=DIRECTION('',(1.22464679914735E-16,-5.37477941796036E-30,-1.));
#7235=DIRECTION('center_axis',(0.,0.,-1.));
#7236=DIRECTION('ref_axis',(1.,-4.37659398927547E-14,0.));
#7237=DIRECTION('',(1.22464679914735E-16,-5.37477941796036E-30,-1.));
#7238=DIRECTION('center_axis',(0.,0.,-1.));
#7239=DIRECTION('ref_axis',(-0.609348731823397,-0.792902341417414,0.));
#7240=DIRECTION('',(1.22464679914735E-16,-5.37477941796036E-30,-1.));
#7241=DIRECTION('center_axis',(0.,0.,-1.));
#7242=DIRECTION('ref_axis',(1.,-4.37659398927547E-14,0.));
#7243=DIRECTION('center_axis',(0.,0.,-1.));
#7244=DIRECTION('ref_axis',(-0.770520370143733,0.637415374142769,0.));
#7245=DIRECTION('',(1.22464679914735E-16,-5.30860927203279E-30,-1.));
#7246=DIRECTION('center_axis',(0.,0.,1.));
#7247=DIRECTION('ref_axis',(1.,-4.32256196471651E-14,0.));
#7248=DIRECTION('center_axis',(0.,0.,-1.));
#7249=DIRECTION('ref_axis',(1.,-4.32256196471651E-14,0.));
#7250=DIRECTION('',(1.22464679914735E-16,-5.30860927203279E-30,-1.));
#7251=DIRECTION('center_axis',(0.,0.,-1.));
#7252=DIRECTION('ref_axis',(1.,-4.32256196471651E-14,0.));
#7253=DIRECTION('',(1.22464679914735E-16,-5.30860927203279E-30,-1.));
#7254=DIRECTION('center_axis',(0.,0.,-1.));
#7255=DIRECTION('ref_axis',(1.,-4.32256196471651E-14,0.));
#7256=DIRECTION('',(1.22464679914735E-16,-5.30860927203279E-30,-1.));
#7257=DIRECTION('center_axis',(0.,0.,-1.));
#7258=DIRECTION('ref_axis',(1.,-4.32256196471651E-14,0.));
#7259=DIRECTION('',(1.22464679914735E-16,-5.30860927203279E-30,-1.));
#7260=DIRECTION('center_axis',(0.,0.,-1.));
#7261=DIRECTION('ref_axis',(1.,-4.32256196471651E-14,0.));
#7262=DIRECTION('',(1.22464679914735E-16,-5.30860927203279E-30,-1.));
#7263=DIRECTION('center_axis',(0.,0.,-1.));
#7264=DIRECTION('ref_axis',(1.,-4.32256196471651E-14,0.));
#7265=DIRECTION('',(1.22464679914735E-16,-5.30860927203279E-30,-1.));
#7266=DIRECTION('center_axis',(0.,0.,-1.));
#7267=DIRECTION('ref_axis',(1.,-4.32256196471651E-14,0.));
#7268=DIRECTION('',(1.22464679914735E-16,-5.30860927203279E-30,-1.));
#7269=DIRECTION('center_axis',(0.,0.,-1.));
#7270=DIRECTION('ref_axis',(1.,-4.32256196471651E-14,0.));
#7271=DIRECTION('',(1.22464679914735E-16,-5.30860927203279E-30,-1.));
#7272=DIRECTION('center_axis',(0.,0.,-1.));
#7273=DIRECTION('ref_axis',(1.,-4.32256196471651E-14,0.));
#7274=DIRECTION('',(1.22464679914735E-16,-5.30860927203279E-30,-1.));
#7275=DIRECTION('center_axis',(0.,0.,-1.));
#7276=DIRECTION('ref_axis',(1.,-4.32256196471651E-14,0.));
#7277=DIRECTION('',(1.22464679914735E-16,-5.30860927203279E-30,-1.));
#7278=DIRECTION('center_axis',(0.,0.,-1.));
#7279=DIRECTION('ref_axis',(-0.6093487836746,-0.792902301569547,0.));
#7280=DIRECTION('',(1.22464679914735E-16,-5.30860927203279E-30,-1.));
#7281=DIRECTION('center_axis',(0.,0.,-1.));
#7282=DIRECTION('ref_axis',(1.,-4.32256196471651E-14,0.));
#7283=DIRECTION('center_axis',(0.707106781186548,-0.707106781186547,0.));
#7284=DIRECTION('ref_axis',(-0.5,-0.499999999999999,0.707106781186548));
#7285=DIRECTION('',(-0.707106781186548,0.707106781186547,0.));
#7286=DIRECTION('center_axis',(0.923879532511287,-0.38268343236509,0.));
#7287=DIRECTION('ref_axis',(0.38268343236509,0.923879532511287,0.));
#7288=DIRECTION('',(0.707106781186548,-0.707106781186547,0.));
#7289=DIRECTION('center_axis',(0.38268343236509,-0.923879532511287,-9.37720122241284E-16));
#7290=DIRECTION('ref_axis',(0.923879532511287,0.38268343236509,-2.26385663682506E-15));
#7291=DIRECTION('center_axis',(1.,0.,0.));
#7292=DIRECTION('ref_axis',(0.,-0.707106781186547,0.707106781186548));
#7293=DIRECTION('',(-1.,0.,0.));
#7294=DIRECTION('center_axis',(0.923879532511287,0.38268343236509,0.));
#7295=DIRECTION('ref_axis',(-0.38268343236509,0.923879532511287,0.));
#7296=DIRECTION('',(1.,0.,0.));
#7297=DIRECTION('center_axis',(0.707106781186548,0.707106781186547,0.));
#7298=DIRECTION('ref_axis',(0.499999999999999,-0.5,0.707106781186548));
#7299=DIRECTION('',(-0.707106781186548,-0.707106781186547,0.));
#7300=DIRECTION('center_axis',(0.38268343236509,0.923879532511287,0.));
#7301=DIRECTION('ref_axis',(-0.923879532511287,0.38268343236509,0.));
#7302=DIRECTION('',(0.707106781186548,0.707106781186547,0.));
#7303=DIRECTION('center_axis',(0.,1.,0.));
#7304=DIRECTION('ref_axis',(0.707106781186547,0.,0.707106781186548));
#7305=DIRECTION('',(0.,-1.,0.));
#7306=DIRECTION('center_axis',(-0.707106781186548,0.707106781186548,0.));
#7307=DIRECTION('ref_axis',(-0.707106781186547,-0.707106781186547,0.));
#7308=DIRECTION('',(0.,1.,0.));
#7309=DIRECTION('center_axis',(-1.,0.,0.));
#7310=DIRECTION('ref_axis',(0.,0.707106781186547,0.707106781186548));
#7311=DIRECTION('',(-1.,0.,0.));
#7312=DIRECTION('',(1.,0.,0.));
#7313=DIRECTION('center_axis',(-0.707106781186548,-0.707106781186548,0.));
#7314=DIRECTION('ref_axis',(0.707106781186547,-0.707106781186547,0.));
#7315=DIRECTION('center_axis',(0.,-1.,0.));
#7316=DIRECTION('ref_axis',(-0.707106781186547,0.,0.707106781186548));
#7317=DIRECTION('',(0.,-1.,0.));
#7318=DIRECTION('',(0.,1.,0.));
#7319=DIRECTION('center_axis',(0.,1.,0.));
#7320=DIRECTION('ref_axis',(-1.,0.,0.));
#7321=DIRECTION('',(0.,0.,1.));
#7322=DIRECTION('',(1.,0.,0.));
#7323=DIRECTION('',(1.,0.,0.));
#7324=DIRECTION('',(1.,0.,0.));
#7325=DIRECTION('',(0.,0.,1.));
#7326=DIRECTION('center_axis',(-1.,0.,0.));
#7327=DIRECTION('ref_axis',(0.,-1.,0.));
#7328=DIRECTION('',(0.,0.,1.));
#7329=DIRECTION('',(0.,1.,0.));
#7330=DIRECTION('',(0.,1.,0.));
#7331=DIRECTION('center_axis',(-0.707106781186547,-0.707106781186548,0.));
#7332=DIRECTION('ref_axis',(0.707106781186548,-0.707106781186547,0.));
#7333=DIRECTION('',(0.,0.,1.));
#7334=DIRECTION('',(-0.707106781186548,0.707106781186547,0.));
#7335=DIRECTION('center_axis',(0.,0.,1.));
#7336=DIRECTION('ref_axis',(1.,0.,0.));
#7337=DIRECTION('',(0.,-1.,0.));
#7338=DIRECTION('center_axis',(0.,0.,1.));
#7339=DIRECTION('ref_axis',(-1.,-1.22464679914735E-16,0.));
#7340=DIRECTION('',(0.,-1.,0.));
#7341=DIRECTION('',(1.,0.,0.));
#7342=DIRECTION('',(0.,1.,0.));
#7343=DIRECTION('center_axis',(0.,0.,1.));
#7344=DIRECTION('ref_axis',(-1.,-1.22464679914735E-16,0.));
#7345=DIRECTION('center_axis',(0.,0.,1.));
#7346=DIRECTION('ref_axis',(-1.,-1.22464679914735E-16,0.));
#7347=DIRECTION('',(0.,1.,0.));
#7348=DIRECTION('',(-1.,0.,0.));
#7349=DIRECTION('center_axis',(0.,1.,0.));
#7350=DIRECTION('ref_axis',(0.707106781186546,0.,0.707106781186549));
#7351=DIRECTION('center_axis',(0.707106781186547,0.707106781186548,1.57009245868377E-15));
#7352=DIRECTION('ref_axis',(0.707106781186548,-0.707106781186547,1.57009245868377E-15));
#7353=DIRECTION('',(0.,1.,0.));
#7354=DIRECTION('center_axis',(-0.707106781186547,0.707106781186548,7.85046229341886E-16));
#7355=DIRECTION('ref_axis',(0.707106781186548,0.707106781186547,7.85046229341885E-16));
#7356=DIRECTION('center_axis',(1.,0.,0.));
#7357=DIRECTION('ref_axis',(0.,-0.707106781186545,0.70710678118655));
#7358=DIRECTION('center_axis',(0.707106781186547,-0.707106781186548,7.85046229341886E-16));
#7359=DIRECTION('ref_axis',(-0.707106781186548,-0.707106781186547,7.85046229341885E-16));
#7360=DIRECTION('',(1.,0.,0.));
#7361=DIRECTION('center_axis',(0.,-1.,0.));
#7362=DIRECTION('ref_axis',(-0.707106781186546,0.,0.707106781186549));
#7363=DIRECTION('center_axis',(-0.707106781186547,-0.707106781186548,1.57009245868377E-15));
#7364=DIRECTION('ref_axis',(-0.707106781186548,0.707106781186547,1.57009245868377E-15));
#7365=DIRECTION('',(0.,-1.,0.));
#7366=DIRECTION('center_axis',(-1.,0.,0.));
#7367=DIRECTION('ref_axis',(0.,0.707106781186545,0.70710678118655));
#7368=DIRECTION('',(-1.,0.,0.));
#7369=DIRECTION('center_axis',(0.,1.,0.));
#7370=DIRECTION('ref_axis',(-1.,0.,0.));
#7371=DIRECTION('',(0.,0.,1.));
#7372=DIRECTION('',(-1.,0.,0.));
#7373=DIRECTION('',(0.,0.,1.));
#7374=DIRECTION('center_axis',(1.,0.,0.));
#7375=DIRECTION('ref_axis',(0.,1.,0.));
#7376=DIRECTION('',(0.,0.,1.));
#7377=DIRECTION('',(0.,1.,0.));
#7378=DIRECTION('center_axis',(0.,0.,-1.));
#7379=DIRECTION('ref_axis',(-1.,0.,0.));
#7380=DIRECTION('center_axis',(-1.22464679914735E-16,-1.,0.));
#7381=DIRECTION('ref_axis',(1.,-1.22464679914735E-16,0.));
#7382=DIRECTION('center_axis',(0.,0.,-1.));
#7383=DIRECTION('ref_axis',(-1.,-1.22464679914735E-16,0.));
#7384=DIRECTION('center_axis',(0.,0.,-1.));
#7385=DIRECTION('ref_axis',(-1.,-1.22464679914735E-16,0.));
#7386=DIRECTION('center_axis',(0.,0.,-1.));
#7387=DIRECTION('ref_axis',(-1.,0.,0.));
#7388=DIRECTION('center_axis',(-1.22464679914735E-16,-1.,0.));
#7389=DIRECTION('ref_axis',(1.,-1.22464679914735E-16,0.));
#7390=DIRECTION('center_axis',(0.,0.,-1.));
#7391=DIRECTION('ref_axis',(-1.,-1.22464679914735E-16,0.));
#7392=DIRECTION('center_axis',(0.,0.,-1.));
#7393=DIRECTION('ref_axis',(-1.,-1.22464679914735E-16,0.));
#7394=DIRECTION('center_axis',(0.,0.,-1.));
#7395=DIRECTION('ref_axis',(1.,0.,0.));
#7396=DIRECTION('',(0.,0.,-1.));
#7397=DIRECTION('center_axis',(0.,0.,1.));
#7398=DIRECTION('ref_axis',(1.,0.,0.));
#7399=DIRECTION('center_axis',(0.,0.,-1.));
#7400=DIRECTION('ref_axis',(1.,0.,0.));
#7401=DIRECTION('',(0.,0.,-1.));
#7402=DIRECTION('center_axis',(0.,0.,1.));
#7403=DIRECTION('ref_axis',(1.,0.,0.));
#7404=DIRECTION('center_axis',(0.,0.,-1.));
#7405=DIRECTION('ref_axis',(1.,-4.32256196471651E-14,0.));
#7406=DIRECTION('center_axis',(0.,0.,1.));
#7407=DIRECTION('ref_axis',(1.,0.,0.));
#7408=DIRECTION('',(0.,-1.,0.));
#7409=DIRECTION('',(-0.707106781186547,-0.707106781186547,0.));
#7410=DIRECTION('',(-1.,0.,0.));
#7411=DIRECTION('',(-0.707106781186547,0.707106781186547,0.));
#7412=DIRECTION('',(0.,1.,0.));
#7413=DIRECTION('',(1.,0.,0.));
#7414=DIRECTION('',(1.,0.,0.));
#7415=DIRECTION('',(0.,1.,0.));
#7416=DIRECTION('',(-1.,0.,0.));
#7417=DIRECTION('',(0.,-1.,0.));
#7418=DIRECTION('',(1.,0.,0.));
#7419=DIRECTION('',(0.,1.,0.));
#7420=DIRECTION('',(-1.,0.,0.));
#7421=DIRECTION('',(0.,-1.,0.));
#7422=DIRECTION('',(1.,0.,0.));
#7423=DIRECTION('',(0.,1.,0.));
#7424=DIRECTION('',(-1.,0.,0.));
#7425=DIRECTION('',(0.,-1.,0.));
#7426=DIRECTION('center_axis',(0.,0.,-1.));
#7427=DIRECTION('ref_axis',(1.,-4.37659398927547E-14,0.));
#7428=DIRECTION('center_axis',(0.,0.,-1.));
#7429=DIRECTION('ref_axis',(1.,-4.2144979155986E-14,0.));
#7430=DIRECTION('center_axis',(0.,0.,-1.));
#7431=DIRECTION('ref_axis',(1.,-4.32256196471651E-14,0.));
#7432=DIRECTION('center_axis',(0.,0.,1.));
#7433=DIRECTION('ref_axis',(1.,0.,0.));
#7434=DIRECTION('',(-1.,0.,0.));
#7435=DIRECTION('',(-0.707106781186548,-0.707106781186547,0.));
#7436=DIRECTION('',(0.,-1.,0.));
#7437=DIRECTION('',(-1.,0.,0.));
#7438=DIRECTION('',(0.,1.,0.));
#7439=DIRECTION('',(1.,0.,0.));
#7440=DIRECTION('',(0.,-1.,0.));
#7441=DIRECTION('',(-1.,0.,0.));
#7442=DIRECTION('',(0.,1.,0.));
#7443=DIRECTION('',(1.,0.,0.));
#7444=DIRECTION('',(0.,-1.,0.));
#7445=DIRECTION('',(-1.,0.,0.));
#7446=DIRECTION('',(0.,1.,0.));
#7447=DIRECTION('',(1.,0.,0.));
#7448=DIRECTION('',(0.,-1.,0.));
#7449=DIRECTION('center_axis',(0.,0.,1.));
#7450=DIRECTION('ref_axis',(-1.,0.,0.));
#7451=DIRECTION('center_axis',(0.,0.,-1.));
#7452=DIRECTION('ref_axis',(1.,0.,0.));
#7453=DIRECTION('center_axis',(0.,0.,1.));
#7454=DIRECTION('ref_axis',(-1.,0.,0.));
#7455=DIRECTION('',(0.,-1.,0.));
#7456=DIRECTION('center_axis',(0.,0.,-1.));
#7457=DIRECTION('ref_axis',(1.,0.,0.));
#7458=DIRECTION('center_axis',(0.,0.,-1.));
#7459=DIRECTION('ref_axis',(1.,0.,0.));
#7460=DIRECTION('center_axis',(0.,0.,1.));
#7461=DIRECTION('ref_axis',(-1.,0.,0.));
#7462=DIRECTION('center_axis',(0.,0.,-1.));
#7463=DIRECTION('ref_axis',(1.,0.,0.));
#7464=DIRECTION('center_axis',(0.,0.,1.));
#7465=DIRECTION('ref_axis',(-1.,0.,0.));
#7466=DIRECTION('center_axis',(0.,-1.,0.));
#7467=DIRECTION('ref_axis',(-1.,0.,0.));
#7468=DIRECTION('',(0.,0.,-1.));
#7469=DIRECTION('',(0.,0.,-1.));
#7470=DIRECTION('center_axis',(1.,0.,0.));
#7471=DIRECTION('ref_axis',(0.,-1.,0.));
#7472=DIRECTION('',(0.,0.,-1.));
#7473=DIRECTION('center_axis',(0.,1.,0.));
#7474=DIRECTION('ref_axis',(1.,0.,0.));
#7475=DIRECTION('',(0.,0.,-1.));
#7476=DIRECTION('center_axis',(-1.,0.,0.));
#7477=DIRECTION('ref_axis',(0.,1.,0.));
#7478=DIRECTION('center_axis',(0.,-1.,0.));
#7479=DIRECTION('ref_axis',(-1.,0.,0.));
#7480=DIRECTION('',(0.,0.,-1.));
#7481=DIRECTION('',(0.,0.,-1.));
#7482=DIRECTION('center_axis',(1.,0.,0.));
#7483=DIRECTION('ref_axis',(0.,-1.,0.));
#7484=DIRECTION('',(0.,0.,-1.));
#7485=DIRECTION('center_axis',(0.,1.,0.));
#7486=DIRECTION('ref_axis',(1.,0.,0.));
#7487=DIRECTION('',(0.,0.,-1.));
#7488=DIRECTION('center_axis',(-1.,0.,0.));
#7489=DIRECTION('ref_axis',(0.,1.,0.));
#7490=DIRECTION('center_axis',(0.,-1.,0.));
#7491=DIRECTION('ref_axis',(-1.,0.,0.));
#7492=DIRECTION('',(0.,0.,-1.));
#7493=DIRECTION('',(0.,0.,-1.));
#7494=DIRECTION('center_axis',(1.,0.,0.));
#7495=DIRECTION('ref_axis',(0.,-1.,0.));
#7496=DIRECTION('',(0.,0.,-1.));
#7497=DIRECTION('center_axis',(0.,1.,0.));
#7498=DIRECTION('ref_axis',(1.,0.,0.));
#7499=DIRECTION('',(0.,0.,-1.));
#7500=DIRECTION('center_axis',(-1.,0.,0.));
#7501=DIRECTION('ref_axis',(0.,1.,0.));
#7502=DIRECTION('center_axis',(0.,0.,1.));
#7503=DIRECTION('ref_axis',(1.,0.,0.));
#7504=DIRECTION('',(0.,-1.,0.));
#7505=DIRECTION('',(1.,0.,0.));
#7506=DIRECTION('',(0.707106781186548,0.707106781186548,0.));
#7507=DIRECTION('',(0.,1.,0.));
#7508=DIRECTION('',(-1.,0.,0.));
#7509=DIRECTION('',(0.,-1.,0.));
#7510=DIRECTION('',(0.707106781186548,-0.707106781186548,0.));
#7511=DIRECTION('',(1.,0.,0.));
#7512=DIRECTION('center_axis',(0.,-1.,0.));
#7513=DIRECTION('ref_axis',(1.,0.,0.));
#7514=DIRECTION('',(0.,0.,1.));
#7515=DIRECTION('center_axis',(-1.,0.,0.));
#7516=DIRECTION('ref_axis',(0.,-1.,0.));
#7517=DIRECTION('center_axis',(0.,-1.,0.));
#7518=DIRECTION('ref_axis',(1.,0.,0.));
#7519=DIRECTION('',(0.,0.,1.));
#7520=DIRECTION('center_axis',(0.707106781186547,-0.707106781186548,0.));
#7521=DIRECTION('ref_axis',(0.707106781186548,0.707106781186547,0.));
#7522=DIRECTION('',(0.,0.,1.));
#7523=DIRECTION('center_axis',(1.,0.,0.));
#7524=DIRECTION('ref_axis',(0.,1.,0.));
#7525=DIRECTION('',(0.,0.,1.));
#7526=DIRECTION('',(0.,0.,1.));
#7527=DIRECTION('center_axis',(0.,-1.,0.));
#7528=DIRECTION('ref_axis',(1.,0.,0.));
#7529=DIRECTION('',(0.,0.,1.));
#7530=DIRECTION('center_axis',(-1.,0.,0.));
#7531=DIRECTION('ref_axis',(0.,-1.,0.));
#7532=DIRECTION('',(0.,0.,1.));
#7533=DIRECTION('center_axis',(1.,0.,0.));
#7534=DIRECTION('ref_axis',(0.,1.,0.));
#7535=DIRECTION('center_axis',(-0.707106781186548,0.707106781186548,0.));
#7536=DIRECTION('ref_axis',(-0.707106781186548,-0.707106781186548,0.));
#7537=DIRECTION('',(0.,0.,1.));
#7538=DIRECTION('center_axis',(0.,1.,0.));
#7539=DIRECTION('ref_axis',(-1.,0.,0.));
#7540=DIRECTION('',(0.,0.,1.));
#7541=DIRECTION('center_axis',(0.707106781186548,0.707106781186548,0.));
#7542=DIRECTION('ref_axis',(-0.707106781186548,0.707106781186548,0.));
#8354=CARTESIAN_POINT('',(0.,0.,0.));
#8355=CARTESIAN_POINT('Origin',(15.,10.,4.));
#8356=CARTESIAN_POINT('',(13.3328088490546,10.0013492358765,0.571480363390205));
#8357=CARTESIAN_POINT('',(13.3364070293386,10.0006645492999,0.378519636609792));
#8358=CARTESIAN_POINT('',(13.334,10.,4.));
#8359=CARTESIAN_POINT('',(16.6117095221421,9.57816067485776,0.));
#8360=CARTESIAN_POINT('Ctrl Pts',(13.3364070293386,10.0006645492999,0.378519636609792));
#8361=CARTESIAN_POINT('Ctrl Pts',(13.3354289147321,10.2261439494212,0.363487571935548));
#8362=CARTESIAN_POINT('Ctrl Pts',(13.3780964617564,10.4512892386983,0.348455507261304));
#8363=CARTESIAN_POINT('Ctrl Pts',(13.4661891862405,10.6570298059976,0.33342344258706));
#8364=CARTESIAN_POINT('Ctrl Pts',(13.6832967870101,11.1640846304335,0.29637639341072));
#8365=CARTESIAN_POINT('Ctrl Pts',(14.1763138565653,11.5532764803646,0.259329344234379));
#8366=CARTESIAN_POINT('Ctrl Pts',(14.7201523395477,11.6454139726504,0.222282295058039));
#8367=CARTESIAN_POINT('Ctrl Pts',(15.2639908225302,11.7375514649362,0.185235245881699));
#8368=CARTESIAN_POINT('Ctrl Pts',(15.8586507189399,11.5326345995767,0.14818819670536));
#8369=CARTESIAN_POINT('Ctrl Pts',(16.230649324425,11.1267737685767,0.11114114752902));
#8370=CARTESIAN_POINT('Ctrl Pts',(16.6026479299101,10.7209129375768,0.074094098352681));
#8371=CARTESIAN_POINT('Ctrl Pts',(16.7519852444706,10.1141081409362,0.0370470491763412));
#8372=CARTESIAN_POINT('Ctrl Pts',(16.6117095221421,9.5781606748578,2.42861286636753E-15));
#8373=CARTESIAN_POINT('',(14.324922814325,8.47690223774665,0.));
#8374=CARTESIAN_POINT('Origin',(15.,10.,0.));
#8375=CARTESIAN_POINT('Ctrl Pts',(14.3235905172155,8.47417638326182,1.73472347597681E-17));
#8376=CARTESIAN_POINT('Ctrl Pts',(14.8183179067709,8.25559293309757,0.0363261751465299));
#8377=CARTESIAN_POINT('Ctrl Pts',(15.4299365639682,8.29934549446852,0.0726523502930599));
#8378=CARTESIAN_POINT('Ctrl Pts',(15.8878245545432,8.58718953131908,0.10897852543959));
#8379=CARTESIAN_POINT('Ctrl Pts',(16.354799093857,8.88074568319316,0.14602557461593));
#8380=CARTESIAN_POINT('Ctrl Pts',(16.6618810168406,9.42817717104187,0.18307262379227));
#8381=CARTESIAN_POINT('Ctrl Pts',(16.6686053025862,9.97953156441245,0.22011967296861));
#8382=CARTESIAN_POINT('Ctrl Pts',(16.6753295883318,10.530885957783,0.257166722144951));
#8383=CARTESIAN_POINT('Ctrl Pts',(16.3816962368394,11.0861632566755,0.294213771321291));
#8384=CARTESIAN_POINT('Ctrl Pts',(15.9220537145076,11.3909183482768,0.331260820497631));
#8385=CARTESIAN_POINT('Ctrl Pts',(15.4624111921758,11.6956734398782,0.368307869673971));
#8386=CARTESIAN_POINT('Ctrl Pts',(14.8367594990047,11.7499063241884,0.405354918850311));
#8387=CARTESIAN_POINT('Ctrl Pts',(14.3314685943663,11.5289531757505,0.442401968026651));
#8388=CARTESIAN_POINT('Ctrl Pts',(13.8261776897279,11.3080000273125,0.479449017202991));
#8389=CARTESIAN_POINT('Ctrl Pts',(13.4412475736223,10.8118608461263,0.516496066379331));
#8390=CARTESIAN_POINT('Ctrl Pts',(13.3528420328787,10.2675275034982,0.55354311555567));
#8391=CARTESIAN_POINT('Ctrl Pts',(13.338574121043,10.1796766733746,0.559522198167182));
#8392=CARTESIAN_POINT('Ctrl Pts',(13.3320298587031,10.0905705179199,0.565501280778694));
#8393=CARTESIAN_POINT('Ctrl Pts',(13.3328088490546,10.0013492358765,0.571480363390205));
#8394=CARTESIAN_POINT('Origin',(15.,10.,4.));
#8395=CARTESIAN_POINT('',(13.3366506987084,10.0003647761852,1.27148036339021));
#8396=CARTESIAN_POINT('',(13.3350093517191,9.9985620319516,1.07851963660979));
#8397=CARTESIAN_POINT('',(13.334,10.,4.));
#8398=CARTESIAN_POINT('Ctrl Pts',(13.3350093517191,9.9985620319516,1.07851963660979));
#8399=CARTESIAN_POINT('Ctrl Pts',(13.3382277662221,10.3890985886774,1.05243653366026));
#8400=CARTESIAN_POINT('Ctrl Pts',(13.4753923609414,10.7816700702397,1.02635343071072));
#8401=CARTESIAN_POINT('Ctrl Pts',(13.7262226055549,11.0780443718138,1.00027032776118));
#8402=CARTESIAN_POINT('Ctrl Pts',(14.0824885155229,11.498998632749,0.963223278584839));
#8403=CARTESIAN_POINT('Ctrl Pts',(14.6680617736869,11.7258861702055,0.9261762294085));
#8404=CARTESIAN_POINT('Ctrl Pts',(15.214946994521,11.6548455259047,0.88912918023216));
#8405=CARTESIAN_POINT('Ctrl Pts',(15.761832215355,11.5838048816039,0.85208213105582));
#8406=CARTESIAN_POINT('Ctrl Pts',(16.2700293988592,11.2148360555457,0.81503508187948));
#8407=CARTESIAN_POINT('Ctrl Pts',(16.5069275188232,10.7168466062646,0.77798803270314));
#8408=CARTESIAN_POINT('Ctrl Pts',(16.7438256387873,10.2188571569834,0.7409409835268));
#8409=CARTESIAN_POINT('Ctrl Pts',(16.7094246952114,9.59184708447927,0.703893934350459));
#8410=CARTESIAN_POINT('Ctrl Pts',(16.4195065689417,9.12271321406216,0.666846885174119));
#8411=CARTESIAN_POINT('Ctrl Pts',(16.1295884426719,8.65357934364505,0.62979983599778));
#8412=CARTESIAN_POINT('Ctrl Pts',(15.5841531337084,8.34232167531498,0.59275278682144));
#8413=CARTESIAN_POINT('Ctrl Pts',(15.032763395353,8.33153873726589,0.5557057376451));
#8414=CARTESIAN_POINT('Ctrl Pts',(14.4813736569975,8.32075579921679,0.518658688468759));
#8415=CARTESIAN_POINT('Ctrl Pts',(13.9240294892501,8.61044759144868,0.481611639292419));
#8416=CARTESIAN_POINT('Ctrl Pts',(13.6159564713684,9.06775238703494,0.444564590116079));
#8417=CARTESIAN_POINT('Ctrl Pts',(13.4328859471306,9.33950299096684,0.422549605613983));
#8418=CARTESIAN_POINT('Ctrl Pts',(13.337839512392,9.67044208107719,0.400534621111888));
#8419=CARTESIAN_POINT('Ctrl Pts',(13.3364070293386,10.0006645492999,0.378519636609792));
#8420=CARTESIAN_POINT('Ctrl Pts',(13.3328088490546,10.0013492358765,0.571480363390205));
#8421=CARTESIAN_POINT('Ctrl Pts',(13.3368565680386,9.5377457054525,0.602548329955034));
#8422=CARTESIAN_POINT('Ctrl Pts',(13.5386288253055,9.07103380876728,0.633616296519862));
#8423=CARTESIAN_POINT('Ctrl Pts',(13.8819529042008,8.76117501449623,0.664684263084691));
#8424=CARTESIAN_POINT('Ctrl Pts',(14.2913502816478,8.39168337219233,0.70173131226103));
#8425=CARTESIAN_POINT('Ctrl Pts',(14.9020260019234,8.24522759165455,0.73877836143737));
#8426=CARTESIAN_POINT('Ctrl Pts',(15.4344829009358,8.38881597583482,0.77582541061371));
#8427=CARTESIAN_POINT('Ctrl Pts',(15.9669397999483,8.53240436001509,0.81287245979005));
#8428=CARTESIAN_POINT('Ctrl Pts',(16.4211778776976,8.96603690891341,0.84991950896639));
#8429=CARTESIAN_POINT('Ctrl Pts',(16.589302871581,9.49125972577423,0.88696655814273));
#8430=CARTESIAN_POINT('Ctrl Pts',(16.7574278654643,10.0164825426351,0.92401360731907));
#8431=CARTESIAN_POINT('Ctrl Pts',(16.6394397754816,10.6332956274584,0.961060656495409));
#8432=CARTESIAN_POINT('Ctrl Pts',(16.2893386307264,11.0593900732881,0.998107705671749));
#8433=CARTESIAN_POINT('Ctrl Pts',(15.9392374859711,11.4854845191178,1.03515475484809));
#8434=CARTESIAN_POINT('Ctrl Pts',(15.3570232864432,11.7208603259538,1.07220180402443));
#8435=CARTESIAN_POINT('Ctrl Pts',(14.8091643682469,11.6577936066139,1.10924885320077));
#8436=CARTESIAN_POINT('Ctrl Pts',(14.2613054500506,11.594726887274,1.14629590237711));
#8437=CARTESIAN_POINT('Ctrl Pts',(13.7478018131859,11.2332176417582,1.18334295155345));
#8438=CARTESIAN_POINT('Ctrl Pts',(13.5036737118494,10.7387199750775,1.22039000072979));
#8439=CARTESIAN_POINT('Ctrl Pts',(13.3914507097464,10.5114048385405,1.2374201216166));
#8440=CARTESIAN_POINT('Ctrl Pts',(13.3361505226053,10.255987390206,1.2544502425034));
#8441=CARTESIAN_POINT('Ctrl Pts',(13.3366506987084,10.0003647761852,1.27148036339021));
#8442=CARTESIAN_POINT('Origin',(15.,10.,4.));
#8443=CARTESIAN_POINT('',(13.3341440524774,9.99847620463016,1.97148036339021));
#8444=CARTESIAN_POINT('',(13.3312583494731,10.0000242625446,1.77851963660979));
#8445=CARTESIAN_POINT('',(13.334,10.,4.));
#8446=CARTESIAN_POINT('Ctrl Pts',(13.3312588297318,10.0000242582945,1.77851963660979));
#8447=CARTESIAN_POINT('Ctrl Pts',(13.3311401928165,10.5527978235745,1.74138549538496));
#8448=CARTESIAN_POINT('Ctrl Pts',(13.633172617078,11.1054588469535,1.70425135416013));
#8449=CARTESIAN_POINT('Ctrl Pts',(14.0982990092452,11.4041487296504,1.6671172129353));
#8450=CARTESIAN_POINT('Ctrl Pts',(14.562334523612,11.7021380841302,1.63007016375896));
#8451=CARTESIAN_POINT('Ctrl Pts',(15.1886983700061,11.7473461999417,1.59302311458262));
#8452=CARTESIAN_POINT('Ctrl Pts',(15.6907163851895,11.5190818474979,1.55597606540628));
#8453=CARTESIAN_POINT('Ctrl Pts',(16.1927344003729,11.2908174950541,1.51892901622994));
#8454=CARTESIAN_POINT('Ctrl Pts',(16.5704065843456,10.789080674355,1.4818819670536));
#8455=CARTESIAN_POINT('Ctrl Pts',(16.650879481241,10.2435071243058,1.44483491787726));
#8456=CARTESIAN_POINT('Ctrl Pts',(16.7313523781363,9.69793357425666,1.40778786870092));
#8457=CARTESIAN_POINT('Ctrl Pts',(16.5146259879544,9.10852329485745,1.37074081952458));
#8458=CARTESIAN_POINT('Ctrl Pts',(16.0998923987615,8.74503633532444,1.33369377034824));
#8459=CARTESIAN_POINT('Ctrl Pts',(15.6851588095687,8.38154937579143,1.2966467211719));
#8460=CARTESIAN_POINT('Ctrl Pts',(15.072418021365,8.24398573612463,1.25959967199556));
#8461=CARTESIAN_POINT('Ctrl Pts',(14.5421080170767,8.39530825722336,1.22255262281922));
#8462=CARTESIAN_POINT('Ctrl Pts',(14.0117980127884,8.5466307783221,1.18550557364288));
#8463=CARTESIAN_POINT('Ctrl Pts',(13.5639187924156,8.98683946018636,1.14845852446654));
#8464=CARTESIAN_POINT('Ctrl Pts',(13.4034584631152,9.51445429332549,1.1114114752902));
#8465=CARTESIAN_POINT('Ctrl Pts',(13.3559707829599,9.67060008057741,1.1004475290634));
#8466=CARTESIAN_POINT('Ctrl Pts',(13.3336565018065,9.83440127945886,1.0894835828366));
#8467=CARTESIAN_POINT('Ctrl Pts',(13.3350093517191,9.9985620319516,1.07851963660979));
#8468=CARTESIAN_POINT('Ctrl Pts',(13.3366506987084,10.0003647761852,1.27148036339021));
#8469=CARTESIAN_POINT('Ctrl Pts',(13.3372385975997,9.69991009544355,1.29149729167974));
#8470=CARTESIAN_POINT('Ctrl Pts',(13.4149162099074,9.39917197274857,1.31151421996928));
#8471=CARTESIAN_POINT('Ctrl Pts',(13.5678608709571,9.14345047930851,1.33153114825881));
#8472=CARTESIAN_POINT('Ctrl Pts',(13.8509286972094,8.67016473806549,1.36857819743515));
#8473=CARTESIAN_POINT('Ctrl Pts',(14.3918169155223,8.3510793434248,1.40562524661149));
#8474=CARTESIAN_POINT('Ctrl Pts',(14.9429716248518,8.3322329656282,1.44267229578783));
#8475=CARTESIAN_POINT('Ctrl Pts',(15.4941263341813,8.31338658783161,1.47971934496417));
#8476=CARTESIAN_POINT('Ctrl Pts',(16.0555475345274,8.59477922687911,1.51676639414051));
#8477=CARTESIAN_POINT('Ctrl Pts',(16.3702838693714,9.04762324449391,1.55381344331685));
#8478=CARTESIAN_POINT('Ctrl Pts',(16.6850202042153,9.50046726210872,1.59086049249319));
#8479=CARTESIAN_POINT('Ctrl Pts',(16.7530716735571,10.1247626582908,1.62790754166953));
#8480=CARTESIAN_POINT('Ctrl Pts',(16.543292450279,10.6347816628546,1.66495459084587));
#8481=CARTESIAN_POINT('Ctrl Pts',(16.3335132270009,11.1448006674184,1.70200164002221));
#8482=CARTESIAN_POINT('Ctrl Pts',(15.8459033111031,11.5405432803638,1.73904868919855));
#8483=CARTESIAN_POINT('Ctrl Pts',(15.3036321297176,11.6408859866488,1.77609573837489));
#8484=CARTESIAN_POINT('Ctrl Pts',(14.7613609483321,11.7412286929337,1.81314278755123));
#8485=CARTESIAN_POINT('Ctrl Pts',(14.1644285014591,11.5461714925582,1.85018983672757));
#8486=CARTESIAN_POINT('Ctrl Pts',(13.7860389659804,11.1449881814256,1.88723688590391));
#8487=CARTESIAN_POINT('Ctrl Pts',(13.4992248469807,10.8408966906439,1.91531804506601));
#8488=CARTESIAN_POINT('Ctrl Pts',(13.3379731090858,10.4183768092574,1.94339920422811));
#8489=CARTESIAN_POINT('Ctrl Pts',(13.3341440524774,9.99847620463016,1.97148036339021));
#8490=CARTESIAN_POINT('Origin',(15.,10.,4.));
#8491=CARTESIAN_POINT('',(13.3314908561079,10.0005637456851,2.67148036339021));
#8492=CARTESIAN_POINT('',(13.3350798111394,10.0014222545761,2.4785196366098));
#8493=CARTESIAN_POINT('',(13.334,10.,4.));
#8494=CARTESIAN_POINT('Ctrl Pts',(13.3350798111394,10.0014222545761,2.4785196366098));
#8495=CARTESIAN_POINT('Ctrl Pts',(13.3337246262576,10.1682098032958,2.46738150628601));
#8496=CARTESIAN_POINT('Ctrl Pts',(13.356768377288,10.3346314141306,2.45624337596222));
#8497=CARTESIAN_POINT('Ctrl Pts',(13.4057541973467,10.4930302810831,2.44510524563844));
#8498=CARTESIAN_POINT('Ctrl Pts',(13.568688193619,11.0198880608789,2.4080581964621));
#8499=CARTESIAN_POINT('Ctrl Pts',(14.018625736829,11.4579882343367,2.37101114728576));
#8500=CARTESIAN_POINT('Ctrl Pts',(14.5496393059462,11.6068210159811,2.33396409810942));
#8501=CARTESIAN_POINT('Ctrl Pts',(15.0806528750634,11.7556537976255,2.29691704893308));
#8502=CARTESIAN_POINT('Ctrl Pts',(15.6927424700877,11.6152191874565,2.25986999975674));
#8503=CARTESIAN_POINT('Ctrl Pts',(16.1057667866446,11.2497913234872,2.2228229505804));
#8504=CARTESIAN_POINT('Ctrl Pts',(16.5187911032016,10.884363459518,2.18577590140406));
#8505=CARTESIAN_POINT('Ctrl Pts',(16.7327501412913,10.2939423417484,2.14872885222772));
#8506=CARTESIAN_POINT('Ctrl Pts',(16.6497190718447,9.74875205788567,2.11168180305138));
#8507=CARTESIAN_POINT('Ctrl Pts',(16.5666880023982,9.20356177402293,2.07463475387504));
#8508=CARTESIAN_POINT('Ctrl Pts',(16.1866668254153,8.70360232406701,2.0375877046987));
#8509=CARTESIAN_POINT('Ctrl Pts',(15.6835837346665,8.47769523896532,2.00054065552236));
#8510=CARTESIAN_POINT('Ctrl Pts',(15.1805006439177,8.25178815386362,1.96349360634602));
#8511=CARTESIAN_POINT('Ctrl Pts',(14.5543556394029,8.29993343361615,1.92644655716968));
#8512=CARTESIAN_POINT('Ctrl Pts',(14.0917228863641,8.60009598607672,1.88939950799334));
#8513=CARTESIAN_POINT('Ctrl Pts',(13.6301777134446,8.89955290145806,1.85243955086549));
#8514=CARTESIAN_POINT('Ctrl Pts',(13.3313769101603,9.44984357280461,1.81547959373764));
#8515=CARTESIAN_POINT('Ctrl Pts',(13.3312588297318,10.0000242582945,1.77851963660979));
#8516=CARTESIAN_POINT('Ctrl Pts',(13.3341440524774,9.99847620463016,1.97148036339021));
#8517=CARTESIAN_POINT('Ctrl Pts',(13.3329214925321,9.86440828327876,1.98044625340445));
#8518=CARTESIAN_POINT('Ctrl Pts',(13.3477470486685,9.73060737845345,1.98941214341869));
#8519=CARTESIAN_POINT('Ctrl Pts',(13.379657735774,9.60101344779502,1.99837803343293));
#8520=CARTESIAN_POINT('Ctrl Pts',(13.5115126651307,9.06553144718687,2.03542508260927));
#8521=CARTESIAN_POINT('Ctrl Pts',(13.9350691479286,8.6018768678603,2.07247213178561));
#8522=CARTESIAN_POINT('Ctrl Pts',(14.4564737537651,8.42225523761979,2.10951918096195));
#8523=CARTESIAN_POINT('Ctrl Pts',(14.9778783596017,8.24263360737928,2.14656623013829));
#8524=CARTESIAN_POINT('Ctrl Pts',(15.5971310884769,8.34704492622482,2.18361327931463));
#8525=CARTESIAN_POINT('Ctrl Pts',(16.030812208256,8.68770220147219,2.22066032849097));
#8526=CARTESIAN_POINT('Ctrl Pts',(16.4644933280352,9.02835947671956,2.25770737766731));
#8527=CARTESIAN_POINT('Ctrl Pts',(16.7126028387182,9.60526270836876,2.29475442684365));
#8528=CARTESIAN_POINT('Ctrl Pts',(16.6615859215914,10.1543746894207,2.33180147601999));
#8529=CARTESIAN_POINT('Ctrl Pts',(16.6105690044646,10.7034866704727,2.36884852519633));
#8530=CARTESIAN_POINT('Ctrl Pts',(16.2604256595279,11.2248074009274,2.40589557437267));
#8531=CARTESIAN_POINT('Ctrl Pts',(15.7714095743024,11.4797386889282,2.44294262354901));
#8532=CARTESIAN_POINT('Ctrl Pts',(15.282393489077,11.7346699769289,2.47998967272535));
#8533=CARTESIAN_POINT('Ctrl Pts',(14.6545046635628,11.7232118224755,2.51703672190169));
#8534=CARTESIAN_POINT('Ctrl Pts',(14.1751154010763,11.4506083958144,2.55408377107803));
#8535=CARTESIAN_POINT('Ctrl Pts',(13.6957261385897,11.1780049691532,2.59113082025437));
#8536=CARTESIAN_POINT('Ctrl Pts',(13.3648364391308,10.6442562702842,2.62817786943071));
#8537=CARTESIAN_POINT('Ctrl Pts',(13.3338879771839,10.0936485278662,2.66522491860705));
#8538=CARTESIAN_POINT('Ctrl Pts',(13.3321460805134,10.0626582384328,2.6673100668681));
#8539=CARTESIAN_POINT('Ctrl Pts',(13.3313543571281,10.0316145418291,2.66939521512915));
#8540=CARTESIAN_POINT('Ctrl Pts',(13.3314908561079,10.0005637456851,2.67148036339021));
#8541=CARTESIAN_POINT('Origin',(15.,10.,4.));
#8542=CARTESIAN_POINT('',(13.3358101889457,10.0011694310247,3.37148036339021));
#8543=CARTESIAN_POINT('',(13.3362901345243,9.99914721744613,3.1785196366098));
#8544=CARTESIAN_POINT('',(13.334,10.,4.));
#8545=CARTESIAN_POINT('Ctrl Pts',(13.3362901345243,9.99914721744613,3.1785196366098));
#8546=CARTESIAN_POINT('Ctrl Pts',(13.3378337351605,10.3320266569125,3.15633046801072));
#8547=CARTESIAN_POINT('Ctrl Pts',(13.4345606138998,10.6657320713228,3.13414129941164));
#8548=CARTESIAN_POINT('Ctrl Pts',(13.6203848363125,10.9388080400732,3.11195213081256));
#8549=CARTESIAN_POINT('Ctrl Pts',(13.9306370692944,11.394735840973,3.07490508163622));
#8550=CARTESIAN_POINT('Ctrl Pts',(14.489254042355,11.6816550509133,3.03785803245987));
#8551=CARTESIAN_POINT('Ctrl Pts',(15.0405678095774,11.6682484193642,3.00081098328353));
#8552=CARTESIAN_POINT('Ctrl Pts',(15.5918815767999,11.6548417878151,2.96376393410719));
#8553=CARTESIAN_POINT('Ctrl Pts',(16.1358921381843,11.3411093147767,2.92671688493086));
#8554=CARTESIAN_POINT('Ctrl Pts',(16.4236166138013,10.8706401511932,2.88966983575452));
#8555=CARTESIAN_POINT('Ctrl Pts',(16.7113410894183,10.4001709876096,2.85262278657818));
#8556=CARTESIAN_POINT('Ctrl Pts',(16.7427794792678,9.77296513348092,2.81557573740183));
#8557=CARTESIAN_POINT('Ctrl Pts',(16.5035430536575,9.27608230995051,2.7785286882255));
#8558=CARTESIAN_POINT('Ctrl Pts',(16.2643066280471,8.7791994864201,2.74148163904916));
#8559=CARTESIAN_POINT('Ctrl Pts',(15.7543953869767,8.41263969348797,2.70443458987282));
#8560=CARTESIAN_POINT('Ctrl Pts',(15.207185625858,8.34417010176588,2.66738754069648));
#8561=CARTESIAN_POINT('Ctrl Pts',(14.6599758647393,8.27570051004378,2.63034049152014));
#8562=CARTESIAN_POINT('Ctrl Pts',(14.0754675835721,8.50532111953174,2.59329344234379));
#8563=CARTESIAN_POINT('Ctrl Pts',(13.7211786676559,8.92793911734263,2.55624639316745));
#8564=CARTESIAN_POINT('Ctrl Pts',(13.4734060925949,9.22349775573222,2.5303374743149));
#8565=CARTESIAN_POINT('Ctrl Pts',(13.3382321692202,9.61345004202563,2.50442855546235));
#8566=CARTESIAN_POINT('Ctrl Pts',(13.3350798111394,10.0014222545761,2.4785196366098));
#8567=CARTESIAN_POINT('Ctrl Pts',(13.3314908561079,10.0005637456851,2.67148036339021));
#8568=CARTESIAN_POINT('Ctrl Pts',(13.3337795489059,9.47993177029892,2.70644226430549));
#8569=CARTESIAN_POINT('Ctrl Pts',(13.5970248044157,8.95730385981114,2.74140416522078));
#8570=CARTESIAN_POINT('Ctrl Pts',(14.017753627907,8.65096650012722,2.77636606613607));
#8571=CARTESIAN_POINT('Ctrl Pts',(14.4635749650119,8.3263590007736,2.81341311531241));
#8572=CARTESIAN_POINT('Ctrl Pts',(15.0862248636567,8.24461078803355,2.85046016448875));
#8573=CARTESIAN_POINT('Ctrl Pts',(15.6007287737264,8.44313640296184,2.88750721366509));
#8574=CARTESIAN_POINT('Ctrl Pts',(16.115232683796,8.64166201789014,2.92455426284143));
#8575=CARTESIAN_POINT('Ctrl Pts',(16.5215906052904,9.12046146048677,2.96160131201777));
#8576=CARTESIAN_POINT('Ctrl Pts',(16.6338205503814,9.66039769069899,2.99864836119411));
#8577=CARTESIAN_POINT('Ctrl Pts',(16.7460504954725,10.2003339209112,3.03569541037045));
#8578=CARTESIAN_POINT('Ctrl Pts',(16.5641524641601,10.801406938739,3.07274245954679));
#8579=CARTESIAN_POINT('Ctrl Pts',(16.1713775896356,11.1885175058972,3.10978950872313));
#8580=CARTESIAN_POINT('Ctrl Pts',(15.7786027151111,11.5756280730554,3.14683655789947));
#8581=CARTESIAN_POINT('Ctrl Pts',(15.1749509973745,11.7487761895439,3.18388360707581));
#8582=CARTESIAN_POINT('Ctrl Pts',(14.6367018947022,11.6287153852114,3.22093065625215));
#8583=CARTESIAN_POINT('Ctrl Pts',(14.0984527920298,11.5086545808789,3.25797770542849));
#8584=CARTESIAN_POINT('Ctrl Pts',(13.6256063044218,11.0953848557254,3.29502475460483));
#8585=CARTESIAN_POINT('Ctrl Pts',(13.4345749220722,10.5780515934819,3.33207180378117));
#8586=CARTESIAN_POINT('Ctrl Pts',(13.3668387884629,10.3946149531724,3.34520799031751));
#8587=CARTESIAN_POINT('Ctrl Pts',(13.3345346524356,10.198094631663,3.35834417685386));
#8588=CARTESIAN_POINT('Ctrl Pts',(13.3358101889457,10.0011694310247,3.37148036339021));
#8589=CARTESIAN_POINT('Origin',(15.,10.,4.));
#8590=CARTESIAN_POINT('',(13.3357191812891,9.99878755125724,4.07148036339021));
#8591=CARTESIAN_POINT('',(13.3319678106811,9.99903395442804,3.8785196366098));
#8592=CARTESIAN_POINT('',(13.334,10.,4.));
#8593=CARTESIAN_POINT('Ctrl Pts',(13.3319678106811,9.99903395442804,3.8785196366098));
#8594=CARTESIAN_POINT('Ctrl Pts',(13.3353869165692,10.4944017554198,3.84527942973543));
#8595=CARTESIAN_POINT('Ctrl Pts',(13.5702060291847,10.9925841837293,3.81203922286105));
#8596=CARTESIAN_POINT('Ctrl Pts',(13.956288166515,11.3020614980076,3.77879901598667));
#8597=CARTESIAN_POINT('Ctrl Pts',(14.3865864490088,11.6469817725522,3.74175196681033));
#8598=CARTESIAN_POINT('Ctrl Pts',(15.0047785913624,11.7574988787253,3.70470491763399));
#8599=CARTESIAN_POINT('Ctrl Pts',(15.5279302703839,11.5830313217246,3.66765786845765));
#8600=CARTESIAN_POINT('Ctrl Pts',(16.0510819494053,11.4085637647238,3.63061081928131));
#8601=CARTESIAN_POINT('Ctrl Pts',(16.4791931650947,10.9491115445491,3.59356377010497));
#8602=CARTESIAN_POINT('Ctrl Pts',(16.6163258768942,10.4149568599639,3.55651672092863));
#8603=CARTESIAN_POINT('Ctrl Pts',(16.7534585886938,9.88080217537861,3.51946967175229));
#8604=CARTESIAN_POINT('Ctrl Pts',(16.5996127966036,9.27194502638277,3.48242262257595));
#8605=CARTESIAN_POINT('Ctrl Pts',(16.2252006784518,8.86704729424585,3.44537557339961));
#8606=CARTESIAN_POINT('Ctrl Pts',(15.8507885603,8.46214956210894,3.40832852422327));
#8607=CARTESIAN_POINT('Ctrl Pts',(15.2558101160866,8.26121124683096,3.37128147504694));
#8608=CARTESIAN_POINT('Ctrl Pts',(14.712575218255,8.35619784317566,3.3342344258706));
#8609=CARTESIAN_POINT('Ctrl Pts',(14.1693403204234,8.45118443952036,3.29718737669426));
#8610=CARTESIAN_POINT('Ctrl Pts',(13.6778489689736,8.84209594748775,3.26014032751791));
#8611=CARTESIAN_POINT('Ctrl Pts',(13.4630470397004,9.35001989740103,3.22309327834157));
#8612=CARTESIAN_POINT('Ctrl Pts',(13.3768997895452,9.55372501178734,3.20823539776431));
#8613=CARTESIAN_POINT('Ctrl Pts',(13.3352565386142,9.77625094550465,3.19337751718706));
#8614=CARTESIAN_POINT('Ctrl Pts',(13.3362901345243,9.99914721744613,3.1785196366098));
#8615=CARTESIAN_POINT('Ctrl Pts',(13.3358101889457,10.0011694310247,3.37148036339021));
#8616=CARTESIAN_POINT('Ctrl Pts',(13.3381319570023,9.64272054559026,3.3953912260302));
#8617=CARTESIAN_POINT('Ctrl Pts',(13.4517109778754,9.28293020158332,3.4193020886702));
#8618=CARTESIAN_POINT('Ctrl Pts',(13.6653761754273,8.99826222682056,3.44321295131019));
#8619=CARTESIAN_POINT('Ctrl Pts',(13.9964250882229,8.55720292173609,3.48026000048653));
#8620=CARTESIAN_POINT('Ctrl Pts',(14.5677391909053,8.29648111090055,3.51730704966287));
#8621=CARTESIAN_POINT('Ctrl Pts',(15.1178393123602,8.33542401321063,3.55435409883921));
#8622=CARTESIAN_POINT('Ctrl Pts',(15.6679394338151,8.37436691552071,3.59140114801555));
#8623=CARTESIAN_POINT('Ctrl Pts',(16.1968255740426,8.71297453097641,3.62844819719189));
#8624=CARTESIAN_POINT('Ctrl Pts',(16.4624370016316,9.1962728475463,3.66549524636823));
#8625=CARTESIAN_POINT('Ctrl Pts',(16.7280484292206,9.67957116411619,3.70254229554457));
#8626=CARTESIAN_POINT('Ctrl Pts',(16.7303851441713,10.3075601818003,3.7395893447209));
#8627=CARTESIAN_POINT('Ctrl Pts',(16.4683776782427,10.7928217412326,3.77663639389724));
#8628=CARTESIAN_POINT('Ctrl Pts',(16.2063702123141,11.278083300665,3.81368344307358));
#8629=CARTESIAN_POINT('Ctrl Pts',(15.6800185655062,11.6206174018456,3.85073049224993));
#8630=CARTESIAN_POINT('Ctrl Pts',(15.1302234816933,11.6636529578456,3.88777754142627));
#8631=CARTESIAN_POINT('Ctrl Pts',(14.5804283978804,11.7066885138457,3.92482459060261));
#8632=CARTESIAN_POINT('Ctrl Pts',(14.0071898770624,11.4502255246651,3.96187163977895));
#8633=CARTESIAN_POINT('Ctrl Pts',(13.6728678584929,11.011642030716,3.99891868895529));
#8634=CARTESIAN_POINT('Ctrl Pts',(13.4545961741777,10.7253002625409,4.02310591376693));
#8635=CARTESIAN_POINT('Ctrl Pts',(13.33816275372,10.3613295493415,4.04729313857857));
#8636=CARTESIAN_POINT('Ctrl Pts',(13.3357191812891,9.99878755125724,4.07148036339021));
#8637=CARTESIAN_POINT('Origin',(15.,10.,4.));
#8638=CARTESIAN_POINT('',(13.3314356817851,9.99950756868951,4.77148036339021));
#8639=CARTESIAN_POINT('',(13.3333640758576,10.0014616028283,4.5785196366098));
#8640=CARTESIAN_POINT('',(13.334,10.,4.));
#8641=CARTESIAN_POINT('Ctrl Pts',(13.3333640758576,10.0014616028283,4.5785196366098));
#8642=CARTESIAN_POINT('Ctrl Pts',(13.3323717044974,10.1096548526297,4.57127544063647));
#8643=CARTESIAN_POINT('Ctrl Pts',(13.342005436937,10.2176721573884,4.56403124466314));
#8644=CARTESIAN_POINT('Ctrl Pts',(13.3629079833276,10.3234629266178,4.55678704868981));
#8645=CARTESIAN_POINT('Ctrl Pts',(13.4698042720109,10.8644802934135,4.51973999951348));
#8646=CARTESIAN_POINT('Ctrl Pts',(13.8714174816763,11.3472663593339,4.48269295033713));
#8647=CARTESIAN_POINT('Ctrl Pts',(14.3839371853126,11.5508594856755,4.44564590116079));
#8648=CARTESIAN_POINT('Ctrl Pts',(14.896456888949,11.7544526120171,4.40859885198445));
#8649=CARTESIAN_POINT('Ctrl Pts',(15.5198830865563,11.6788527987799,4.37155180280811));
#8650=CARTESIAN_POINT('Ctrl Pts',(15.9688859313197,11.3586605860333,4.33450475363177));
#8651=CARTESIAN_POINT('Ctrl Pts',(16.417888776083,11.0384683732866,4.29745770445543));
#8652=CARTESIAN_POINT('Ctrl Pts',(16.6924682680023,10.4736837610304,4.26041065527909));
#8653=CARTESIAN_POINT('Ctrl Pts',(16.6669548014878,9.92279750168509,4.22336360610275));
#8654=CARTESIAN_POINT('Ctrl Pts',(16.6414413349734,9.37191124233978,4.18631655692641));
#8655=CARTESIAN_POINT('Ctrl Pts',(16.3158349100251,8.83492333590533,4.14926950775008));
#8656=CARTESIAN_POINT('Ctrl Pts',(15.8391591507847,8.55760253203077,4.11222245857374));
#8657=CARTESIAN_POINT('Ctrl Pts',(15.3624833915443,8.28028172815621,4.07517540939739));
#8658=CARTESIAN_POINT('Ctrl Pts',(14.7347382980116,8.26262802684153,4.03812836022105));
#8659=CARTESIAN_POINT('Ctrl Pts',(14.243230390291,8.5127211782015,4.00108131104471));
#8660=CARTESIAN_POINT('Ctrl Pts',(13.7517224825704,8.76281432956148,3.96403426186837));
#8661=CARTESIAN_POINT('Ctrl Pts',(13.3964517606618,9.2806543335961,3.92698721269204));
#8662=CARTESIAN_POINT('Ctrl Pts',(13.3400186110245,9.82923605707147,3.8899401635157));
#8663=CARTESIAN_POINT('Ctrl Pts',(13.3342197118936,9.88560664953272,3.88613332121373));
#8664=CARTESIAN_POINT('Ctrl Pts',(13.3315762367965,9.94230184361494,3.88232647891177));
#8665=CARTESIAN_POINT('Ctrl Pts',(13.3319678106811,9.99903395442804,3.8785196366098));
#8666=CARTESIAN_POINT('Ctrl Pts',(13.3357191812891,9.99878755125724,4.07148036339021));
#8667=CARTESIAN_POINT('Ctrl Pts',(13.3344199866718,9.80603181113007,4.08434018775491));
#8668=CARTESIAN_POINT('Ctrl Pts',(13.3653436581471,9.61367994289709,4.09720001211961));
#8669=CARTESIAN_POINT('Ctrl Pts',(13.4303165283821,9.43361398475765,4.1100598364843));
#8670=CARTESIAN_POINT('Ctrl Pts',(13.6174927331622,8.91487343146603,4.14710688566065));
#8671=CARTESIAN_POINT('Ctrl Pts',(14.0872506590436,8.49809632360041,4.18415393483699));
#8672=CARTESIAN_POINT('Ctrl Pts',(14.6245913894808,8.3740333046211,4.22120098401333));
#8673=CARTESIAN_POINT('Ctrl Pts',(15.161932119918,8.24997028564179,4.25824803318967));
#8674=CARTESIAN_POINT('Ctrl Pts',(15.7668556549109,8.41862135554878,4.295295082366));
#8675=CARTESIAN_POINT('Ctrl Pts',(16.1625004505648,8.80279825352266,4.33234213154234));
#8676=CARTESIAN_POINT('Ctrl Pts',(16.5581452462186,9.18697515149654,4.36938918071868));
#8677=CARTESIAN_POINT('Ctrl Pts',(16.7445113025333,9.7866778775373,4.40643622989502));
#8678=CARTESIAN_POINT('Ctrl Pts',(16.6363025596002,10.3274343488058,4.44348327907136));
#8679=CARTESIAN_POINT('Ctrl Pts',(16.5280938166672,10.8681908200742,4.4805303282477));
#8680=CARTESIAN_POINT('Ctrl Pts',(16.1253102744864,11.3500010365704,4.51757737742405));
#8681=CARTESIAN_POINT('Ctrl Pts',(15.612297998127,11.5523499865775,4.55462442660038));
#8682=CARTESIAN_POINT('Ctrl Pts',(15.0992857217675,11.7546989365846,4.59167147577672));
#8683=CARTESIAN_POINT('Ctrl Pts',(14.4760447112292,11.6775866201028,4.62871852495306));
#8684=CARTESIAN_POINT('Ctrl Pts',(14.0278200568663,11.3563058200469,4.6657655741294));
#8685=CARTESIAN_POINT('Ctrl Pts',(13.6014795346479,11.0507112421021,4.70100383721634));
#8686=CARTESIAN_POINT('Ctrl Pts',(13.3334825638361,10.5242087120345,4.73624210030327));
#8687=CARTESIAN_POINT('Ctrl Pts',(13.3314356817851,9.99950756868951,4.77148036339021));
#8688=CARTESIAN_POINT('Origin',(15.,10.,4.));
#8689=CARTESIAN_POINT('',(13.3342680156708,10.0015218068924,5.47148036339021));
#8690=CARTESIAN_POINT('',(13.3367225736456,10.0000562476499,5.2785196366098));
#8691=CARTESIAN_POINT('',(13.334,10.,4.));
#8692=CARTESIAN_POINT('Ctrl Pts',(13.3367225736456,10.0000562476499,5.2785196366098));
#8693=CARTESIAN_POINT('Ctrl Pts',(13.3366398710265,10.2746976433381,5.26022440236118));
#8694=CARTESIAN_POINT('Ctrl Pts',(13.4008957839674,10.5493026139045,5.24192916811255));
#8695=CARTESIAN_POINT('Ctrl Pts',(13.5297031058243,10.7892563454686,5.22363393386393));
#8696=CARTESIAN_POINT('Ctrl Pts',(13.7905322989496,11.2751521570498,5.18658688468759));
#8697=CARTESIAN_POINT('Ctrl Pts',(14.3160511791024,11.618962369561,5.14953983551125));
#8698=CARTESIAN_POINT('Ctrl Pts',(14.8657401432864,11.6633318450802,5.11249278633491));
#8699=CARTESIAN_POINT('Ctrl Pts',(15.4154291074705,11.7077013205994,5.07544573715857));
#8700=CARTESIAN_POINT('Ctrl Pts',(15.9892881556857,11.4526300591266,5.03839868798224));
#8701=CARTESIAN_POINT('Ctrl Pts',(16.3246733455339,11.014859134846,5.00135163880589));
#8702=CARTESIAN_POINT('Ctrl Pts',(16.6600585353821,10.5770882105654,4.96430458962956));
#8703=CARTESIAN_POINT('Ctrl Pts',(16.7569698668632,9.95661762347699,4.92725754045321));
#8704=CARTESIAN_POINT('Ctrl Pts',(16.5710529393037,9.43742449587025,4.89021049127687));
#8705=CARTESIAN_POINT('Ctrl Pts',(16.3851360117441,8.91823136826352,4.85316344210053));
#8706=CARTESIAN_POINT('Ctrl Pts',(15.9163908251438,8.50031570013841,4.8161163929242));
#8707=CARTESIAN_POINT('Ctrl Pts',(15.3793527852933,8.37494923148702,4.77906934374785));
#8708=CARTESIAN_POINT('Ctrl Pts',(14.8423147454429,8.24958276283564,4.74202229457151));
#8709=CARTESIAN_POINT('Ctrl Pts',(14.2369838523423,8.41676549365797,4.70497524539517));
#8710=CARTESIAN_POINT('Ctrl Pts',(13.8404080896426,8.79998119290459,4.66792819621883));
#8711=CARTESIAN_POINT('Ctrl Pts',(13.5213789226136,9.10826272905,4.63812534301582));
#8712=CARTESIAN_POINT('Ctrl Pts',(13.3374467232736,9.55635112358934,4.60832248981281));
#8713=CARTESIAN_POINT('Ctrl Pts',(13.3333640758576,10.0014616028283,4.5785196366098));
#8714=CARTESIAN_POINT('Ctrl Pts',(13.3314356817851,9.99950756868951,4.77148036339021));
#8715=CARTESIAN_POINT('Ctrl Pts',(13.3313306149783,9.97257456898871,4.77328914947961));
#8716=CARTESIAN_POINT('Ctrl Pts',(13.3319262698781,9.94564631555734,4.77509793556902));
#8717=CARTESIAN_POINT('Ctrl Pts',(13.3332371996276,9.91875292850695,4.77690672165842));
#8718=CARTESIAN_POINT('Ctrl Pts',(13.3600872949395,9.3679301206525,4.81395377083476));
#8719=CARTESIAN_POINT('Ctrl Pts',(13.6869957837509,8.83173378857331,4.8510008200111));
#8720=CARTESIAN_POINT('Ctrl Pts',(14.1643431130298,8.55557039402238,4.88804786918744));
#8721=CARTESIAN_POINT('Ctrl Pts',(14.6416904423087,8.27940699947144,4.92509491836378));
#8722=CARTESIAN_POINT('Ctrl Pts',(15.2694766120551,8.26327654244874,4.96214196754013));
#8723=CARTESIAN_POINT('Ctrl Pts',(15.7603763023923,8.51456161419294,4.99918901671647));
#8724=CARTESIAN_POINT('Ctrl Pts',(16.2512759927295,8.76584668593715,5.03623606589281));
#8725=CARTESIAN_POINT('Ctrl Pts',(16.6052892036575,9.28454728644825,5.07328311506914));
#8726=CARTESIAN_POINT('Ctrl Pts',(16.6603910866373,9.83326440464277,5.11033016424548));
#8727=CARTESIAN_POINT('Ctrl Pts',(16.7154929696171,10.3819815228373,5.14737721342182));
#8728=CARTESIAN_POINT('Ctrl Pts',(16.4716835246487,10.9607151587152,5.18442426259816));
#8729=CARTESIAN_POINT('Ctrl Pts',(16.0405495150863,11.3045903672043,5.2214713117745));
#8730=CARTESIAN_POINT('Ctrl Pts',(15.6094155055239,11.6484655756935,5.25851836095084));
#8731=CARTESIAN_POINT('Ctrl Pts',(14.9909569313674,11.7574823567937,5.29556541012719));
#8732=CARTESIAN_POINT('Ctrl Pts',(14.4682300563887,11.5817458853773,5.33261245930353));
#8733=CARTESIAN_POINT('Ctrl Pts',(13.94550318141,11.4060094139609,5.36965950847987));
#8734=CARTESIAN_POINT('Ctrl Pts',(13.518508005609,10.9455196900277,5.4067065576562));
#8735=CARTESIAN_POINT('Ctrl Pts',(13.3826717801281,10.4110337562418,5.44375360683254));
#8736=CARTESIAN_POINT('Ctrl Pts',(13.3487842592651,10.2776937494211,5.45299585901843));
#8737=CARTESIAN_POINT('Ctrl Pts',(13.3330175869468,10.1397484432952,5.46223811120432));
#8738=CARTESIAN_POINT('Ctrl Pts',(13.3342680156708,10.0015218068924,5.47148036339021));
#8739=CARTESIAN_POINT('Origin',(15.,10.,4.));
#8740=CARTESIAN_POINT('',(13.3366211461937,9.99956957717865,6.17148036339021));
#8741=CARTESIAN_POINT('',(13.3335705647763,9.99850933114582,5.9785196366098));
#8742=CARTESIAN_POINT('',(13.334,10.,4.));
#8743=CARTESIAN_POINT('Ctrl Pts',(13.3335705647763,9.99850933114582,5.9785196366098));
#8744=CARTESIAN_POINT('Ctrl Pts',(13.3376165322179,10.4369404297967,5.94917336408588));
#8745=CARTESIAN_POINT('Ctrl Pts',(13.5153563455701,10.8782736326066,5.91982709156196));
#8746=CARTESIAN_POINT('Ctrl Pts',(13.8257421415539,11.1856715455913,5.89048081903805));
#8747=CARTESIAN_POINT('Ctrl Pts',(14.2175764993273,11.573733967821,5.85343376986171));
#8748=CARTESIAN_POINT('Ctrl Pts',(14.8208062179761,11.7483462850056,5.81638672068537));
#8749=CARTESIAN_POINT('Ctrl Pts',(15.3593449820839,11.6295918879259,5.77933967150903));
#8750=CARTESIAN_POINT('Ctrl Pts',(15.8978837461918,11.5108374908461,5.7422926223327));
#8751=CARTESIAN_POINT('Ctrl Pts',(16.3717315557589,11.098716379502,5.70524557315635));
#8752=CARTESIAN_POINT('Ctrl Pts',(16.5640176341788,10.5818482415203,5.66819852398001));
#8753=CARTESIAN_POINT('Ctrl Pts',(16.7563037125987,10.0649801035386,5.63115147480367));
#8754=CARTESIAN_POINT('Ctrl Pts',(16.6670280598714,9.44336493891926,5.59410442562733));
#8755=CARTESIAN_POINT('Ctrl Pts',(16.3370503780492,9.0015037195829,5.55705737645099));
#8756=CARTESIAN_POINT('Ctrl Pts',(16.0070726962269,8.55964250024654,5.52001032727465));
#8757=CARTESIAN_POINT('Ctrl Pts',(15.4363929853096,8.29753522619313,5.48296327809831));
#8758=CARTESIAN_POINT('Ctrl Pts',(14.8862000675362,8.33514321590732,5.44591622892197));
#8759=CARTESIAN_POINT('Ctrl Pts',(14.3360071497627,8.37275120562152,5.40886917974563));
#8760=CARTESIAN_POINT('Ctrl Pts',(13.8063010251331,8.71007445910332,5.37182213056929));
#8761=CARTESIAN_POINT('Ctrl Pts',(13.5395177158672,9.1927267911698,5.33477508139295));
#8762=CARTESIAN_POINT('Ctrl Pts',(13.4044820962327,9.43702714454645,5.31602326646523));
#8763=CARTESIAN_POINT('Ctrl Pts',(13.3368073402131,9.71856082903702,5.29727145153751));
#8764=CARTESIAN_POINT('Ctrl Pts',(13.3367225736456,10.0000562476499,5.2785196366098));
#8765=CARTESIAN_POINT('Ctrl Pts',(13.3342680156708,10.0015218068924,5.47148036339021));
#8766=CARTESIAN_POINT('Ctrl Pts',(13.3380298603082,9.58567472908586,5.49928516038066));
#8767=CARTESIAN_POINT('Ctrl Pts',(13.4958089693912,9.16728140562092,5.52708995737111));
#8768=CARTESIAN_POINT('Ctrl Pts',(13.7775518139329,8.86407757611185,5.55489475436156));
#8769=CARTESIAN_POINT('Ctrl Pts',(14.1529453483797,8.4600894734066,5.5919418035379));
#8770=CARTESIAN_POINT('Ctrl Pts',(14.7484096924343,8.26059541163487,5.62898885271425));
#8771=CARTESIAN_POINT('Ctrl Pts',(15.2914125868251,8.35689987529541,5.66603590189058));
#8772=CARTESIAN_POINT('Ctrl Pts',(15.834415481216,8.45320433895594,5.70308295106692));
#8773=CARTESIAN_POINT('Ctrl Pts',(16.3249569259433,8.84530732804875,5.74013000024326));
#8774=CARTESIAN_POINT('Ctrl Pts',(16.5385257988885,9.35375106326425,5.7771770494196));
#8775=CARTESIAN_POINT('Ctrl Pts',(16.7520946718337,9.86219479847975,5.81422409859594));
#8776=CARTESIAN_POINT('Ctrl Pts',(16.6886909729969,10.4869792798179,5.85127114777229));
#8777=CARTESIAN_POINT('Ctrl Pts',(16.3773333216744,10.9421529858403,5.88831819694863));
#8778=CARTESIAN_POINT('Ctrl Pts',(16.0659756703518,11.3973266918625,5.92536524612497));
#8779=CARTESIAN_POINT('Ctrl Pts',(15.5066640665436,11.6828896225689,5.9624122953013));
#8780=CARTESIAN_POINT('Ctrl Pts',(14.9553843754809,11.6681452986554,5.99945934447764));
#8781=CARTESIAN_POINT('Ctrl Pts',(14.4041046844183,11.6534009747418,6.03650639365398));
#8782=CARTESIAN_POINT('Ctrl Pts',(13.8608569061013,11.3383493962082,6.07355344283033));
#8783=CARTESIAN_POINT('Ctrl Pts',(13.5742748086562,10.8671833862294,6.11060049200666));
#8784=CARTESIAN_POINT('Ctrl Pts',(13.4172935139586,10.6090924205921,6.13089378246785));
#8785=CARTESIAN_POINT('Ctrl Pts',(13.3373254782368,10.3041588809966,6.15118707292903));
#8786=CARTESIAN_POINT('Ctrl Pts',(13.3366211461937,9.99956957717865,6.17148036339021));
#8787=CARTESIAN_POINT('Origin',(15.,10.,4.));
#8788=CARTESIAN_POINT('',(13.3326898978632,9.99870038716915,6.87148036339021));
#8789=CARTESIAN_POINT('',(13.3318213113649,10.0008675364682,6.6785196366098));
#8790=CARTESIAN_POINT('',(13.334,10.,4.));
#8791=CARTESIAN_POINT('Ctrl Pts',(13.3318213113649,10.0008675364682,6.6785196366098));
#8792=CARTESIAN_POINT('Ctrl Pts',(13.3315052103317,10.0507838401085,6.67516937498693));
#8793=CARTESIAN_POINT('Ctrl Pts',(13.3335514732033,10.1006738678638,6.67181911336406));
#8794=CARTESIAN_POINT('Ctrl Pts',(13.3380445549174,10.1503425512859,6.66846885174119));
#8795=CARTESIAN_POINT('Ctrl Pts',(13.3877288595927,10.6995767199555,6.63142180256485));
#8796=CARTESIAN_POINT('Ctrl Pts',(13.7366062926716,11.2217452545238,6.59437475338851));
#8797=CARTESIAN_POINT('Ctrl Pts',(14.2250023217333,11.4778622839724,6.55732770421217));
#8798=CARTESIAN_POINT('Ctrl Pts',(14.713398350795,11.7339793134211,6.52028065503583));
#8799=CARTESIAN_POINT('Ctrl Pts',(15.3413129758397,11.7240448377502,6.48323360585949));
#8800=CARTESIAN_POINT('Ctrl Pts',(15.8213622031389,11.4526054920116,6.44618655668315));
#8801=CARTESIAN_POINT('Ctrl Pts',(16.3014114304382,11.181166146273,6.40913950750681));
#8802=CARTESIAN_POINT('Ctrl Pts',(16.633595259992,10.6482219304667,6.37209245833047));
#8803=CARTESIAN_POINT('Ctrl Pts',(16.665879658905,10.0976909688753,6.33504540915413));
#8804=CARTESIAN_POINT('Ctrl Pts',(16.6981640578181,9.54716000728396,6.29799835997779));
#8805=CARTESIAN_POINT('Ctrl Pts',(16.4305490260904,8.9790422999075,6.26095131080145));
#8806=CARTESIAN_POINT('Ctrl Pts',(15.9855167048731,8.65335404348968,6.22390426162511));
#8807=CARTESIAN_POINT('Ctrl Pts',(15.5404843836558,8.32766578707186,6.18685721244877));
#8808=CARTESIAN_POINT('Ctrl Pts',(14.9180347729489,8.24440698161268,6.14981016327243));
#8809=CARTESIAN_POINT('Ctrl Pts',(14.4030507388859,8.44168356099275,6.11276311409609));
#8810=CARTESIAN_POINT('Ctrl Pts',(13.8880667048228,8.63896014037284,6.07571606491975));
#8811=CARTESIAN_POINT('Ctrl Pts',(13.4805482474035,9.11677210459218,6.03866901574341));
#8812=CARTESIAN_POINT('Ctrl Pts',(13.367008517143,9.65643435033934,6.00162196656707));
#8813=CARTESIAN_POINT('Ctrl Pts',(13.3434076063187,9.76861112324408,5.99392118991465));
#8814=CARTESIAN_POINT('Ctrl Pts',(13.3325088595262,9.88346030863584,5.98622041326222));
#8815=CARTESIAN_POINT('Ctrl Pts',(13.3335705647763,9.99850933114582,5.9785196366098));
#8816=CARTESIAN_POINT('Ctrl Pts',(13.3366211461937,9.99956957717865,6.17148036339021));
#8817=CARTESIAN_POINT('Ctrl Pts',(13.3360396629134,9.74810637986497,6.18823412210536));
#8818=CARTESIAN_POINT('Ctrl Pts',(13.3894830746076,9.49687780824835,6.20498788082052));
#8819=CARTESIAN_POINT('Ctrl Pts',(13.4982177136245,9.27243602933048,6.22174163953568));
#8820=CARTESIAN_POINT('Ctrl Pts',(13.7386591326111,8.77613512383438,6.25878868871202));
#8821=CARTESIAN_POINT('Ctrl Pts',(14.2494583871574,8.41081375426625,6.29583573788837));
#8822=CARTESIAN_POINT('Ctrl Pts',(14.7968327516103,8.34367207785079,6.33288278706471));
#8823=CARTESIAN_POINT('Ctrl Pts',(15.3442071160632,8.27653040143534,6.36992983624105));
#8824=CARTESIAN_POINT('Ctrl Pts',(15.9281565904228,8.50756841817255,6.40697688541738));
#8825=CARTESIAN_POINT('Ctrl Pts',(16.2814190520273,8.93104500588939,6.44402393459372));
#8826=CARTESIAN_POINT('Ctrl Pts',(16.6346815136318,9.35452159360624,6.48107098377006));
#8827=CARTESIAN_POINT('Ctrl Pts',(16.7572569624813,9.97043675230272,6.51811803294641));
#8828=CARTESIAN_POINT('Ctrl Pts',(16.5930450226178,10.4968974925493,6.55516508212274));
#8829=CARTESIAN_POINT('Ctrl Pts',(16.4288330827542,11.0233582327959,6.59221213129908));
#8830=CARTESIAN_POINT('Ctrl Pts',(15.9778337541777,11.4603645545926,6.62925918047542));
#8831=CARTESIAN_POINT('Ctrl Pts',(15.4464605454363,11.6079088474927,6.66630622965176));
#8832=CARTESIAN_POINT('Ctrl Pts',(14.9150873366949,11.7554531403928,6.70335327882809));
#8833=CARTESIAN_POINT('Ctrl Pts',(14.3033402477887,11.6135354043964,6.74040032800444));
#8834=CARTESIAN_POINT('Ctrl Pts',(13.891203767925,11.2471055880722,6.77744737718078));
#8835=CARTESIAN_POINT('Ctrl Pts',(13.5425082146664,10.9370809875421,6.80879170591726));
#8836=CARTESIAN_POINT('Ctrl Pts',(13.336700189492,10.4663436055774,6.84013603465374));
#8837=CARTESIAN_POINT('Ctrl Pts',(13.3326898978632,9.99870038716915,6.87148036339021));
#8838=CARTESIAN_POINT('Origin',(15.,10.,4.));
#8839=CARTESIAN_POINT('',(13.3325428889984,10.0012066618994,7.57148036339021));
#8840=CARTESIAN_POINT('',(13.3361815072522,10.0009395500142,7.3785196366098));
#8841=CARTESIAN_POINT('',(13.334,10.,4.));
#8842=CARTESIAN_POINT('',(16.2690708798524,11.0793586530485,8.));
#8843=CARTESIAN_POINT('Ctrl Pts',(13.3325428889984,10.0012066618994,7.57148036339021));
#8844=CARTESIAN_POINT('Ctrl Pts',(13.336490896492,9.52850371015197,7.60317909473112));
#8845=CARTESIAN_POINT('Ctrl Pts',(13.5475479048343,9.05282868422974,7.63487782607203));
#8846=CARTESIAN_POINT('Ctrl Pts',(13.9031583859685,8.74254052399572,7.66657655741294));
#8847=CARTESIAN_POINT('Ctrl Pts',(14.3187686777658,8.37989948933103,7.70362360658928));
#8848=CARTESIAN_POINT('Ctrl Pts',(14.9318266387037,8.24316275503293,7.74067065576562));
#8849=CARTESIAN_POINT('Ctrl Pts',(15.4617848325985,8.39611213748269,7.77771770494196));
#8850=CARTESIAN_POINT('Ctrl Pts',(15.9917430264934,8.54906151993244,7.8147647541183));
#8851=CARTESIAN_POINT('Ctrl Pts',(16.4386014533451,8.99169701913006,7.85181180329464));
#8852=CARTESIAN_POINT('Ctrl Pts',(16.5976641540082,9.51876914569494,7.88885885247098));
#8853=CARTESIAN_POINT('Ctrl Pts',(16.7567268546712,10.0458412722598,7.92590590164732));
#8854=CARTESIAN_POINT('Ctrl Pts',(16.6279938291456,10.657350026192,7.96295295082366));
#8855=CARTESIAN_POINT('Ctrl Pts',(16.2690708798524,11.0793586530485,8.));
#8856=CARTESIAN_POINT('',(13.7285471518004,11.0812363616735,8.));
#8857=CARTESIAN_POINT('Origin',(15.,10.,8.));
#8858=CARTESIAN_POINT('Ctrl Pts',(13.7285463279864,11.0812370110871,8.));
#8859=CARTESIAN_POINT('Ctrl Pts',(14.0794405795174,11.4928283988345,7.96367382485347));
#8860=CARTESIAN_POINT('Ctrl Pts',(14.6494732486073,11.7187788632783,7.92734764970694));
#8861=CARTESIAN_POINT('Ctrl Pts',(15.1869067772186,11.6581102602073,7.89102147456041));
#8862=CARTESIAN_POINT('Ctrl Pts',(15.7350053943497,11.5962377203,7.85397442538407));
#8863=CARTESIAN_POINT('Ctrl Pts',(16.2491982074161,11.2362576290369,7.81692737620773));
#8864=CARTESIAN_POINT('Ctrl Pts',(16.4944802724612,10.7424222627658,7.77988032703139));
#8865=CARTESIAN_POINT('Ctrl Pts',(16.7397623375063,10.2485868964947,7.74283327785505));
#8866=CARTESIAN_POINT('Ctrl Pts',(16.71613365453,9.6208962552156,7.70578622867871));
#8867=CARTESIAN_POINT('Ctrl Pts',(16.4342383674864,9.14688996574335,7.66873917950237));
#8868=CARTESIAN_POINT('Ctrl Pts',(16.1523430804427,8.6728836762711,7.63169213032603));
#8869=CARTESIAN_POINT('Ctrl Pts',(15.6121811893316,8.35256173860573,7.59464508114969));
#8870=CARTESIAN_POINT('Ctrl Pts',(15.0610619107686,8.3323961960037,7.55759803197335));
#8871=CARTESIAN_POINT('Ctrl Pts',(14.5099426322055,8.31223065340166,7.52055098279701));
#8872=CARTESIAN_POINT('Ctrl Pts',(13.9478659661905,8.59222150586297,7.48350393362067));
#8873=CARTESIAN_POINT('Ctrl Pts',(13.6320379889576,9.04429107975044,7.44645688444433));
#8874=CARTESIAN_POINT('Ctrl Pts',(13.4389818253369,9.32062764242292,7.42381113516615));
#8875=CARTESIAN_POINT('Ctrl Pts',(13.3379367298706,9.66126159097544,7.40116538588797));
#8876=CARTESIAN_POINT('Ctrl Pts',(13.3361815072522,10.0009395500142,7.3785196366098));
#8877=CARTESIAN_POINT('Origin',(-15.,10.,4.));
#8878=CARTESIAN_POINT('',(-16.6671909719797,10.0013492775649,0.571480363390205));
#8879=CARTESIAN_POINT('',(-16.6635931317265,10.000664586652,0.378519636609791));
#8880=CARTESIAN_POINT('',(-16.666,10.,4.));
#8881=CARTESIAN_POINT('',(-13.3882904778579,9.57816067485776,0.));
#8882=CARTESIAN_POINT('Ctrl Pts',(-16.6635931317265,10.000664586652,0.378519636609791));
#8883=CARTESIAN_POINT('Ctrl Pts',(-16.6645712763617,10.2261440155287,0.363487571935547));
#8884=CARTESIAN_POINT('Ctrl Pts',(-16.6219037410329,10.4512893271606,0.348455507261303));
#8885=CARTESIAN_POINT('Ctrl Pts',(-16.5338109814408,10.6570298951176,0.333423442587058));
#8886=CARTESIAN_POINT('Ctrl Pts',(-16.3167032941462,11.1640847211743,0.296376393410719));
#8887=CARTESIAN_POINT('Ctrl Pts',(-15.8236858537848,11.5532764409388,0.259329344234379));
#8888=CARTESIAN_POINT('Ctrl Pts',(-15.279847491745,11.6454139691312,0.22228229505804));
#8889=CARTESIAN_POINT('Ctrl Pts',(-14.7360091297051,11.7375514973235,0.1852352458817));
#8890=CARTESIAN_POINT('Ctrl Pts',(-14.1413498459868,11.5326348339436,0.148188196705361));
#8891=CARTESIAN_POINT('Ctrl Pts',(-13.7693512524429,11.1267739948468,0.11114114752902));
#8892=CARTESIAN_POINT('Ctrl Pts',(-13.397352658899,10.72091315575,0.0740940983526811));
#8893=CARTESIAN_POINT('Ctrl Pts',(-13.2480147555294,10.1141081409362,0.0370470491763408));
#8894=CARTESIAN_POINT('Ctrl Pts',(-13.3882904778579,9.57816067485778,1.59594559789866E-15));
#8895=CARTESIAN_POINT('',(-15.675077185675,8.47690223774664,0.));
#8896=CARTESIAN_POINT('Origin',(-15.,10.,0.));
#8897=CARTESIAN_POINT('Ctrl Pts',(-15.676409110153,8.47417610875464,5.20417042793042E-17));
#8898=CARTESIAN_POINT('Ctrl Pts',(-15.1816815462137,8.25559244463078,0.0363261751465299));
#8899=CARTESIAN_POINT('Ctrl Pts',(-14.5700634796721,8.29934581648217,0.0726523502930598));
#8900=CARTESIAN_POINT('Ctrl Pts',(-14.1121756761023,8.58718997742447,0.10897852543959));
#8901=CARTESIAN_POINT('Ctrl Pts',(-13.6452013275045,8.88074625585282,0.14602557461593));
#8902=CARTESIAN_POINT('Ctrl Pts',(-13.338119175407,9.42817715635473,0.18307262379227));
#8903=CARTESIAN_POINT('Ctrl Pts',(-13.3313948226923,9.97953138687446,0.22011967296861));
#8904=CARTESIAN_POINT('Ctrl Pts',(-13.3246704699776,10.5308856173942,0.257166722144951));
#8905=CARTESIAN_POINT('Ctrl Pts',(-13.6183039166457,11.0861631779317,0.294213771321291));
#8906=CARTESIAN_POINT('Ctrl Pts',(-14.0779464201314,11.3909182993711,0.331260820497631));
#8907=CARTESIAN_POINT('Ctrl Pts',(-14.537588923617,11.6956734208104,0.368307869673971));
#8908=CARTESIAN_POINT('Ctrl Pts',(-15.1632404839201,11.7499061031516,0.405354918850311));
#8909=CARTESIAN_POINT('Ctrl Pts',(-15.6685313154342,11.5289529396842,0.442401968026651));
#8910=CARTESIAN_POINT('Ctrl Pts',(-16.1738221469483,11.3079997762168,0.479449017202991));
#8911=CARTESIAN_POINT('Ctrl Pts',(-16.5587522496733,10.8118607669409,0.516496066379331));
#8912=CARTESIAN_POINT('Ctrl Pts',(-16.6471577882404,10.2675275099722,0.55354311555567));
#8913=CARTESIAN_POINT('Ctrl Pts',(-16.6614256997248,10.1796766936732,0.559522198167182));
#8914=CARTESIAN_POINT('Ctrl Pts',(-16.6679699620053,10.0905705497967,0.565501280778694));
#8915=CARTESIAN_POINT('Ctrl Pts',(-16.6671909719797,10.0013492775649,0.571480363390205));
#8916=CARTESIAN_POINT('Origin',(-15.,10.,4.));
#8917=CARTESIAN_POINT('',(-16.6633491135953,10.0003647770189,1.27148036339021));
#8918=CARTESIAN_POINT('',(-16.6649907195691,9.99856203207469,1.07851963660979));
#8919=CARTESIAN_POINT('',(-16.666,10.,4.));
#8920=CARTESIAN_POINT('Ctrl Pts',(-16.6649907195691,9.99856203207469,1.07851963660979));
#8921=CARTESIAN_POINT('Ctrl Pts',(-16.6617723069357,10.3890986075708,1.05243653366026));
#8922=CARTESIAN_POINT('Ctrl Pts',(-16.5246077087442,10.7816701084545,1.02635343071072));
#8923=CARTESIAN_POINT('Ctrl Pts',(-16.2737774517755,11.0780444210991,1.00027032776118));
#8924=CARTESIAN_POINT('Ctrl Pts',(-15.9175115242587,11.4989986977583,0.963223278584839));
#8925=CARTESIAN_POINT('Ctrl Pts',(-15.3319382306252,11.7258862342935,0.9261762294085));
#8926=CARTESIAN_POINT('Ctrl Pts',(-14.7850529907541,11.654845590621,0.88912918023216));
#8927=CARTESIAN_POINT('Ctrl Pts',(-14.238167750883,11.5838049469485,0.85208213105582));
#8928=CARTESIAN_POINT('Ctrl Pts',(-13.7299705647742,11.2148361230683,0.815035081879479));
#8929=CARTESIAN_POINT('Ctrl Pts',(-13.4930724270708,10.7168466467109,0.77798803270314));
#8930=CARTESIAN_POINT('Ctrl Pts',(-13.2561742893673,10.2188571703535,0.7409409835268));
#8931=CARTESIAN_POINT('Ctrl Pts',(-13.2905752000691,9.59184704151887,0.703893934350459));
#8932=CARTESIAN_POINT('Ctrl Pts',(-13.5804933523073,9.12271316008998,0.666846885174119));
#8933=CARTESIAN_POINT('Ctrl Pts',(-13.8704115045454,8.6535792786611,0.62979983599778));
#8934=CARTESIAN_POINT('Ctrl Pts',(-14.4158468983198,8.34232164463794,0.59275278682144));
#8935=CARTESIAN_POINT('Ctrl Pts',(-14.9672366360564,8.33153869325115,0.5557057376451));
#8936=CARTESIAN_POINT('Ctrl Pts',(-15.5186263737931,8.32075574186434,0.518658688468759));
#8937=CARTESIAN_POINT('Ctrl Pts',(-16.075970455492,8.61044747311391,0.481611639292419));
#8938=CARTESIAN_POINT('Ctrl Pts',(-16.3840435292275,9.06775230491307,0.444564590116079));
#8939=CARTESIAN_POINT('Ctrl Pts',(-16.5671140866562,9.33950293036427,0.422549605613983));
#8940=CARTESIAN_POINT('Ctrl Pts',(-16.662160604695,9.67044207631607,0.400534621111887));
#8941=CARTESIAN_POINT('Ctrl Pts',(-16.6635931317265,10.000664586652,0.378519636609791));
#8942=CARTESIAN_POINT('Ctrl Pts',(-16.6671909719797,10.0013492775649,0.571480363390205));
#8943=CARTESIAN_POINT('Ctrl Pts',(-16.6631432546885,9.53774579812301,0.602548329955034));
#8944=CARTESIAN_POINT('Ctrl Pts',(-16.4613710095151,9.07103390472509,0.633616296519862));
#8945=CARTESIAN_POINT('Ctrl Pts',(-16.1180469662142,8.76117513340022,0.66468426308469));
#8946=CARTESIAN_POINT('Ctrl Pts',(-15.7086496312117,8.39168351845854,0.70173131226103));
#8947=CARTESIAN_POINT('Ctrl Pts',(-15.0979739867974,8.24522779323672,0.73877836143737));
#8948=CARTESIAN_POINT('Ctrl Pts',(-14.5655171497087,8.3888161695707,0.77582541061371));
#8949=CARTESIAN_POINT('Ctrl Pts',(-14.03306031262,8.53240454590468,0.81287245979005));
#8950=CARTESIAN_POINT('Ctrl Pts',(-13.5788222828569,8.96603702379445,0.84991950896639));
#8951=CARTESIAN_POINT('Ctrl Pts',(-13.4106973070842,9.49125977655298,0.88696655814273));
#8952=CARTESIAN_POINT('Ctrl Pts',(-13.2425723313114,10.0164825293115,0.92401360731907));
#8953=CARTESIAN_POINT('Ctrl Pts',(-13.3605604095291,10.6332955569388,0.961060656495409));
#8954=CARTESIAN_POINT('Ctrl Pts',(-13.7106615151752,11.0593899574044,0.998107705671749));
#8955=CARTESIAN_POINT('Ctrl Pts',(-14.0607626208212,11.48548435787,1.03515475484809));
#8956=CARTESIAN_POINT('Ctrl Pts',(-14.6429767538956,11.7208601311739,1.07220180402443));
#8957=CARTESIAN_POINT('Ctrl Pts',(-15.1908356100492,11.6577934174094,1.10924885320077));
#8958=CARTESIAN_POINT('Ctrl Pts',(-15.7386944662028,11.5947267036449,1.14629590237711));
#8959=CARTESIAN_POINT('Ctrl Pts',(-16.2521980454357,11.2332175028119,1.18334295155345));
#8960=CARTESIAN_POINT('Ctrl Pts',(-16.4963261193042,10.7387198928195,1.22039000072979));
#8961=CARTESIAN_POINT('Ctrl Pts',(-16.6085491087805,10.5114047823413,1.2374201216166));
#8962=CARTESIAN_POINT('Ctrl Pts',(-16.663849289669,10.2559873626026,1.2544502425034));
#8963=CARTESIAN_POINT('Ctrl Pts',(-16.6633491135953,10.0003647770189,1.27148036339021));
#8964=CARTESIAN_POINT('Origin',(-15.,10.,4.));
#8965=CARTESIAN_POINT('',(-16.6658557594656,9.99847620480149,1.97148036339021));
#8966=CARTESIAN_POINT('',(-16.6687417212197,10.000024262485,1.77851963660979));
#8967=CARTESIAN_POINT('',(-16.666,10.,4.));
#8968=CARTESIAN_POINT('Ctrl Pts',(-16.6687412413332,10.0000242582383,1.77851963660979));
#8969=CARTESIAN_POINT('Ctrl Pts',(-16.6688598782876,10.5527978471161,1.74138549538496));
#8970=CARTESIAN_POINT('Ctrl Pts',(-16.3668274413062,11.1054588942412,1.70425135416013));
#8971=CARTESIAN_POINT('Ctrl Pts',(-15.9017010292556,11.4041487895867,1.6671172129353));
#8972=CARTESIAN_POINT('Ctrl Pts',(-15.4376654950521,11.7021381566853,1.63007016375896));
#8973=CARTESIAN_POINT('Ctrl Pts',(-14.8113016216914,11.7473462740701,1.59302311458262));
#8974=CARTESIAN_POINT('Ctrl Pts',(-14.3092835852333,11.5190819120405,1.55597606540628));
#8975=CARTESIAN_POINT('Ctrl Pts',(-13.8072655487753,11.2908175500109,1.51892901622994));
#8976=CARTESIAN_POINT('Ctrl Pts',(-13.42959334922,10.789080708567,1.4818819670536));
#8977=CARTESIAN_POINT('Ctrl Pts',(-13.3491204486805,10.2435071350204,1.44483491787726));
#8978=CARTESIAN_POINT('Ctrl Pts',(-13.268647548141,9.69793356147377,1.40778786870092));
#8979=CARTESIAN_POINT('Ctrl Pts',(-13.4853739466174,9.10852325582452,1.37074081952458));
#8980=CARTESIAN_POINT('Ctrl Pts',(-13.9001075538765,8.7450362812419,1.33369377034824));
#8981=CARTESIAN_POINT('Ctrl Pts',(-14.3148411611356,8.38154930665928,1.2966467211719));
#8982=CARTESIAN_POINT('Ctrl Pts',(-14.9275819771775,8.24398566314329,1.25959967199556));
#8983=CARTESIAN_POINT('Ctrl Pts',(-15.4578920033439,8.39530818992637,1.22255262281922));
#8984=CARTESIAN_POINT('Ctrl Pts',(-15.9882020295104,8.54663071670945,1.18550557364288));
#8985=CARTESIAN_POINT('Ctrl Pts',(-16.4360812658015,8.98683941379159,1.14845852446654));
#8986=CARTESIAN_POINT('Ctrl Pts',(-16.596541603247,9.51445427072422,1.1114114752902));
#8987=CARTESIAN_POINT('Ctrl Pts',(-16.6440292858128,9.67060006501775,1.1004475290634));
#8988=CARTESIAN_POINT('Ctrl Pts',(-16.6663435686959,9.8344012716919,1.0894835828366));
#8989=CARTESIAN_POINT('Ctrl Pts',(-16.6649907195691,9.99856203207469,1.07851963660979));
#8990=CARTESIAN_POINT('Ctrl Pts',(-16.6633491135953,10.0003647770189,1.27148036339021));
#8991=CARTESIAN_POINT('Ctrl Pts',(-16.6627612147386,9.69991012970163,1.29149729167974));
#8992=CARTESIAN_POINT('Ctrl Pts',(-16.5850836111443,9.39917204021162,1.31151421996928));
#8993=CARTESIAN_POINT('Ctrl Pts',(-16.4321389673375,9.14345057537975,1.33153114825881));
#8994=CARTESIAN_POINT('Ctrl Pts',(-16.149071172998,8.67016488708435,1.36857819743515));
#8995=CARTESIAN_POINT('Ctrl Pts',(-15.6081830158149,8.3510795296454,1.40562524661149));
#8996=CARTESIAN_POINT('Ctrl Pts',(-15.0570283687243,8.33223315424277,1.44267229578783));
#8997=CARTESIAN_POINT('Ctrl Pts',(-14.5058737216337,8.31338677884013,1.47971934496417));
#8998=CARTESIAN_POINT('Ctrl Pts',(-13.9444525846355,8.59477938547379,1.51676639414051));
#8999=CARTESIAN_POINT('Ctrl Pts',(-13.6297162853131,9.04762335182059,1.55381344331685));
#9000=CARTESIAN_POINT('Ctrl Pts',(-13.3149799859908,9.5004673181674,1.59086049249319));
#9001=CARTESIAN_POINT('Ctrl Pts',(-13.2469285243443,10.1247626442273,1.62790754166953));
#9002=CARTESIAN_POINT('Ctrl Pts',(-13.4567077239444,10.634781591296,1.66495459084587));
#9003=CARTESIAN_POINT('Ctrl Pts',(-13.6664869235445,11.1448005383647,1.70200164002221));
#9004=CARTESIAN_POINT('Ctrl Pts',(-14.1540967843911,11.5405431064421,1.73904868919855));
#9005=CARTESIAN_POINT('Ctrl Pts',(-14.6963679045584,11.6408858013554,1.77609573837489));
#9006=CARTESIAN_POINT('Ctrl Pts',(-15.2386390247256,11.7412284962687,1.81314278755123));
#9007=CARTESIAN_POINT('Ctrl Pts',(-15.8355714042134,11.5461713180179,1.85018983672757));
#9008=CARTESIAN_POINT('Ctrl Pts',(-16.2139608969767,11.1449880521985,1.88723688590391));
#9009=CARTESIAN_POINT('Ctrl Pts',(-16.5007749835987,10.8408965957637,1.91531804506601));
#9010=CARTESIAN_POINT('Ctrl Pts',(-16.6620267032898,10.4183767620469,1.94339920422811));
#9011=CARTESIAN_POINT('Ctrl Pts',(-16.6658557594656,9.99847620480149,1.97148036339021));
#9012=CARTESIAN_POINT('Origin',(-15.,10.,4.));
#9013=CARTESIAN_POINT('',(-16.6685089555354,10.000563745621,2.67148036339021));
#9014=CARTESIAN_POINT('',(-16.6649202598041,10.0014222546351,2.47851963660979));
#9015=CARTESIAN_POINT('',(-16.666,10.,4.));
#9016=CARTESIAN_POINT('Ctrl Pts',(-16.6649202598041,10.0014222546351,2.47851963660979));
#9017=CARTESIAN_POINT('Ctrl Pts',(-16.6662754447434,10.1682098104616,2.46738150628601));
#9018=CARTESIAN_POINT('Ctrl Pts',(-16.6432316927311,10.3346314283879,2.45624337596222));
#9019=CARTESIAN_POINT('Ctrl Pts',(-16.5942458705854,10.4930303020904,2.44510524563844));
#9020=CARTESIAN_POINT('Ctrl Pts',(-16.431311867371,11.0198881043375,2.4080581964621));
#9021=CARTESIAN_POINT('Ctrl Pts',(-15.9813743049921,11.4579882964685,2.37101114728576));
#9022=CARTESIAN_POINT('Ctrl Pts',(-15.4503607132462,11.6068210844527,2.33396409810942));
#9023=CARTESIAN_POINT('Ctrl Pts',(-14.9193471215002,11.7556538724368,2.29691704893308));
#9024=CARTESIAN_POINT('Ctrl Pts',(-14.3072575003873,11.6152192562742,2.25986999975674));
#9025=CARTESIAN_POINT('Ctrl Pts',(-13.8942331662336,11.2497913767376,2.2228229505804));
#9026=CARTESIAN_POINT('Ctrl Pts',(-13.48120883208,10.8843634972009,2.18577590140406));
#9027=CARTESIAN_POINT('Ctrl Pts',(-13.2672497848857,10.2939423542903,2.14872885222772));
#9028=CARTESIAN_POINT('Ctrl Pts',(-13.350280857865,9.7487520471889,2.11168180305138));
#9029=CARTESIAN_POINT('Ctrl Pts',(-13.4333119308442,9.2035617400875,2.07463475387504));
#9030=CARTESIAN_POINT('Ctrl Pts',(-13.813333123997,8.70360226879533,2.0375877046987));
#9031=CARTESIAN_POINT('Ctrl Pts',(-14.3164162361929,8.4776951740808,2.00054065552236));
#9032=CARTESIAN_POINT('Ctrl Pts',(-14.8194993483888,8.25178807936627,1.96349360634602));
#9033=CARTESIAN_POINT('Ctrl Pts',(-15.4456443796278,8.2999333612294,1.92644655716968));
#9034=CARTESIAN_POINT('Ctrl Pts',(-15.9082771523615,8.60009592645602,1.88939950799334));
#9035=CARTESIAN_POINT('Ctrl Pts',(-16.3698223449295,8.8995528545734,1.85243955086549));
#9036=CARTESIAN_POINT('Ctrl Pts',(-16.668623160866,9.4498435492614,1.81547959373764));
#9037=CARTESIAN_POINT('Ctrl Pts',(-16.6687412413332,10.0000242582383,1.77851963660979));
#9038=CARTESIAN_POINT('Ctrl Pts',(-16.6658557594656,9.99847620480149,1.97148036339021));
#9039=CARTESIAN_POINT('Ctrl Pts',(-16.6670783192728,9.8644082985784,1.98044625340445));
#9040=CARTESIAN_POINT('Ctrl Pts',(-16.65225276481,9.73060740885205,1.98941214341869));
#9041=CARTESIAN_POINT('Ctrl Pts',(-16.6203420813068,9.60101349282022,1.99837803343293));
#9042=CARTESIAN_POINT('Ctrl Pts',(-16.4884871668348,9.06553155264917,2.03542508260927));
#9043=CARTESIAN_POINT('Ctrl Pts',(-16.0649307318521,8.60187702569495,2.07247213178561));
#9044=CARTESIAN_POINT('Ctrl Pts',(-15.5435261848766,8.42225541573886,2.10951918096195));
#9045=CARTESIAN_POINT('Ctrl Pts',(-15.0221216379011,8.24263380578278,2.14656623013829));
#9046=CARTESIAN_POINT('Ctrl Pts',(-14.4028689789328,8.34704511282482,2.18361327931463));
#9047=CARTESIAN_POINT('Ctrl Pts',(-13.9691879081116,8.68770234961182,2.22066032849097));
#9048=CARTESIAN_POINT('Ctrl Pts',(-13.5355068372904,9.02835958639883,2.25770737766731));
#9049=CARTESIAN_POINT('Ctrl Pts',(-13.2873973546162,9.60526275293079,2.29475442684365));
#9050=CARTESIAN_POINT('Ctrl Pts',(-13.3384142659838,10.154374671996,2.33180147601999));
#9051=CARTESIAN_POINT('Ctrl Pts',(-13.3894311773513,10.7034865910612,2.36884852519633));
#9052=CARTESIAN_POINT('Ctrl Pts',(-13.7395744827606,11.2248072626597,2.40589557437267));
#9053=CARTESIAN_POINT('Ctrl Pts',(-14.2285905127814,11.4797385218802,2.44294262354901));
#9054=CARTESIAN_POINT('Ctrl Pts',(-14.7176065428022,11.7346697811008,2.47998967272535));
#9055=CARTESIAN_POINT('Ctrl Pts',(-15.3454952974345,11.7232116279436,2.51703672190169));
#9056=CARTESIAN_POINT('Ctrl Pts',(-15.8248845058031,11.450608232057,2.55408377107803));
#9057=CARTESIAN_POINT('Ctrl Pts',(-16.3042737141718,11.1780048361704,2.59113082025437));
#9058=CARTESIAN_POINT('Ctrl Pts',(-16.6351633762768,10.6442561975546,2.62817786943071));
#9059=CARTESIAN_POINT('Ctrl Pts',(-16.66611183473,10.0936485172939,2.66522491860705));
#9060=CARTESIAN_POINT('Ctrl Pts',(-16.6678537312038,10.062658231359,2.6673100668681));
#9061=CARTESIAN_POINT('Ctrl Pts',(-16.6686454544998,10.0316145382597,2.66939521512915));
#9062=CARTESIAN_POINT('Ctrl Pts',(-16.6685089555354,10.000563745621,2.67148036339021));
#9063=CARTESIAN_POINT('Origin',(-15.,10.,4.));
#9064=CARTESIAN_POINT('',(-16.6641896231852,10.0011694308927,3.37148036339021));
#9065=CARTESIAN_POINT('',(-16.6637099363687,9.99914721740977,3.1785196366098));
#9066=CARTESIAN_POINT('',(-16.666,10.,4.));
#9067=CARTESIAN_POINT('Ctrl Pts',(-16.6637099363687,9.99914721740977,3.1785196366098));
#9068=CARTESIAN_POINT('Ctrl Pts',(-16.6621663356667,10.3320266710605,3.15633046801072));
#9069=CARTESIAN_POINT('Ctrl Pts',(-16.5654394528057,10.6657320996906,3.13414129941163));
#9070=CARTESIAN_POINT('Ctrl Pts',(-16.3796152224748,10.9388080800771,3.11195213081255));
#9071=CARTESIAN_POINT('Ctrl Pts',(-16.0693629762726,11.3947359004046,3.07490508163621));
#9072=CARTESIAN_POINT('Ctrl Pts',(-15.5107459794087,11.681655122571,3.03785803245988));
#9073=CARTESIAN_POINT('Ctrl Pts',(-14.959432188694,11.6682484904506,3.00081098328354));
#9074=CARTESIAN_POINT('Ctrl Pts',(-14.4081183979792,11.6548418583303,2.9637639341072));
#9075=CARTESIAN_POINT('Ctrl Pts',(-13.8641078134136,11.341109371923,2.92671688493086));
#9076=CARTESIAN_POINT('Ctrl Pts',(-13.5763833255364,10.8706401882922,2.88966983575452));
#9077=CARTESIAN_POINT('Ctrl Pts',(-13.2886588376591,10.4001710046614,2.85262278657818));
#9078=CARTESIAN_POINT('Ctrl Pts',(-13.2572204464702,9.77296512380708,2.81557573740183));
#9079=CARTESIAN_POINT('Ctrl Pts',(-13.4964568822746,9.27608227910361,2.77852868822549));
#9080=CARTESIAN_POINT('Ctrl Pts',(-13.7356933180791,8.77919943440014,2.74148163904915));
#9081=CARTESIAN_POINT('Ctrl Pts',(-14.2456045808769,8.41263962584757,2.70443458987282));
#9082=CARTESIAN_POINT('Ctrl Pts',(-14.7928143653133,8.34417003120825,2.66738754069648));
#9083=CARTESIAN_POINT('Ctrl Pts',(-15.3400241497496,8.27570043656892,2.63034049152014));
#9084=CARTESIAN_POINT('Ctrl Pts',(-15.9245324558244,8.50532105584284,2.5932934423438));
#9085=CARTESIAN_POINT('Ctrl Pts',(-16.278821386837,8.92793907166143,2.55624639316746));
#9086=CARTESIAN_POINT('Ctrl Pts',(-16.5265939724556,9.22349772264472,2.5303374743149));
#9087=CARTESIAN_POINT('Ctrl Pts',(-16.6617679015892,9.61345002555303,2.50442855546235));
#9088=CARTESIAN_POINT('Ctrl Pts',(-16.6649202598041,10.0014222546351,2.47851963660979));
#9089=CARTESIAN_POINT('Ctrl Pts',(-16.6685089555354,10.000563745621,2.67148036339021));
#9090=CARTESIAN_POINT('Ctrl Pts',(-16.6662202629958,9.4799318290084,2.70644226430549));
#9091=CARTESIAN_POINT('Ctrl Pts',(-16.4029750372034,8.95730397752036,2.74140416522078));
#9092=CARTESIAN_POINT('Ctrl Pts',(-15.982246261208,8.65096665241879,2.77636606613607));
#9093=CARTESIAN_POINT('Ctrl Pts',(-15.5364249744315,8.32635918971003,2.81341311531241));
#9094=CARTESIAN_POINT('Ctrl Pts',(-14.9137751460771,8.24461098619809,2.85046016448875));
#9095=CARTESIAN_POINT('Ctrl Pts',(-14.3992712940895,8.44313657871488,2.88750721366509));
#9096=CARTESIAN_POINT('Ctrl Pts',(-13.8847674421018,8.64166217123168,2.92455426284143));
#9097=CARTESIAN_POINT('Ctrl Pts',(-13.4784095664808,9.12046155977721,2.96160131201777));
#9098=CARTESIAN_POINT('Ctrl Pts',(-13.3661796340593,9.6603977290365,2.99864836119411));
#9099=CARTESIAN_POINT('Ctrl Pts',(-13.2539497016378,10.2003338982958,3.03569541037045));
#9100=CARTESIAN_POINT('Ctrl Pts',(-13.4358477124159,10.8014068482688,3.07274245954679));
#9101=CARTESIAN_POINT('Ctrl Pts',(-13.8286225426003,11.1885173717263,3.10978950872313));
#9102=CARTESIAN_POINT('Ctrl Pts',(-14.2213973727848,11.5756278951839,3.14683655789947));
#9103=CARTESIAN_POINT('Ctrl Pts',(-14.8250490223756,11.7487759921259,3.18388360707581));
#9104=CARTESIAN_POINT('Ctrl Pts',(-15.3632980642854,11.628715201347,3.22093065625215));
#9105=CARTESIAN_POINT('Ctrl Pts',(-15.9015471061952,11.5086544105681,3.25797770542849));
#9106=CARTESIAN_POINT('Ctrl Pts',(-16.374393540424,11.0953847320682,3.29502475460482));
#9107=CARTESIAN_POINT('Ctrl Pts',(-16.5654249012081,10.5780515282261,3.33207180378116));
#9108=CARTESIAN_POINT('Ctrl Pts',(-16.6331610271708,10.3946149086246,3.34520799031751));
#9109=CARTESIAN_POINT('Ctrl Pts',(-16.6654651595513,10.1980946093002,3.35834417685386));
#9110=CARTESIAN_POINT('Ctrl Pts',(-16.6641896231852,10.0011694308927,3.37148036339021));
#9111=CARTESIAN_POINT('Origin',(-15.,10.,4.));
#9112=CARTESIAN_POINT('',(-16.6642806308315,9.99878755139411,4.07148036339021));
#9113=CARTESIAN_POINT('',(-16.6680322603961,9.99903395438687,3.8785196366098));
#9114=CARTESIAN_POINT('',(-16.666,10.,4.));
#9115=CARTESIAN_POINT('Ctrl Pts',(-16.6680322603961,9.99903395438687,3.8785196366098));
#9116=CARTESIAN_POINT('Ctrl Pts',(-16.6646131543622,10.494401776487,3.84527942973542));
#9117=CARTESIAN_POINT('Ctrl Pts',(-16.4297940317408,10.9925842260247,3.81203922286105));
#9118=CARTESIAN_POINT('Ctrl Pts',(-16.043711877959,11.3020615534902,3.77879901598667));
#9119=CARTESIAN_POINT('Ctrl Pts',(-15.6134135771296,11.6469818427323,3.74175196681033));
#9120=CARTESIAN_POINT('Ctrl Pts',(-14.995221408434,11.7574989536148,3.70470491763399));
#9121=CARTESIAN_POINT('Ctrl Pts',(-14.4720697071203,11.5830313891797,3.66765786845765));
#9122=CARTESIAN_POINT('Ctrl Pts',(-13.9489180058066,11.4085638247447,3.63061081928131));
#9123=CARTESIAN_POINT('Ctrl Pts',(-13.5208067718749,10.9491115849921,3.59356377010497));
#9124=CARTESIAN_POINT('Ctrl Pts',(-13.3836740542319,10.4149568776457,3.55651672092864));
#9125=CARTESIAN_POINT('Ctrl Pts',(-13.2465413365889,9.88080217029943,3.5194696717523));
#9126=CARTESIAN_POINT('Ctrl Pts',(-13.4003871352347,9.27194499535936,3.48242262257596));
#9127=CARTESIAN_POINT('Ctrl Pts',(-13.7747992693407,8.86704724596919,3.44537557339962));
#9128=CARTESIAN_POINT('Ctrl Pts',(-14.1492114034467,8.46214949657901,3.40832852422328));
#9129=CARTESIAN_POINT('Ctrl Pts',(-14.744189873013,8.26121117273875,3.37128147504693));
#9130=CARTESIAN_POINT('Ctrl Pts',(-15.2874247939926,8.35619777313096,3.3342344258706));
#9131=CARTESIAN_POINT('Ctrl Pts',(-15.8306597149722,8.45118437352318,3.29718737669425));
#9132=CARTESIAN_POINT('Ctrl Pts',(-16.3221510873651,8.84209589814789,3.26014032751792));
#9133=CARTESIAN_POINT('Ctrl Pts',(-16.5369530257913,9.3500198697045,3.22309327834158));
#9134=CARTESIAN_POINT('Ctrl Pts',(-16.6231002796173,9.55372499277096,3.20823539776432));
#9135=CARTESIAN_POINT('Ctrl Pts',(-16.6647435323228,9.77625093597039,3.19337751718706));
#9136=CARTESIAN_POINT('Ctrl Pts',(-16.6637099363687,9.99914721740977,3.1785196366098));
#9137=CARTESIAN_POINT('Ctrl Pts',(-16.6641896231852,10.0011694308927,3.37148036339021));
#9138=CARTESIAN_POINT('Ctrl Pts',(-16.6618678553907,9.64272058592326,3.3953912260302));
#9139=CARTESIAN_POINT('Ctrl Pts',(-16.5482888473394,9.28293028253278,3.4193020886702));
#9140=CARTESIAN_POINT('Ctrl Pts',(-16.3346236739081,8.99826233990597,3.44321295131019));
#9141=CARTESIAN_POINT('Ctrl Pts',(-16.0035747984843,8.55720308461235,3.48026000048653));
#9142=CARTESIAN_POINT('Ctrl Pts',(-15.4322607602971,8.2964813032095,3.51730704966287));
#9143=CARTESIAN_POINT('Ctrl Pts',(-14.8821607009425,8.33542420112334,3.5543540988392));
#9144=CARTESIAN_POINT('Ctrl Pts',(-14.332060641588,8.37436709903719,3.59140114801554));
#9145=CARTESIAN_POINT('Ctrl Pts',(-13.8031745610662,8.71297467626774,3.62844819719189));
#9146=CARTESIAN_POINT('Ctrl Pts',(-13.5375631634618,9.19627293827846,3.66549524636823));
#9147=CARTESIAN_POINT('Ctrl Pts',(-13.2719517658575,9.67957120028917,3.70254229554457));
#9148=CARTESIAN_POINT('Ctrl Pts',(-13.2696150511706,10.30756014708,3.73958934472091));
#9149=CARTESIAN_POINT('Ctrl Pts',(-13.5316224875214,10.7928216517316,3.77663639389725));
#9150=CARTESIAN_POINT('Ctrl Pts',(-13.7936299238721,11.2780831563831,3.81368344307358));
#9151=CARTESIAN_POINT('Ctrl Pts',(-14.3199815112606,11.6206172188953,3.85073049224993));
#9152=CARTESIAN_POINT('Ctrl Pts',(-14.8697765330075,11.6636527700371,3.88777754142627));
#9153=CARTESIAN_POINT('Ctrl Pts',(-15.4195715547545,11.7066883211789,3.92482459060261));
#9154=CARTESIAN_POINT('Ctrl Pts',(-15.99281001086,11.4502253609502,3.96187163977895));
#9155=CARTESIAN_POINT('Ctrl Pts',(-16.3271319916882,11.0116419165125,3.99891868895529));
#9156=CARTESIAN_POINT('Ctrl Pts',(-16.5454036513628,10.7253001806623,4.02310591376693));
#9157=CARTESIAN_POINT('Ctrl Pts',(-16.6618370586765,10.3613295085513,4.04729313857857));
#9158=CARTESIAN_POINT('Ctrl Pts',(-16.6642806308315,9.99878755139411,4.07148036339021));
#9159=CARTESIAN_POINT('Origin',(-15.,10.,4.));
#9160=CARTESIAN_POINT('',(-16.6685641298519,9.99950756874516,4.77148036339021));
#9161=CARTESIAN_POINT('',(-16.66663599516,10.0014616028905,4.5785196366098));
#9162=CARTESIAN_POINT('',(-16.666,10.,4.));
#9163=CARTESIAN_POINT('Ctrl Pts',(-16.66663599516,10.0014616028905,4.5785196366098));
#9164=CARTESIAN_POINT('Ctrl Pts',(-16.6676283665625,10.1096548573022,4.57127544063647));
#9165=CARTESIAN_POINT('Ctrl Pts',(-16.6579946337124,10.2176721666637,4.56403124466314));
#9166=CARTESIAN_POINT('Ctrl Pts',(-16.6370920864311,10.323462940401,4.55678704868981));
#9167=CARTESIAN_POINT('Ctrl Pts',(-16.5301957931928,10.8644803302501,4.51973999951347));
#9168=CARTESIAN_POINT('Ctrl Pts',(-16.1285825664142,11.3472664167428,4.48269295033713));
#9169=CARTESIAN_POINT('Ctrl Pts',(-15.6160628409387,11.5508595517598,4.44564590116079));
#9170=CARTESIAN_POINT('Ctrl Pts',(-15.1035431154632,11.7544526867768,4.40859885198445));
#9171=CARTESIAN_POINT('Ctrl Pts',(-14.4801168912907,11.6788528703182,4.37155180280811));
#9172=CARTESIAN_POINT('Ctrl Pts',(-14.0311140273948,11.3586606439277,4.33450475363177));
#9173=CARTESIAN_POINT('Ctrl Pts',(-13.5821111634988,11.0384684175371,4.29745770445543));
#9174=CARTESIAN_POINT('Ctrl Pts',(-13.3075316598793,10.4736837812147,4.26041065527909));
#9175=CARTESIAN_POINT('Ctrl Pts',(-13.3330451274809,9.92279749839539,4.22336360610275));
#9176=CARTESIAN_POINT('Ctrl Pts',(-13.3585585950825,9.37191121557606,4.18631655692641));
#9177=CARTESIAN_POINT('Ctrl Pts',(-13.6841650339053,8.83492328625981,4.14926950775007));
#9178=CARTESIAN_POINT('Ctrl Pts',(-14.1608408134576,8.55760247056822,4.11222245857373));
#9179=CARTESIAN_POINT('Ctrl Pts',(-14.6375165930098,8.28028165487663,4.07517540939739));
#9180=CARTESIAN_POINT('Ctrl Pts',(-15.2652617132915,8.2626279528097,4.03812836022105));
#9181=CARTESIAN_POINT('Ctrl Pts',(-15.756769641956,8.51272111482649,4.00108131104471));
#9182=CARTESIAN_POINT('Ctrl Pts',(-16.2482775706204,8.76281427684328,3.96403426186837));
#9183=CARTESIAN_POINT('Ctrl Pts',(-16.6035483076676,9.28065430294379,3.92698721269203));
#9184=CARTESIAN_POINT('Ctrl Pts',(-16.6599814597096,9.82923604979498,3.88994016351569));
#9185=CARTESIAN_POINT('Ctrl Pts',(-16.6657803590876,9.88560664465826,3.88613332121373));
#9186=CARTESIAN_POINT('Ctrl Pts',(-16.6684238342973,9.94230184115634,3.88232647891176));
#9187=CARTESIAN_POINT('Ctrl Pts',(-16.6680322603961,9.99903395438687,3.8785196366098));
#9188=CARTESIAN_POINT('Ctrl Pts',(-16.6642806308315,9.99878755139411,4.07148036339021));
#9189=CARTESIAN_POINT('Ctrl Pts',(-16.6655798253021,9.80603183302699,4.08434018775491));
#9190=CARTESIAN_POINT('Ctrl Pts',(-16.6346561573177,9.61367998650847,4.09720001211961));
#9191=CARTESIAN_POINT('Ctrl Pts',(-16.5696832944175,9.43361404869653,4.11005983648431));
#9192=CARTESIAN_POINT('Ctrl Pts',(-16.3825071107676,8.91487355396514,4.14710688566065));
#9193=CARTESIAN_POINT('Ctrl Pts',(-15.9127492379168,8.49809649314917,4.18415393483699));
#9194=CARTESIAN_POINT('Ctrl Pts',(-15.3754085681396,8.37403348817524,4.22120098401333));
#9195=CARTESIAN_POINT('Ctrl Pts',(-14.8380678983624,8.24997048320131,4.25824803318967));
#9196=CARTESIAN_POINT('Ctrl Pts',(-14.2331444316588,8.41862153406943,4.295295082366));
#9197=CARTESIAN_POINT('Ctrl Pts',(-13.837499680669,8.80279838867386,4.33234213154234));
#9198=CARTESIAN_POINT('Ctrl Pts',(-13.4418549296792,9.18697524327829,4.36938918071868));
#9199=CARTESIAN_POINT('Ctrl Pts',(-13.2554888944033,9.78667790161905,4.40643622989502));
#9200=CARTESIAN_POINT('Ctrl Pts',(-13.3636976251207,10.3274343118419,4.44348327907136));
#9201=CARTESIAN_POINT('Ctrl Pts',(-13.4719063558382,10.8681907220648,4.4805303282477));
#9202=CARTESIAN_POINT('Ctrl Pts',(-13.874689852549,11.3500008841698,4.51757737742404));
#9203=CARTESIAN_POINT('Ctrl Pts',(-14.3877020709949,11.5523498113339,4.55462442660038));
#9204=CARTESIAN_POINT('Ctrl Pts',(-14.9007142894408,11.754698738498,4.59167147577672));
#9205=CARTESIAN_POINT('Ctrl Pts',(-15.5239552296219,11.6775864307212,4.62871852495307));
#9206=CARTESIAN_POINT('Ctrl Pts',(-15.9721798333851,11.3563056669346,4.6657655741294));
#9207=CARTESIAN_POINT('Ctrl Pts',(-16.3985203074742,11.050711123488,4.70100383721634));
#9208=CARTESIAN_POINT('Ctrl Pts',(-16.666517248032,10.5242086528571,4.73624210030327));
#9209=CARTESIAN_POINT('Ctrl Pts',(-16.6685641298519,9.99950756874516,4.77148036339021));
#9210=CARTESIAN_POINT('Origin',(-15.,10.,4.));
#9211=CARTESIAN_POINT('',(-16.665731796286,10.0015218067206,5.47148036339021));
#9212=CARTESIAN_POINT('',(-16.6632774972289,10.0000562476522,5.2785196366098));
#9213=CARTESIAN_POINT('',(-16.666,10.,4.));
#9214=CARTESIAN_POINT('Ctrl Pts',(-16.6632774972289,10.0000562476522,5.2785196366098));
#9215=CARTESIAN_POINT('Ctrl Pts',(-16.6633601998516,10.2746976550433,5.26022440236118));
#9216=CARTESIAN_POINT('Ctrl Pts',(-16.5991042841727,10.5493026373111,5.24192916811255));
#9217=CARTESIAN_POINT('Ctrl Pts',(-16.4702969568271,10.7892563791,5.22363393386393));
#9218=CARTESIAN_POINT('Ctrl Pts',(-16.2094677525875,11.2751522113859,5.1865868846876));
#9219=CARTESIAN_POINT('Ctrl Pts',(-15.6839488500416,11.6189624385472,5.14953983551125));
#9220=CARTESIAN_POINT('Ctrl Pts',(-15.1342598624345,11.663331915957,5.11249278633491));
#9221=CARTESIAN_POINT('Ctrl Pts',(-14.5845708748275,11.7077013933668,5.07544573715857));
#9222=CARTESIAN_POINT('Ctrl Pts',(-14.0107118021594,11.4526301210251,5.03839868798223));
#9223=CARTESIAN_POINT('Ctrl Pts',(-13.67532659802,11.0148591780905,5.00135163880589));
#9224=CARTESIAN_POINT('Ctrl Pts',(-13.3399413938806,10.5770882351559,4.96430458962955));
#9225=CARTESIAN_POINT('Ctrl Pts',(-13.2430300582699,9.95661762162842,4.92725754045321));
#9226=CARTESIAN_POINT('Ctrl Pts',(-13.4289469937516,9.43742447189813,4.89021049127687));
#9227=CARTESIAN_POINT('Ctrl Pts',(-13.6148639292333,8.91823132216784,4.85316344210053));
#9228=CARTESIAN_POINT('Ctrl Pts',(-14.0836091358075,8.50031563623478,4.81611639292419));
#9229=CARTESIAN_POINT('Ctrl Pts',(-14.6206471985419,8.37494916224136,4.77906934374785));
#9230=CARTESIAN_POINT('Ctrl Pts',(-15.1576852612763,8.24958268824794,4.74202229457151));
#9231=CARTESIAN_POINT('Ctrl Pts',(-15.7630161801709,8.41676542619417,4.70497524539517));
#9232=CARTESIAN_POINT('Ctrl Pts',(-16.1595919597692,8.79998114177013,4.66792819621883));
#9233=CARTESIAN_POINT('Ctrl Pts',(-16.4786211403925,9.10826269105184,4.63812534301582));
#9234=CARTESIAN_POINT('Ctrl Pts',(-16.6625533475701,9.55635110468484,4.60832248981281));
#9235=CARTESIAN_POINT('Ctrl Pts',(-16.66663599516,10.0014616028905,4.5785196366098));
#9236=CARTESIAN_POINT('Ctrl Pts',(-16.6685641298519,9.99950756874516,4.77148036339021));
#9237=CARTESIAN_POINT('Ctrl Pts',(-16.6686691966469,9.9725745720848,4.77328914947961));
#9238=CARTESIAN_POINT('Ctrl Pts',(-16.6680735418144,9.94564632169335,4.77509793556902));
#9239=CARTESIAN_POINT('Ctrl Pts',(-16.6667626122128,9.91875293767893,4.77690672165842));
#9240=CARTESIAN_POINT('Ctrl Pts',(-16.639912519932,9.36793019200639,4.81395377083476));
#9241=CARTESIAN_POINT('Ctrl Pts',(-16.313004068025,8.83173392045779,4.8510008200111));
#9242=CARTESIAN_POINT('Ctrl Pts',(-15.8356567926335,8.55557055708282,4.88804786918744));
#9243=CARTESIAN_POINT('Ctrl Pts',(-15.358309517242,8.27940719370785,4.92509491836379));
#9244=CARTESIAN_POINT('Ctrl Pts',(-14.7305234183659,8.2632767385065,4.96214196754013));
#9245=CARTESIAN_POINT('Ctrl Pts',(-14.239623783446,8.51456178188315,4.99918901671647));
#9246=CARTESIAN_POINT('Ctrl Pts',(-13.7487241485261,8.76584682525981,5.03623606589281));
#9247=CARTESIAN_POINT('Ctrl Pts',(-13.3947109775624,9.28454736721446,5.07328311506914));
#9248=CARTESIAN_POINT('Ctrl Pts',(-13.339609100803,9.83326442346505,5.11033016424548));
#9249=CARTESIAN_POINT('Ctrl Pts',(-13.2845072240436,10.3819814797156,5.14737721342182));
#9250=CARTESIAN_POINT('Ctrl Pts',(-13.5283166414883,10.9607150502622,5.18442426259816));
#9251=CARTESIAN_POINT('Ctrl Pts',(-13.9594506023805,11.3045902199309,5.2214713117745));
#9252=CARTESIAN_POINT('Ctrl Pts',(-14.3905845632726,11.6484653895996,5.25851836095084));
#9253=CARTESIAN_POINT('Ctrl Pts',(-15.009043067612,11.7574821583904,5.29556541012718));
#9254=CARTESIAN_POINT('Ctrl Pts',(-15.5317698835803,11.5817457068139,5.33261245930352));
#9255=CARTESIAN_POINT('Ctrl Pts',(-16.0544966995486,11.4060092552373,5.36965950847986));
#9256=CARTESIAN_POINT('Ctrl Pts',(-16.4814918271458,10.9455195832933,5.4067065576562));
#9257=CARTESIAN_POINT('Ctrl Pts',(-16.6173280372926,10.411033709843,5.44375360683254));
#9258=CARTESIAN_POINT('Ctrl Pts',(-16.6512155543302,10.2776937180744,5.45299585901843));
#9259=CARTESIAN_POINT('Ctrl Pts',(-16.6669822248687,10.1397484275201,5.46223811120432));
#9260=CARTESIAN_POINT('Ctrl Pts',(-16.665731796286,10.0015218067206,5.47148036339021));
#9261=CARTESIAN_POINT('Origin',(-15.,10.,4.));
#9262=CARTESIAN_POINT('',(-16.6633786660592,9.9995695770803,6.17148036339021));
#9263=CARTESIAN_POINT('',(-16.6664295062294,9.99850933107572,5.9785196366098));
#9264=CARTESIAN_POINT('',(-16.666,10.,4.));
#9265=CARTESIAN_POINT('Ctrl Pts',(-16.6664295062294,9.99850933107572,5.9785196366098));
#9266=CARTESIAN_POINT('Ctrl Pts',(-16.6623835386158,10.4369404484093,5.94917336408588));
#9267=CARTESIAN_POINT('Ctrl Pts',(-16.4846437176932,10.8782736700321,5.91982709156197));
#9268=CARTESIAN_POINT('Ctrl Pts',(-16.1742579084843,11.1856715961173,5.89048081903805));
#9269=CARTESIAN_POINT('Ctrl Pts',(-15.7824235340154,11.5737340348854,5.85343376986171));
#9270=CARTESIAN_POINT('Ctrl Pts',(-15.1791937896595,11.7483463595048,5.81638672068537));
#9271=CARTESIAN_POINT('Ctrl Pts',(-14.6406550026031,11.6295919573634,5.77933967150903));
#9272=CARTESIAN_POINT('Ctrl Pts',(-14.1021162155467,11.5108375552221,5.74229262233269));
#9273=CARTESIAN_POINT('Ctrl Pts',(-13.6282683857898,11.09871642632,5.70524557315635));
#9274=CARTESIAN_POINT('Ctrl Pts',(-13.4359822991767,10.5818482663145,5.66819852398002));
#9275=CARTESIAN_POINT('Ctrl Pts',(-13.2436962125636,10.064980106309,5.63115147480367));
#9276=CARTESIAN_POINT('Ctrl Pts',(-13.3329718690941,9.44336491520019,5.59410442562733));
#9277=CARTESIAN_POINT('Ctrl Pts',(-13.662949564977,9.00150367703514,5.55705737645099));
#9278=CARTESIAN_POINT('Ctrl Pts',(-13.9929272608599,8.55964243887008,5.52001032727465));
#9279=CARTESIAN_POINT('Ctrl Pts',(-14.5636069960951,8.29753515364879,5.48296327809831));
#9280=CARTESIAN_POINT('Ctrl Pts',(-15.1137999373131,8.33514314496572,5.44591622892197));
#9281=CARTESIAN_POINT('Ctrl Pts',(-15.6639928785312,8.37275113628264,5.40886917974563));
#9282=CARTESIAN_POINT('Ctrl Pts',(-16.193699025732,8.71007440413778,5.37182213056929));
#9283=CARTESIAN_POINT('Ctrl Pts',(-16.4604823463659,9.19272675677063,5.33477508139295));
#9284=CARTESIAN_POINT('Ctrl Pts',(-16.5955179717545,9.43702712055721,5.31602326646523));
#9285=CARTESIAN_POINT('Ctrl Pts',(-16.6631927306577,9.71856081704436,5.29727145153751));
#9286=CARTESIAN_POINT('Ctrl Pts',(-16.6632774972289,10.0000562476522,5.2785196366098));
#9287=CARTESIAN_POINT('Ctrl Pts',(-16.665731796286,10.0015218067206,5.47148036339021));
#9288=CARTESIAN_POINT('Ctrl Pts',(-16.6619699520738,9.58567477585555,5.49928516038066));
#9289=CARTESIAN_POINT('Ctrl Pts',(-16.504190860803,9.16728149961843,5.52708995737111));
#9290=CARTESIAN_POINT('Ctrl Pts',(-16.2224480480665,8.86407770434065,5.55489475436156));
#9291=CARTESIAN_POINT('Ctrl Pts',(-15.847054555997,8.46008964724508,5.5919418035379));
#9292=CARTESIAN_POINT('Ctrl Pts',(-15.2515902791614,8.26059560801048,5.62898885271424));
#9293=CARTESIAN_POINT('Ctrl Pts',(-14.7085874460709,8.3569000607923,5.66603590189058));
#9294=CARTESIAN_POINT('Ctrl Pts',(-14.1655846129804,8.45320451357413,5.70308295106692));
#9295=CARTESIAN_POINT('Ctrl Pts',(-13.6750432236349,8.84530745837239,5.74013000024326));
#9296=CARTESIAN_POINT('Ctrl Pts',(-13.461474374797,9.35375113620292,5.7771770494196));
#9297=CARTESIAN_POINT('Ctrl Pts',(-13.2479055259592,9.86219481403344,5.81422409859594));
#9298=CARTESIAN_POINT('Ctrl Pts',(-13.3113092176289,10.4869792248962,5.85127114777228));
#9299=CARTESIAN_POINT('Ctrl Pts',(-13.6226668338069,10.9421528795107,5.88831819694862));
#9300=CARTESIAN_POINT('Ctrl Pts',(-13.9340244499849,11.3973265341252,5.92536524612496));
#9301=CARTESIAN_POINT('Ctrl Pts',(-14.4933359906712,11.6828894324913,5.9624122953013));
#9302=CARTESIAN_POINT('Ctrl Pts',(-15.0446156194918,11.6681451102855,5.99945934447764));
#9303=CARTESIAN_POINT('Ctrl Pts',(-15.5958952483124,11.6534007880796,6.03650639365398));
#9304=CARTESIAN_POINT('Ctrl Pts',(-16.1391429652673,11.3383492453018,6.07355344283032));
#9305=CARTESIAN_POINT('Ctrl Pts',(-16.4257250303767,10.8671832884336,6.11060049200666));
#9306=CARTESIAN_POINT('Ctrl Pts',(-16.5827063073618,10.6090923518887,6.13089378246784));
#9307=CARTESIAN_POINT('Ctrl Pts',(-16.6626743340805,10.304158846593,6.15118707292903));
#9308=CARTESIAN_POINT('Ctrl Pts',(-16.6633786660592,9.9995695770803,6.17148036339021));
#9309=CARTESIAN_POINT('Origin',(-15.,10.,4.));
#9310=CARTESIAN_POINT('',(-16.6673099161007,9.99870037981829,6.87148036339021));
#9311=CARTESIAN_POINT('',(-16.6681787596498,10.0008675363463,6.67851963660979));
#9312=CARTESIAN_POINT('',(-16.666,10.,4.));
#9313=CARTESIAN_POINT('Ctrl Pts',(-16.6681787596498,10.0008675363463,6.67851963660979));
#9314=CARTESIAN_POINT('Ctrl Pts',(-16.6684948606872,10.0507838420897,6.67516937498693));
#9315=CARTESIAN_POINT('Ctrl Pts',(-16.6664485977206,10.1006738719505,6.67181911336406));
#9316=CARTESIAN_POINT('Ctrl Pts',(-16.6619555158093,10.1503425574736,6.66846885174119));
#9317=CARTESIAN_POINT('Ctrl Pts',(-16.6122712089522,10.6995767493754,6.63142180256485));
#9318=CARTESIAN_POINT('Ctrl Pts',(-16.2633937611776,11.2217453066089,6.59437475338851));
#9319=CARTESIAN_POINT('Ctrl Pts',(-15.7749977113418,11.4778623470653,6.55732770421217));
#9320=CARTESIAN_POINT('Ctrl Pts',(-15.286601661506,11.7339793875217,6.52028065503583));
#9321=CARTESIAN_POINT('Ctrl Pts',(-14.658687009609,11.724044911201,6.48323360585949));
#9322=CARTESIAN_POINT('Ctrl Pts',(-14.178637761833,11.4526055538444,6.44618655668315));
#9323=CARTESIAN_POINT('Ctrl Pts',(-13.6985885140571,11.1811661964878,6.40913950750681));
#9324=CARTESIAN_POINT('Ctrl Pts',(-13.3664046704023,10.6482219580952,6.37209245833047));
#9325=CARTESIAN_POINT('Ctrl Pts',(-13.3341202701254,10.0976909730731,6.33504540915413));
#9326=CARTESIAN_POINT('Ctrl Pts',(-13.3018358698486,9.54715998805105,6.29799835997779));
#9327=CARTESIAN_POINT('Ctrl Pts',(-13.5694509129499,8.97904225639946,6.26095131080145));
#9328=CARTESIAN_POINT('Ctrl Pts',(-14.0144832531239,8.65335398608828,6.22390426162511));
#9329=CARTESIAN_POINT('Ctrl Pts',(-14.459515593298,8.3276657157771,6.18685721244877));
#9330=CARTESIAN_POINT('Ctrl Pts',(-15.0819652305448,8.24440690680633,6.14981016327243));
#9331=CARTESIAN_POINT('Ctrl Pts',(-15.5969492865558,8.44168349460096,6.11276311409609));
#9332=CARTESIAN_POINT('Ctrl Pts',(-16.1119333425668,8.63896008239559,6.07571606491975));
#9333=CARTESIAN_POINT('Ctrl Pts',(-16.5194518173418,9.11677206695562,6.03866901574341));
#9334=CARTESIAN_POINT('Ctrl Pts',(-16.6329915524384,9.65643433569403,6.00162196656707));
#9335=CARTESIAN_POINT('Ctrl Pts',(-16.6565924642679,9.76861111337784,5.99392118991465));
#9336=CARTESIAN_POINT('Ctrl Pts',(-16.6674912115247,9.8834603036632,5.98622041326222));
#9337=CARTESIAN_POINT('Ctrl Pts',(-16.6664295062294,9.99850933107572,5.9785196366098));
#9338=CARTESIAN_POINT('Ctrl Pts',(-16.6633786660592,9.9995695770803,6.17148036339021));
#9339=CARTESIAN_POINT('Ctrl Pts',(-16.6639601492863,9.7481064080884,6.18823412210537));
#9340=CARTESIAN_POINT('Ctrl Pts',(-16.6105167436314,9.49687786479725,6.20498788082053));
#9341=CARTESIAN_POINT('Ctrl Pts',(-16.5017821168752,9.27243611128139,6.22174163953568));
#9342=CARTESIAN_POINT('Ctrl Pts',(-16.2613407250004,8.77613526195597,6.25878868871202));
#9343=CARTESIAN_POINT('Ctrl Pts',(-15.7505415279869,8.41081393426368,6.29583573788836));
#9344=CARTESIAN_POINT('Ctrl Pts',(-15.2031672253873,8.34367226516766,6.3328827870647));
#9345=CARTESIAN_POINT('Ctrl Pts',(-14.6557929227877,8.27653059607164,6.36992983624104));
#9346=CARTESIAN_POINT('Ctrl Pts',(-14.0718435146019,8.50756858557189,6.40697688541738));
#9347=CARTESIAN_POINT('Ctrl Pts',(-13.7185810927601,8.93104512595157,6.44402393459372));
#9348=CARTESIAN_POINT('Ctrl Pts',(-13.3653186709184,9.35452166633125,6.48107098377006));
#9349=CARTESIAN_POINT('Ctrl Pts',(-13.2427432354206,9.97043675759037,6.5181180329464));
#9350=CARTESIAN_POINT('Ctrl Pts',(-13.4069551569713,10.4968974375652,6.55516508212274));
#9351=CARTESIAN_POINT('Ctrl Pts',(-13.571167078522,11.0233581175401,6.59221213129908));
#9352=CARTESIAN_POINT('Ctrl Pts',(-14.0221663571212,11.4603643862307,6.62925918047542));
#9353=CARTESIAN_POINT('Ctrl Pts',(-14.553539505443,11.6079086639697,6.66630622965176));
#9354=CARTESIAN_POINT('Ctrl Pts',(-15.0849126537649,11.7554529417086,6.7033532788281));
#9355=CARTESIAN_POINT('Ctrl Pts',(-15.6966596718095,11.6135352284959,6.74040032800444));
#9356=CARTESIAN_POINT('Ctrl Pts',(-16.1087961059817,11.247105450898,6.77744737718078));
#9357=CARTESIAN_POINT('Ctrl Pts',(-16.4574916205823,10.9370808831329,6.80879170591726));
#9358=CARTESIAN_POINT('Ctrl Pts',(-16.6632996251162,10.4663435453455,6.84013603465373));
#9359=CARTESIAN_POINT('Ctrl Pts',(-16.6673099161007,9.99870037981829,6.87148036339021));
#9360=CARTESIAN_POINT('Origin',(-15.,10.,4.));
#9361=CARTESIAN_POINT('',(-16.6674569633666,10.0012065537184,7.57148036339021));
#9362=CARTESIAN_POINT('',(-16.6638185641669,10.0009395545784,7.3785196366098));
#9363=CARTESIAN_POINT('',(-16.666,10.,4.));
#9364=CARTESIAN_POINT('',(-13.7309291201476,11.0793586530485,8.));
#9365=CARTESIAN_POINT('Ctrl Pts',(-16.6674569633666,10.0012065537184,7.57148036339021));
#9366=CARTESIAN_POINT('Ctrl Pts',(-16.6635088351118,9.52850380962102,7.60317909473112));
#9367=CARTESIAN_POINT('Ctrl Pts',(-16.4524516198717,9.05282917058819,7.63487782607203));
#9368=CARTESIAN_POINT('Ctrl Pts',(-16.0968413167821,8.74254092877981,7.66657655741294));
#9369=CARTESIAN_POINT('Ctrl Pts',(-15.6812312330697,8.37989979877725,7.70362360658928));
#9370=CARTESIAN_POINT('Ctrl Pts',(-15.0681740060149,8.24316232925988,7.74067065576562));
#9371=CARTESIAN_POINT('Ctrl Pts',(-14.5382155648778,8.39611193633351,7.77771770494196));
#9372=CARTESIAN_POINT('Ctrl Pts',(-14.0082571237407,8.54906154340714,7.8147647541183));
#9373=CARTESIAN_POINT('Ctrl Pts',(-13.5613974685214,8.99169822707177,7.85181180329464));
#9374=CARTESIAN_POINT('Ctrl Pts',(-13.4023347302998,9.51877034776798,7.88885885247098));
#9375=CARTESIAN_POINT('Ctrl Pts',(-13.2432719920782,10.0458424684642,7.92590590164732));
#9376=CARTESIAN_POINT('Ctrl Pts',(-13.3720061708544,10.657350026192,7.96295295082366));
#9377=CARTESIAN_POINT('Ctrl Pts',(-13.7309291201476,11.0793586530485,8.));
#9378=CARTESIAN_POINT('',(-16.2714529275337,11.0812362047421,8.));
#9379=CARTESIAN_POINT('Origin',(-15.,10.,8.));
#9380=CARTESIAN_POINT('Ctrl Pts',(-16.271453753893,11.081236856086,8.));
#9381=CARTESIAN_POINT('Ctrl Pts',(-15.920559526648,11.4928281424795,7.96367382485347));
#9382=CARTESIAN_POINT('Ctrl Pts',(-15.3505267893051,11.7187789801255,7.92734764970694));
#9383=CARTESIAN_POINT('Ctrl Pts',(-14.8130932173799,11.6581104500235,7.89102147456041));
#9384=CARTESIAN_POINT('Ctrl Pts',(-14.2649945560753,11.5962379845332,7.85397442538407));
#9385=CARTESIAN_POINT('Ctrl Pts',(-13.7508017247742,11.2362576554198,7.81692737620773));
#9386=CARTESIAN_POINT('Ctrl Pts',(-13.5055196558539,10.7424222226956,7.77988032703139));
#9387=CARTESIAN_POINT('Ctrl Pts',(-13.2602375869336,10.2485867899714,7.74283327785505));
#9388=CARTESIAN_POINT('Ctrl Pts',(-13.2838662803941,9.62089625363646,7.70578622867871));
#9389=CARTESIAN_POINT('Ctrl Pts',(-13.5657615787267,9.14688997129425,7.66873917950237));
#9390=CARTESIAN_POINT('Ctrl Pts',(-13.8476568770592,8.67288368895204,7.63169213032603));
#9391=CARTESIAN_POINT('Ctrl Pts',(-14.3878187802639,8.35256166060256,7.59464508114969));
#9392=CARTESIAN_POINT('Ctrl Pts',(-14.9389380812345,8.3323961008681,7.55759803197335));
#9393=CARTESIAN_POINT('Ctrl Pts',(-15.490057382205,8.31223054113365,7.52055098279701));
#9394=CARTESIAN_POINT('Ctrl Pts',(-16.0521340809416,8.59222145001422,7.48350393362067));
#9395=CARTESIAN_POINT('Ctrl Pts',(-16.3679620729449,9.04429105270523,7.44645688444433));
#9396=CARTESIAN_POINT('Ctrl Pts',(-16.5610182455944,9.32062763298445,7.42381113516615));
#9397=CARTESIAN_POINT('Ctrl Pts',(-16.6620633433819,9.66126158882507,7.40116538588798));
#9398=CARTESIAN_POINT('Ctrl Pts',(-16.6638185641669,10.0009395545784,7.3785196366098));
#9399=CARTESIAN_POINT('Origin',(-15.,-10.,4.));
#9400=CARTESIAN_POINT('',(-16.6671910371619,-9.99865073764983,0.571480363390209));
#9401=CARTESIAN_POINT('',(-16.6635932794994,-9.99933537909448,0.378519636609792));
#9402=CARTESIAN_POINT('',(-16.666,-10.,4.));
#9403=CARTESIAN_POINT('',(-13.3882904778579,-10.4218393251423,0.));
#9404=CARTESIAN_POINT('Ctrl Pts',(-16.6635932794994,-9.99933537909448,0.378519636609792));
#9405=CARTESIAN_POINT('Ctrl Pts',(-16.6645714516563,-9.77385592384011,0.363487571935548));
#9406=CARTESIAN_POINT('Ctrl Pts',(-16.6219039270364,-9.54871059169984,0.348455507261303));
#9407=CARTESIAN_POINT('Ctrl Pts',(-16.5338111352405,-9.34297002313031,0.333423442587059));
#9408=CARTESIAN_POINT('Ctrl Pts',(-16.3167033685785,-8.83591519556408,0.29637639341072));
#9409=CARTESIAN_POINT('Ctrl Pts',(-15.8236855882005,-8.44672359513559,0.25932934423438));
#9410=CARTESIAN_POINT('Ctrl Pts',(-15.2798473371766,-8.35458603397586,0.222282295058041));
#9411=CARTESIAN_POINT('Ctrl Pts',(-14.7360090861527,-8.26244847281612,0.185235245881701));
#9412=CARTESIAN_POINT('Ctrl Pts',(-14.1413503644829,-8.46736495092516,0.14818819670536));
#9413=CARTESIAN_POINT('Ctrl Pts',(-13.7693517818271,-8.87322579748708,0.111141147529019));
#9414=CARTESIAN_POINT('Ctrl Pts',(-13.3973531991712,-9.279086644049,0.0740940983526794));
#9415=CARTESIAN_POINT('Ctrl Pts',(-13.2480147555294,-9.88589185906381,0.0370470491763398));
#9416=CARTESIAN_POINT('Ctrl Pts',(-13.3882904778579,-10.4218393251423,-1.04083408558608E-16));
#9417=CARTESIAN_POINT('',(-15.675077185675,-11.5230977622533,0.));
#9418=CARTESIAN_POINT('Origin',(-15.,-10.,0.));
#9419=CARTESIAN_POINT('Ctrl Pts',(-15.6764092460936,-11.5258237909713,6.93889390390723E-17));
#9420=CARTESIAN_POINT('Ctrl Pts',(-15.1816817456953,-11.7444073771468,0.03632617514653));
#9421=CARTESIAN_POINT('Ctrl Pts',(-14.5700634637383,-11.7006543009145,0.0726523502930598));
#9422=CARTESIAN_POINT('Ctrl Pts',(-14.112175591995,-11.4128101852352,0.10897852543959));
#9423=CARTESIAN_POINT('Ctrl Pts',(-13.6452011738709,-11.119253952968,0.14602557461593));
#9424=CARTESIAN_POINT('Ctrl Pts',(-13.3381191053909,-10.5718228382361,0.183072623792269));
#9425=CARTESIAN_POINT('Ctrl Pts',(-13.3313947771057,-10.0204685483491,0.220119672968609));
#9426=CARTESIAN_POINT('Ctrl Pts',(-13.3246704488204,-9.46911425846216,0.257166722144949));
#9427=CARTESIAN_POINT('Ctrl Pts',(-13.6183038607298,-8.91383679342002,0.294213771321291));
#9428=CARTESIAN_POINT('Ctrl Pts',(-14.0779463710605,-8.6090816828823,0.331260820497631));
#9429=CARTESIAN_POINT('Ctrl Pts',(-14.5375888813912,-8.30432657234457,0.368307869673971));
#9430=CARTESIAN_POINT('Ctrl Pts',(-15.1632404901431,-8.25009381631124,0.405354918850311));
#9431=CARTESIAN_POINT('Ctrl Pts',(-15.6685313483052,-8.47104697428163,0.442401968026651));
#9432=CARTESIAN_POINT('Ctrl Pts',(-16.1738222064672,-8.69200013225201,0.47944901720299));
#9433=CARTESIAN_POINT('Ctrl Pts',(-16.5587523140395,-9.18813920422607,0.516496066379328));
#9434=CARTESIAN_POINT('Ctrl Pts',(-16.6471578533932,-9.73247249241234,0.553543115555668));
#9435=CARTESIAN_POINT('Ctrl Pts',(-16.6614257650046,-9.82032331374959,0.559522198167181));
#9436=CARTESIAN_POINT('Ctrl Pts',(-16.6679700273063,-9.90942946184446,0.565501280778695));
#9437=CARTESIAN_POINT('Ctrl Pts',(-16.6671910371619,-9.99865073764983,0.571480363390209));
#9438=CARTESIAN_POINT('Origin',(-15.,-10.,4.));
#9439=CARTESIAN_POINT('',(-16.6633491819668,-9.99963522328558,1.27148036339021));
#9440=CARTESIAN_POINT('',(-16.6649907850313,-10.0014379678122,1.07851963660979));
#9441=CARTESIAN_POINT('',(-16.666,-10.,4.));
#9442=CARTESIAN_POINT('Ctrl Pts',(-16.6649907850313,-10.0014379678122,1.07851963660979));
#9443=CARTESIAN_POINT('Ctrl Pts',(-16.6617723741096,-9.61090137508408,1.05243653366026));
#9444=CARTESIAN_POINT('Ctrl Pts',(-16.5246077727235,-9.21832985646356,1.02635343071072));
#9445=CARTESIAN_POINT('Ctrl Pts',(-16.2737775044129,-8.92195553365029,1.00027032776118));
#9446=CARTESIAN_POINT('Ctrl Pts',(-15.9175115607866,-8.50100124254812,0.96322327858484));
#9447=CARTESIAN_POINT('Ctrl Pts',(-15.3319382346072,-8.2741137068379,0.926176229408499));
#9448=CARTESIAN_POINT('Ctrl Pts',(-14.785052977246,-8.34515434993965,0.889129180232159));
#9449=CARTESIAN_POINT('Ctrl Pts',(-14.2381677198847,-8.4161949930414,0.852082131055818));
#9450=CARTESIAN_POINT('Ctrl Pts',(-13.7299705313417,-8.78516381495513,0.815035081879479));
#9451=CARTESIAN_POINT('Ctrl Pts',(-13.4930723773631,-9.28315331616688,0.777988032703139));
#9452=CARTESIAN_POINT('Ctrl Pts',(-13.2561742233845,-9.78114281737862,0.740940983526799));
#9453=CARTESIAN_POINT('Ctrl Pts',(-13.2905751039703,-10.4081529978884,0.703893934350459));
#9454=CARTESIAN_POINT('Ctrl Pts',(-13.5804932800309,-10.8772868894421,0.66684688517412));
#9455=CARTESIAN_POINT('Ctrl Pts',(-13.8704114560916,-11.3464207809959,0.629799835997779));
#9456=CARTESIAN_POINT('Ctrl Pts',(-14.4158469276272,-11.6576783835936,0.592752786821439));
#9457=CARTESIAN_POINT('Ctrl Pts',(-14.9672366648336,-11.6684613472114,0.555705737645099));
#9458=CARTESIAN_POINT('Ctrl Pts',(-15.51862640204,-11.6792443108291,0.518658688468759));
#9459=CARTESIAN_POINT('Ctrl Pts',(-16.0759704049172,-11.3895526354668,0.481611639292419));
#9460=CARTESIAN_POINT('Ctrl Pts',(-16.3840435298828,-10.9322477704337,0.444564590116079));
#9461=CARTESIAN_POINT('Ctrl Pts',(-16.5671141177547,-10.6604971252334,0.422549605613983));
#9462=CARTESIAN_POINT('Ctrl Pts',(-16.6621607121613,-10.3295579280615,0.400534621111888));
#9463=CARTESIAN_POINT('Ctrl Pts',(-16.6635932794994,-9.99933537909448,0.378519636609792));
#9464=CARTESIAN_POINT('Ctrl Pts',(-16.6671910371619,-9.99865073764983,0.571480363390209));
#9465=CARTESIAN_POINT('Ctrl Pts',(-16.6631433192538,-10.4622542356605,0.602548329955036));
#9466=CARTESIAN_POINT('Ctrl Pts',(-16.4613710696859,-10.9289661302211,0.633616296519864));
#9467=CARTESIAN_POINT('Ctrl Pts',(-16.118047013422,-11.2388249098967,0.664684263084691));
#9468=CARTESIAN_POINT('Ctrl Pts',(-15.7086496629616,-11.6083165347963,0.70173131226103));
#9469=CARTESIAN_POINT('Ctrl Pts',(-15.0979739909057,-11.7547722801968,0.738778361437369));
#9470=CARTESIAN_POINT('Ctrl Pts',(-14.5655171312584,-11.6111839010105,0.775825410613709));
#9471=CARTESIAN_POINT('Ctrl Pts',(-14.033060271611,-11.4675955218242,0.812872459790049));
#9472=CARTESIAN_POINT('Ctrl Pts',(-13.5788222243723,-11.033963018051,0.84991950896639));
#9473=CARTESIAN_POINT('Ctrl Pts',(-13.4106972420034,-10.5087402419385,0.886966558142731));
#9474=CARTESIAN_POINT('Ctrl Pts',(-13.2425722596345,-9.98351746582605,0.92401360731907));
#9475=CARTESIAN_POINT('Ctrl Pts',(-13.3605603421356,-9.36670441737438,0.961060656495409));
#9476=CARTESIAN_POINT('Ctrl Pts',(-13.7106614620273,-8.94061000038623,0.998107705671748));
#9477=CARTESIAN_POINT('Ctrl Pts',(-14.0607625819191,-8.51451558339806,1.03515475484809));
#9478=CARTESIAN_POINT('Ctrl Pts',(-14.6429767392015,-8.27913979787342,1.07220180402443));
#9479=CARTESIAN_POINT('Ctrl Pts',(-15.1908356179555,-8.34220651366761,1.10924885320077));
#9480=CARTESIAN_POINT('Ctrl Pts',(-15.7386944967096,-8.4052732294618,1.14629590237711));
#9481=CARTESIAN_POINT('Ctrl Pts',(-16.2521980969352,-8.76678244657481,1.18334295155345));
#9482=CARTESIAN_POINT('Ctrl Pts',(-16.4963261808093,-9.26128007721764,1.22039000072979));
#9483=CARTESIAN_POINT('Ctrl Pts',(-16.608549174885,-9.48859519718853,1.2374201216166));
#9484=CARTESIAN_POINT('Ctrl Pts',(-16.6638493580512,-9.74401262734354,1.2544502425034));
#9485=CARTESIAN_POINT('Ctrl Pts',(-16.6633491819668,-9.99963522328558,1.27148036339021));
#9486=CARTESIAN_POINT('Origin',(-15.,-10.,4.));
#9487=CARTESIAN_POINT('',(-16.6658558279687,-10.0015237952609,1.97148036339021));
#9488=CARTESIAN_POINT('',(-16.6687417861364,-9.99997573756952,1.7785196366098));
#9489=CARTESIAN_POINT('',(-16.666,-10.,4.));
#9490=CARTESIAN_POINT('Ctrl Pts',(-16.668741306591,-9.99997574181308,1.7785196366098));
#9491=CARTESIAN_POINT('Ctrl Pts',(-16.6688599435811,-9.44720213126613,1.74138549538496));
#9492=CARTESIAN_POINT('Ctrl Pts',(-16.3668274949188,-8.89454106233592,1.70425135416013));
#9493=CARTESIAN_POINT('Ctrl Pts',(-15.9017010646099,-8.59585115537534,1.6671172129353));
#9494=CARTESIAN_POINT('Ctrl Pts',(-15.4376655121909,-8.29786177668883,1.63007016375896));
#9495=CARTESIAN_POINT('Ctrl Pts',(-14.8113016140681,-8.2526536578585,1.59302311458262));
#9496=CARTESIAN_POINT('Ctrl Pts',(-14.3092835580737,-8.48091802869088,1.55597606540628));
#9497=CARTESIAN_POINT('Ctrl Pts',(-13.8072655020792,-8.70918239952326,1.51892901622994));
#9498=CARTESIAN_POINT('Ctrl Pts',(-13.4295932882132,-9.21091926001836,1.4818819670536));
#9499=CARTESIAN_POINT('Ctrl Pts',(-13.349120384328,-9.7564928551416,1.44483491787726));
#9500=CARTESIAN_POINT('Ctrl Pts',(-13.2686474804428,-10.3020664502648,1.40778786870092));
#9501=CARTESIAN_POINT('Ctrl Pts',(-13.4853738865385,-10.8914767800162,1.37074081952458));
#9502=CARTESIAN_POINT('Ctrl Pts',(-13.9001075103865,-11.2549637684195,1.33369377034824));
#9503=CARTESIAN_POINT('Ctrl Pts',(-14.3148411342344,-11.6184507568228,1.2966467211719));
#9504=CARTESIAN_POINT('Ctrl Pts',(-14.9275819758347,-11.7560144038781,1.25959967199556));
#9505=CARTESIAN_POINT('Ctrl Pts',(-15.4578920220932,-11.6046918718737,1.22255262281922));
#9506=CARTESIAN_POINT('Ctrl Pts',(-15.9882020683518,-11.4533693398692,1.18550557364288));
#9507=CARTESIAN_POINT('Ctrl Pts',(-16.4360813192687,-11.0131606288049,1.14845852446654));
#9508=CARTESIAN_POINT('Ctrl Pts',(-16.5965416641905,-10.4855457500257,1.1114114752902));
#9509=CARTESIAN_POINT('Ctrl Pts',(-16.6440293489689,-10.3293999492668,1.1004475290634));
#9510=CARTESIAN_POINT('Ctrl Pts',(-16.6663436334385,-10.1655987354384,1.08948358283659));
#9511=CARTESIAN_POINT('Ctrl Pts',(-16.6649907850313,-10.0014379678122,1.07851963660979));
#9512=CARTESIAN_POINT('Ctrl Pts',(-16.6633491819668,-9.99963522328558,1.27148036339021));
#9513=CARTESIAN_POINT('Ctrl Pts',(-16.6627612830976,-10.3000898827778,1.29149729167974));
#9514=CARTESIAN_POINT('Ctrl Pts',(-16.5850836763294,-10.6008279843625,1.31151421996927));
#9515=CARTESIAN_POINT('Ctrl Pts',(-16.4321390262416,-10.8565494596152,1.33153114825881));
#9516=CARTESIAN_POINT('Ctrl Pts',(-16.1490712202775,-11.3298351671973,1.36857819743515));
#9517=CARTESIAN_POINT('Ctrl Pts',(-15.6081830408266,-11.6489205381888,1.40562524661149));
#9518=CARTESIAN_POINT('Ctrl Pts',(-15.0570283710643,-11.6677669144638,1.44267229578783));
#9519=CARTESIAN_POINT('Ctrl Pts',(-14.505873701302,-11.6866132907387,1.47971934496417));
#9520=CARTESIAN_POINT('Ctrl Pts',(-13.9444525412283,-11.4052206722971,1.51676639414051));
#9521=CARTESIAN_POINT('Ctrl Pts',(-13.6297162289666,-10.9523766872749,1.55381344331685));
#9522=CARTESIAN_POINT('Ctrl Pts',(-13.3149799167049,-10.4995327022527,1.59086049249319));
#9523=CARTESIAN_POINT('Ctrl Pts',(-13.2469284522552,-9.87523735064986,1.62790754166953));
#9524=CARTESIAN_POINT('Ctrl Pts',(-13.4567076604804,-9.36521838263765,1.66495459084587));
#9525=CARTESIAN_POINT('Ctrl Pts',(-13.6664868687056,-8.85519941462545,1.70200164002221));
#9526=CARTESIAN_POINT('Ctrl Pts',(-14.1540967496057,-8.45945683020384,1.73904868919855));
#9527=CARTESIAN_POINT('Ctrl Pts',(-14.6963678920727,-8.35911413114816,1.77609573837489));
#9528=CARTESIAN_POINT('Ctrl Pts',(-15.2386390345398,-8.25877143209247,1.81314278755123));
#9529=CARTESIAN_POINT('Ctrl Pts',(-15.8355714385739,-8.45382861840273,1.85018983672757));
#9530=CARTESIAN_POINT('Ctrl Pts',(-16.213960946897,-8.85501190072828,1.88723688590391));
#9531=CARTESIAN_POINT('Ctrl Pts',(-16.5007750453132,-9.15910336967454,1.91531804506601));
#9532=CARTESIAN_POINT('Ctrl Pts',(-16.6620267716353,-9.58162322075589,1.94339920422811));
#9533=CARTESIAN_POINT('Ctrl Pts',(-16.6658558279687,-10.0015237952609,1.97148036339021));
#9534=CARTESIAN_POINT('Origin',(-15.,-10.,4.));
#9535=CARTESIAN_POINT('',(-16.6685090241476,-9.99943625435561,2.67148036339021));
#9536=CARTESIAN_POINT('',(-16.66492032495,-9.99857774531074,2.47851963660979));
#9537=CARTESIAN_POINT('',(-16.666,-10.,4.));
#9538=CARTESIAN_POINT('Ctrl Pts',(-16.66492032495,-9.99857774531074,2.47851963660979));
#9539=CARTESIAN_POINT('Ctrl Pts',(-16.6662755099423,-9.83179018295812,2.46738150628601));
#9540=CARTESIAN_POINT('Ctrl Pts',(-16.6432317570283,-9.66536855851988,2.45624337596222));
#9541=CARTESIAN_POINT('Ctrl Pts',(-16.594245932966,-9.50696967861907,2.44510524563844));
#9542=CARTESIAN_POINT('Ctrl Pts',(-16.4313119233769,-8.98011185575535,2.4080581964621));
#9543=CARTESIAN_POINT('Ctrl Pts',(-15.9813743433956,-8.54201164647713,2.37101114728576));
#9544=CARTESIAN_POINT('Ctrl Pts',(-15.4503607308701,-8.39317885267126,2.33396409810942));
#9545=CARTESIAN_POINT('Ctrl Pts',(-14.9193471183446,-8.24434605886539,2.29691704893308));
#9546=CARTESIAN_POINT('Ctrl Pts',(-14.307257473275,-8.38478068053188,2.25986999975674));
#9547=CARTESIAN_POINT('Ctrl Pts',(-13.8942331229627,-8.75020857436374,2.2228229505804));
#9548=CARTESIAN_POINT('Ctrl Pts',(-13.4812087726504,-9.1156364681956,2.18577590140406));
#9549=CARTESIAN_POINT('Ctrl Pts',(-13.2672497170955,-9.70605763419282,2.14872885222772));
#9550=CARTESIAN_POINT('Ctrl Pts',(-13.3502807933188,-10.2512479626338,2.11168180305138));
#9551=CARTESIAN_POINT('Ctrl Pts',(-13.433311869542,-10.7964382910748,2.07463475387504));
#9552=CARTESIAN_POINT('Ctrl Pts',(-13.8133330775434,-11.2963977819595,2.0375877046987));
#9553=CARTESIAN_POINT('Ctrl Pts',(-14.3164162094338,-11.5223048855013,2.00054065552236));
#9554=CARTESIAN_POINT('Ctrl Pts',(-14.8194993413241,-11.7482119890431,1.96349360634602));
#9555=CARTESIAN_POINT('Ctrl Pts',(-15.4456443971033,-11.700066705242,1.92644655716968));
#9556=CARTESIAN_POINT('Ctrl Pts',(-15.9082771879223,-11.3999041282926,1.88939950799334));
#9557=CARTESIAN_POINT('Ctrl Pts',(-16.3698223985333,-11.1004471884798,1.85243955086549));
#9558=CARTESIAN_POINT('Ctrl Pts',(-16.6686232260882,-10.5501564723576,1.81547959373764));
#9559=CARTESIAN_POINT('Ctrl Pts',(-16.668741306591,-9.99997574181308,1.7785196366098));
#9560=CARTESIAN_POINT('Ctrl Pts',(-16.6658558279687,-10.0015237952609,1.97148036339021));
#9561=CARTESIAN_POINT('Ctrl Pts',(-16.6670783878262,-10.1355917069947,1.98044625340445));
#9562=CARTESIAN_POINT('Ctrl Pts',(-16.6522528327537,-10.2693926022211,1.98941214341869));
#9563=CARTESIAN_POINT('Ctrl Pts',(-16.6203421479384,-10.3989865235809,1.99837803343293));
#9564=CARTESIAN_POINT('Ctrl Pts',(-16.4884872280444,-10.9344684857673,2.03542508260927));
#9565=CARTESIAN_POINT('Ctrl Pts',(-16.0649307756441,-11.3981230317991,2.07247213178561));
#9566=CARTESIAN_POINT('Ctrl Pts',(-15.5435262072274,-11.5777446491442,2.10951918096195));
#9567=CARTESIAN_POINT('Ctrl Pts',(-15.0221216388108,-11.7573662664892,2.14656623013829));
#9568=CARTESIAN_POINT('Ctrl Pts',(-14.4028689543777,-11.6529549551475,2.18361327931463));
#9569=CARTESIAN_POINT('Ctrl Pts',(-13.9691878657227,-11.3122977043507,2.22066032849097));
#9570=CARTESIAN_POINT('Ctrl Pts',(-13.5355067770677,-10.9716404535538,2.25770737766731));
#9571=CARTESIAN_POINT('Ctrl Pts',(-13.2873972841907,-10.3947372633017,2.29475442684365));
#9572=CARTESIAN_POINT('Ctrl Pts',(-13.3384141976562,-9.84562532165677,2.33180147601999));
#9573=CARTESIAN_POINT('Ctrl Pts',(-13.3894311111217,-9.29651338001179,2.36884852519633));
#9574=CARTESIAN_POINT('Ctrl Pts',(-13.7395744309295,-8.77519268697389,2.40589557437267));
#9575=CARTESIAN_POINT('Ctrl Pts',(-14.2285904810596,-8.52026141726962,2.44294262354901));
#9576=CARTESIAN_POINT('Ctrl Pts',(-14.7176065311896,-8.26533014756536,2.47998967272535));
#9577=CARTESIAN_POINT('Ctrl Pts',(-15.3454953116418,-8.27678830119472,2.51703672190169));
#9578=CARTESIAN_POINT('Ctrl Pts',(-15.8248845397239,-8.54939170829145,2.55408377107803));
#9579=CARTESIAN_POINT('Ctrl Pts',(-16.3042737678059,-8.82199511538819,2.59113082025437));
#9580=CARTESIAN_POINT('Ctrl Pts',(-16.6351634435178,-9.3557437759523,2.62817786943071));
#9581=CARTESIAN_POINT('Ctrl Pts',(-16.6661119032437,-9.90635147885495,2.66522491860705));
#9582=CARTESIAN_POINT('Ctrl Pts',(-16.6678537997891,-9.93734176606421,2.6673100668681));
#9583=CARTESIAN_POINT('Ctrl Pts',(-16.6686455231177,-9.96838546044008,2.66939521512916));
#9584=CARTESIAN_POINT('Ctrl Pts',(-16.6685090241476,-9.99943625435561,2.67148036339021));
#9585=CARTESIAN_POINT('Origin',(-15.,-10.,4.));
#9586=CARTESIAN_POINT('',(-16.6641896916198,-9.99883056905918,3.37148036339021));
#9587=CARTESIAN_POINT('',(-16.6637100014683,-10.0008527826236,3.17851963660979));
#9588=CARTESIAN_POINT('',(-16.666,-10.,4.));
#9589=CARTESIAN_POINT('Ctrl Pts',(-16.6637100014683,-10.0008527826236,3.17851963660979));
#9590=CARTESIAN_POINT('Ctrl Pts',(-16.6621664007059,-9.66797331594755,3.15633046801071));
#9591=CARTESIAN_POINT('Ctrl Pts',(-16.56543951406,-9.33426787425992,3.13414129941163));
#9592=CARTESIAN_POINT('Ctrl Pts',(-16.379615276458,-9.06119188318812,3.11195213081255));
#9593=CARTESIAN_POINT('Ctrl Pts',(-16.0693630181159,-8.60526404502054,3.07490508163621));
#9594=CARTESIAN_POINT('Ctrl Pts',(-15.5107459993938,-8.31834481162707,3.03785803245988));
#9595=CARTESIAN_POINT('Ctrl Pts',(-14.9594321871066,-8.3317514442721,3.00081098328354));
#9596=CARTESIAN_POINT('Ctrl Pts',(-14.4081183748194,-8.34515807691714,2.9637639341072));
#9597=CARTESIAN_POINT('Ctrl Pts',(-13.864107768967,-8.65889057560069,2.92671688493085));
#9598=CARTESIAN_POINT('Ctrl Pts',(-13.5763832698313,-9.12935977764045,2.88966983575451));
#9599=CARTESIAN_POINT('Ctrl Pts',(-13.2886587706957,-9.59982897968023,2.85262278657817));
#9600=CARTESIAN_POINT('Ctrl Pts',(-13.2572203782769,-10.2270348850762,2.81557573740184));
#9601=CARTESIAN_POINT('Ctrl Pts',(-13.4964568234424,-10.7239177492225,2.7785286882255));
#9602=CARTESIAN_POINT('Ctrl Pts',(-13.7356932686079,-11.2208006133687,2.74148163904916));
#9603=CARTESIAN_POINT('Ctrl Pts',(-14.2456045513576,-11.5873604362652,2.70443458987282));
#9604=CARTESIAN_POINT('Ctrl Pts',(-14.792814357206,-11.6558300335834,2.66738754069648));
#9605=CARTESIAN_POINT('Ctrl Pts',(-15.3400241630545,-11.7242996309016,2.63034049152013));
#9606=CARTESIAN_POINT('Ctrl Pts',(-15.9245324920015,-11.4946790026414,2.5932934423438));
#9607=CARTESIAN_POINT('Ctrl Pts',(-16.2788214368767,-11.0720609702867,2.55624639316746));
#9608=CARTESIAN_POINT('Ctrl Pts',(-16.5265940321902,-10.7765023077388,2.5303374743149));
#9609=CARTESIAN_POINT('Ctrl Pts',(-16.6617679666121,-10.3865499895734,2.50442855546235));
#9610=CARTESIAN_POINT('Ctrl Pts',(-16.66492032495,-9.99857774531074,2.47851963660979));
#9611=CARTESIAN_POINT('Ctrl Pts',(-16.6685090241476,-9.99943625435561,2.67148036339021));
#9612=CARTESIAN_POINT('Ctrl Pts',(-16.6662203315139,-10.5200681923775,2.7064422643055));
#9613=CARTESIAN_POINT('Ctrl Pts',(-16.4029750948965,-11.0426960653573,2.74140416522078));
#9614=CARTESIAN_POINT('Ctrl Pts',(-15.9822463015998,-11.3490334030561,2.77636606613607));
#9615=CARTESIAN_POINT('Ctrl Pts',(-15.5364249964903,-11.6736408791134,2.81341311531241));
#9616=CARTESIAN_POINT('Ctrl Pts',(-14.9137751425314,-11.7553890859868,2.85046016448875));
#9617=CARTESIAN_POINT('Ctrl Pts',(-14.3992712693864,-11.5568634853063,2.88750721366509));
#9618=CARTESIAN_POINT('Ctrl Pts',(-13.8847673962414,-11.3583378846257,2.92455426284143));
#9619=CARTESIAN_POINT('Ctrl Pts',(-13.4784095039101,-10.8795384763911,2.96160131201777));
#9620=CARTESIAN_POINT('Ctrl Pts',(-13.3661795668735,-10.3396022849287,2.99864836119411));
#9621=CARTESIAN_POINT('Ctrl Pts',(-13.2539496298369,-9.7996660934662,3.03569541037045));
#9622=CARTESIAN_POINT('Ctrl Pts',(-13.4358476480949,-9.19859311877586,3.07274245954679));
#9623=CARTESIAN_POINT('Ctrl Pts',(-13.828622494431,-8.81148257939958,3.10978950872313));
#9624=CARTESIAN_POINT('Ctrl Pts',(-14.2213973407671,-8.42437204002329,3.14683655789947));
#9625=CARTESIAN_POINT('Ctrl Pts',(-14.8250490151812,-8.25122393596108,3.18388360707581));
#9626=CARTESIAN_POINT('Ctrl Pts',(-15.3632980792249,-8.37128473167712,3.22093065625215));
#9627=CARTESIAN_POINT('Ctrl Pts',(-15.9015471432685,-8.49134552739316,3.25797770542849));
#9628=CARTESIAN_POINT('Ctrl Pts',(-16.3743935969416,-8.90461522288745,3.29502475460483));
#9629=CARTESIAN_POINT('Ctrl Pts',(-16.5654249655814,-9.4219484480033,3.33207180378117));
#9630=CARTESIAN_POINT('Ctrl Pts',(-16.6331610943294,-9.60538507514802,3.34520799031751));
#9631=CARTESIAN_POINT('Ctrl Pts',(-16.6654652280384,-9.80190538255376,3.35834417685386));
#9632=CARTESIAN_POINT('Ctrl Pts',(-16.6641896916198,-9.99883056905918,3.37148036339021));
#9633=CARTESIAN_POINT('Origin',(-15.,-10.,4.));
#9634=CARTESIAN_POINT('',(-16.6642806992699,-10.0012124486558,4.07148036339022));
#9635=CARTESIAN_POINT('',(-16.6680323256648,-10.0009660456509,3.8785196366098));
#9636=CARTESIAN_POINT('',(-16.666,-10.,4.));
#9637=CARTESIAN_POINT('Ctrl Pts',(-16.6680323256648,-10.0009660456509,3.8785196366098));
#9638=CARTESIAN_POINT('Ctrl Pts',(-16.6646132194972,-9.50559820416748,3.84527942973542));
#9639=CARTESIAN_POINT('Ctrl Pts',(-16.4297940876874,-9.00741573513633,3.81203922286105));
#9640=CARTESIAN_POINT('Ctrl Pts',(-16.0437119187986,-8.6979383955612,3.77879901598668));
#9641=CARTESIAN_POINT('Ctrl Pts',(-15.613413601132,-8.35301809282261,3.74175196681034));
#9642=CARTESIAN_POINT('Ctrl Pts',(-14.995221408247,-8.24250097761573,3.704704917634));
#9643=CARTESIAN_POINT('Ctrl Pts',(-14.4720696864628,-8.41696854887757,3.66765786845765));
#9644=CARTESIAN_POINT('Ctrl Pts',(-13.9489179646786,-8.59143612013942,3.63061081928131));
#9645=CARTESIAN_POINT('Ctrl Pts',(-13.5208067139953,-9.05088837786998,3.59356377010497));
#9646=CARTESIAN_POINT('Ctrl Pts',(-13.3836739909864,-9.58504310611734,3.55651672092863));
#9647=CARTESIAN_POINT('Ctrl Pts',(-13.2465412679775,-10.1191978343647,3.51946967175229));
#9648=CARTESIAN_POINT('Ctrl Pts',(-13.4003870726431,-10.7280550331288,3.48242262257595));
#9649=CARTESIAN_POINT('Ctrl Pts',(-13.7747992213996,-11.1329527983623,3.44537557339961));
#9650=CARTESIAN_POINT('Ctrl Pts',(-14.1492113701561,-11.5378505635958,3.40832852422327));
#9651=CARTESIAN_POINT('Ctrl Pts',(-14.7441898630034,-11.7387888952986,3.37128147504694));
#9652=CARTESIAN_POINT('Ctrl Pts',(-15.2874248052393,-11.6438022911897,3.3342344258706));
#9653=CARTESIAN_POINT('Ctrl Pts',(-15.8306597474752,-11.5488156870807,3.29718737669426));
#9654=CARTESIAN_POINT('Ctrl Pts',(-16.3221511390998,-11.1579041471599,3.26014032751792));
#9655=CARTESIAN_POINT('Ctrl Pts',(-16.536953085931,-10.6499801557287,3.22309327834158));
#9656=CARTESIAN_POINT('Ctrl Pts',(-16.6231003431279,-10.4462750246914,3.20823539776432));
#9657=CARTESIAN_POINT('Ctrl Pts',(-16.6647435974628,-10.2237490727847,3.19337751718705));
#9658=CARTESIAN_POINT('Ctrl Pts',(-16.6637100014683,-10.0008527826236,3.17851963660979));
#9659=CARTESIAN_POINT('Ctrl Pts',(-16.6641896916198,-9.99883056905918,3.37148036339021));
#9660=CARTESIAN_POINT('Ctrl Pts',(-16.6618679237299,-10.3572794287687,3.3953912260302));
#9661=CARTESIAN_POINT('Ctrl Pts',(-16.548288911008,-10.7170697469545,3.4193020886702));
#9662=CARTESIAN_POINT('Ctrl Pts',(-16.3346237287904,-11.0017377012874,3.44321295131019));
#9663=CARTESIAN_POINT('Ctrl Pts',(-16.0035748397532,-11.4427969747182,3.48026000048653));
#9664=CARTESIAN_POINT('Ctrl Pts',(-15.4322607780725,-11.7035187668424,3.51730704966287));
#9665=CARTESIAN_POINT('Ctrl Pts',(-14.8821606960968,-11.6645758673272,3.55435409883921));
#9666=CARTESIAN_POINT('Ctrl Pts',(-14.3320606141211,-11.6256329678119,3.59140114801554));
#9667=CARTESIAN_POINT('Ctrl Pts',(-13.8031745118505,-11.2870253766572,3.62844819719188));
#9668=CARTESIAN_POINT('Ctrl Pts',(-13.5375631033236,-10.8037270947724,3.66549524636822));
#9669=CARTESIAN_POINT('Ctrl Pts',(-13.2719516947968,-10.3204288128875,3.70254229554456));
#9670=CARTESIAN_POINT('Ctrl Pts',(-13.2696149800139,-9.69243984027253,3.73958934472091));
#9671=CARTESIAN_POINT('Ctrl Pts',(-13.5316224271389,-9.2071783156661,3.77663639389725));
#9672=CARTESIAN_POINT('Ctrl Pts',(-13.7936298742639,-8.72191679105968,3.81368344307359));
#9673=CARTESIAN_POINT('Ctrl Pts',(-14.3199814832969,-8.37938271446182,3.85073049224993));
#9674=CARTESIAN_POINT('Ctrl Pts',(-14.8697765276525,-8.33634716155033,3.88777754142627));
#9675=CARTESIAN_POINT('Ctrl Pts',(-15.419571572008,-8.29331160863883,3.92482459060261));
#9676=CARTESIAN_POINT('Ctrl Pts',(-15.9928100516862,-8.54977457941371,3.96187163977894));
#9677=CARTESIAN_POINT('Ctrl Pts',(-16.3271320462624,-8.98835804188682,3.99891868895528));
#9678=CARTESIAN_POINT('Ctrl Pts',(-16.5454037149127,-9.27469978951192,4.02310591376693));
#9679=CARTESIAN_POINT('Ctrl Pts',(-16.6618371270144,-9.63867047659017,4.04729313857857));
#9680=CARTESIAN_POINT('Ctrl Pts',(-16.6642806992699,-10.0012124486558,4.07148036339022));
#9681=CARTESIAN_POINT('Origin',(-15.,-10.,4.));
#9682=CARTESIAN_POINT('',(-16.6685641984665,-10.0004924312751,4.77148036339021));
#9683=CARTESIAN_POINT('',(-16.6666360603741,-9.99853839705222,4.5785196366098));
#9684=CARTESIAN_POINT('',(-16.666,-10.,4.));
#9685=CARTESIAN_POINT('Ctrl Pts',(-16.6666360603741,-9.99853839705222,4.5785196366098));
#9686=CARTESIAN_POINT('Ctrl Pts',(-16.6676284318155,-9.89034513840702,4.57127544063647));
#9687=CARTESIAN_POINT('Ctrl Pts',(-16.6579946985884,-9.78232782481888,4.56403124466314));
#9688=CARTESIAN_POINT('Ctrl Pts',(-16.6370921504892,-9.67653704694216,4.55678704868981));
#9689=CARTESIAN_POINT('Ctrl Pts',(-16.5301958530681,-9.13551963592343,4.51973999951347));
#9690=CARTESIAN_POINT('Ctrl Pts',(-16.1285826105747,-8.65273353053979,4.48269295033713));
#9691=CARTESIAN_POINT('Ctrl Pts',(-15.6160628650447,-8.44914038755636,4.44564590116079));
#9692=CARTESIAN_POINT('Ctrl Pts',(-15.1035431195147,-8.24554724457292,4.40859885198445));
#9693=CARTESIAN_POINT('Ctrl Pts',(-14.4801168709481,-8.32114706398968,4.37155180280812));
#9694=CARTESIAN_POINT('Ctrl Pts',(-14.031113989483,-8.64133930290906,4.33450475363177));
#9695=CARTESIAN_POINT('Ctrl Pts',(-13.582111108018,-8.96153154182844,4.29745770445543));
#9696=CARTESIAN_POINT('Ctrl Pts',(-13.3075315936544,-9.52631620025045,4.26041065527909));
#9697=CARTESIAN_POINT('Ctrl Pts',(-13.3330450622543,-10.0772025046255,4.22336360610275));
#9698=CARTESIAN_POINT('Ctrl Pts',(-13.3585585308543,-10.6280888090006,4.18631655692641));
#9699=CARTESIAN_POINT('Ctrl Pts',(-13.6841649824178,-11.1650767593287,4.14926950775007));
#9700=CARTESIAN_POINT('Ctrl Pts',(-14.160840780622,-11.4423975858716,4.11222245857374));
#9701=CARTESIAN_POINT('Ctrl Pts',(-14.6375165788261,-11.7197184124145,4.0751754093974));
#9702=CARTESIAN_POINT('Ctrl Pts',(-15.265261723671,-11.7373721151722,4.03812836022106));
#9703=CARTESIAN_POINT('Ctrl Pts',(-15.7567696715678,-11.4872789433695,4.00108131104471));
#9704=CARTESIAN_POINT('Ctrl Pts',(-16.2482776194645,-11.2371857715668,3.96403426186837));
#9705=CARTESIAN_POINT('Ctrl Pts',(-16.6035483704131,-10.7193457252036,3.92698721269203));
#9706=CARTESIAN_POINT('Ctrl Pts',(-16.6599815246633,-10.1707639568869,3.88994016351569));
#9707=CARTESIAN_POINT('Ctrl Pts',(-16.6657804242682,-10.1143933598178,3.88613332121373));
#9708=CARTESIAN_POINT('Ctrl Pts',(-16.6684238995814,-10.0576981611013,3.88232647891176));
#9709=CARTESIAN_POINT('Ctrl Pts',(-16.6680323256648,-10.0009660456509,3.8785196366098));
#9710=CARTESIAN_POINT('Ctrl Pts',(-16.6642806992699,-10.0012124486558,4.07148036339022));
#9711=CARTESIAN_POINT('Ctrl Pts',(-16.665579893794,-10.1939681749494,4.08434018775491));
#9712=CARTESIAN_POINT('Ctrl Pts',(-16.6346562245379,-10.3863200293777,4.09720001211961));
#9713=CARTESIAN_POINT('Ctrl Pts',(-16.5696833589659,-10.5663859745943,4.11005983648431));
#9714=CARTESIAN_POINT('Ctrl Pts',(-16.382507167619,-11.0851264906573,4.14710688566065));
#9715=CARTESIAN_POINT('Ctrl Pts',(-15.9127492754508,-11.5019035686119,4.18415393483698));
#9716=CARTESIAN_POINT('Ctrl Pts',(-15.3754085835772,-11.6259665786876,4.22120098401332));
#9717=CARTESIAN_POINT('Ctrl Pts',(-14.8380678917035,-11.7500295887632,4.25824803318966));
#9718=CARTESIAN_POINT('Ctrl Pts',(-14.2331444001243,-11.5813785309599,4.29529508236601));
#9719=CARTESIAN_POINT('Ctrl Pts',(-13.8374996328648,-11.1972016605574,4.33234213154235));
#9720=CARTESIAN_POINT('Ctrl Pts',(-13.4418548656054,-10.8130247901549,4.36938918071869));
#9721=CARTESIAN_POINT('Ctrl Pts',(-13.2554888226657,-10.2133221071532,4.40643622989502));
#9722=CARTESIAN_POINT('Ctrl Pts',(-13.3636975578329,-9.67256567469336,4.44348327907136));
#9723=CARTESIAN_POINT('Ctrl Pts',(-13.471906293,-9.13180924223355,4.4805303282477));
#9724=CARTESIAN_POINT('Ctrl Pts',(-13.8746898062741,-8.64999906031561,4.51757737742405));
#9725=CARTESIAN_POINT('Ctrl Pts',(-14.387702045816,-8.44765012483052,4.55462442660039));
#9726=CARTESIAN_POINT('Ctrl Pts',(-14.900714285358,-8.24530118934543,4.59167147577673));
#9727=CARTESIAN_POINT('Ctrl Pts',(-15.5239552511679,-8.3224135002932,4.62871852495307));
#9728=CARTESIAN_POINT('Ctrl Pts',(-15.9721798733629,-8.64369427729152,4.6657655741294));
#9729=CARTESIAN_POINT('Ctrl Pts',(-16.398520364984,-8.94928883330469,4.70100383721634));
#9730=CARTESIAN_POINT('Ctrl Pts',(-16.6665173165624,-9.47579132558647,4.73624210030327));
#9731=CARTESIAN_POINT('Ctrl Pts',(-16.6685641984665,-10.0004924312751,4.77148036339021));
#9732=CARTESIAN_POINT('Origin',(-15.,-10.,4.));
#9733=CARTESIAN_POINT('',(-16.6657318647841,-9.99847819321684,5.47148036339021));
#9734=CARTESIAN_POINT('',(-16.6632775623115,-9.9999437523457,5.2785196366098));
#9735=CARTESIAN_POINT('',(-16.666,-10.,4.));
#9736=CARTESIAN_POINT('Ctrl Pts',(-16.6632775623115,-9.9999437523457,5.2785196366098));
#9737=CARTESIAN_POINT('Ctrl Pts',(-16.6633602649375,-9.72530233420805,5.26022440236118));
#9738=CARTESIAN_POINT('Ctrl Pts',(-16.5991043467443,-9.45069734119511,5.24192916811256));
#9739=CARTESIAN_POINT('Ctrl Pts',(-16.4702970143586,-9.210743590017,5.22363393386394));
#9740=CARTESIAN_POINT('Ctrl Pts',(-16.2094677999131,-8.72484773871831,5.1865868846876));
#9741=CARTESIAN_POINT('Ctrl Pts',(-15.6839488768039,-8.3810374981041,5.14953983551125));
#9742=CARTESIAN_POINT('Ctrl Pts',(-15.134259867688,-8.33666801895819,5.11249278633491));
#9743=CARTESIAN_POINT('Ctrl Pts',(-14.584570858572,-8.29229853981227,5.07544573715857));
#9744=CARTESIAN_POINT('Ctrl Pts',(-14.0107117634493,-8.54736982213464,5.03839868798223));
#9745=CARTESIAN_POINT('Ctrl Pts',(-13.6753265461866,-8.98514078219886,5.00135163880589));
#9746=CARTESIAN_POINT('Ctrl Pts',(-13.3399413289238,-9.42291174226308,4.96430458962955));
#9747=CARTESIAN_POINT('Ctrl Pts',(-13.2430299895211,-10.0433823800691,4.92725754045321));
#9748=CARTESIAN_POINT('Ctrl Pts',(-13.4289469322776,-10.562575550115,4.89021049127687));
#9749=CARTESIAN_POINT('Ctrl Pts',(-13.6148638750341,-11.0817687201609,4.85316344210053));
#9750=CARTESIAN_POINT('Ctrl Pts',(-14.0836090999499,-11.4996844224466,4.81611639292419));
#9751=CARTESIAN_POINT('Ctrl Pts',(-14.6206471836982,-11.6250509013455,4.77906934374785));
#9752=CARTESIAN_POINT('Ctrl Pts',(-15.1576852674464,-11.7504173802444,4.74202229457151));
#9753=CARTESIAN_POINT('Ctrl Pts',(-15.7630162100271,-11.5832346357565,4.70497524539517));
#9754=CARTESIAN_POINT('Ctrl Pts',(-16.1595920051431,-11.2000189051856,4.66792819621883));
#9755=CARTESIAN_POINT('Ctrl Pts',(-16.4786211982497,-10.8917373438411,4.63812534301582));
#9756=CARTESIAN_POINT('Ctrl Pts',(-16.6625534126244,-10.4436489126747,4.60832248981281));
#9757=CARTESIAN_POINT('Ctrl Pts',(-16.6666360603741,-9.99853839705222,4.5785196366098));
#9758=CARTESIAN_POINT('Ctrl Pts',(-16.6685641984665,-10.0004924312751,4.77148036339021));
#9759=CARTESIAN_POINT('Ctrl Pts',(-16.6686692652657,-10.027425429043,4.77328914947961));
#9760=CARTESIAN_POINT('Ctrl Pts',(-16.6680736104087,-10.0543536805418,4.77509793556902));
#9761=CARTESIAN_POINT('Ctrl Pts',(-16.6667626807532,-10.0812470656621,4.77690672165842));
#9762=CARTESIAN_POINT('Ctrl Pts',(-16.6399125873683,-10.6320698339855,4.81395377083476));
#9763=CARTESIAN_POINT('Ctrl Pts',(-16.3130041220183,-11.1682661275834,4.85100082001111));
#9764=CARTESIAN_POINT('Ctrl Pts',(-15.8356568269973,-11.4444295023148,4.88804786918745));
#9765=CARTESIAN_POINT('Ctrl Pts',(-15.3583095319764,-11.7205928770462,4.92509491836379));
#9766=CARTESIAN_POINT('Ctrl Pts',(-14.7305234072845,-11.736723332911,4.96214196754013));
#9767=CARTESIAN_POINT('Ctrl Pts',(-14.2396237521779,-11.485438279201,4.99918901671646));
#9768=CARTESIAN_POINT('Ctrl Pts',(-13.7487240970713,-11.234153225491,5.0362360658928));
#9769=CARTESIAN_POINT('Ctrl Pts',(-13.3947109115499,-10.7154526622061,5.07328311506915));
#9770=CARTESIAN_POINT('Ctrl Pts',(-13.3396090325246,-10.1667355833913,5.11033016424549));
#9771=CARTESIAN_POINT('Ctrl Pts',(-13.2845071534992,-9.61801850457656,5.14737721342183));
#9772=CARTESIAN_POINT('Ctrl Pts',(-13.52831658097,-9.03928491023192,5.18442426259817));
#9773=CARTESIAN_POINT('Ctrl Pts',(-13.9594505595911,-8.6954097264222,5.22147131177451));
#9774=CARTESIAN_POINT('Ctrl Pts',(-14.3905845382122,-8.35153454261247,5.25851836095085));
#9775=CARTESIAN_POINT('Ctrl Pts',(-15.0090430679838,-8.24251776933766,5.29556541012719));
#9776=CARTESIAN_POINT('Ctrl Pts',(-15.5317699054477,-8.41825422814124,5.33261245930353));
#9777=CARTESIAN_POINT('Ctrl Pts',(-16.0544967429115,-8.59399068694482,5.36965950847986));
#9778=CARTESIAN_POINT('Ctrl Pts',(-16.4814918880678,-9.0544803778268,5.4067065576562));
#9779=CARTESIAN_POINT('Ctrl Pts',(-16.6173281038004,-9.5889662732554,5.44375360683254));
#9780=CARTESIAN_POINT('Ctrl Pts',(-16.6512156222314,-9.72230627050696,5.45299585901843));
#9781=CARTESIAN_POINT('Ctrl Pts',(-16.6669822934182,-9.86025156673352,5.46223811120432));
#9782=CARTESIAN_POINT('Ctrl Pts',(-16.6657318647841,-9.99847819321684,5.47148036339021));
#9783=CARTESIAN_POINT('Origin',(-15.,-10.,4.));
#9784=CARTESIAN_POINT('',(-16.6633787344493,-10.0004304228837,6.17148036339021));
#9785=CARTESIAN_POINT('',(-16.6664295714326,-10.0014906689886,5.9785196366098));
#9786=CARTESIAN_POINT('',(-16.666,-10.,4.));
#9787=CARTESIAN_POINT('Ctrl Pts',(-16.6664295714326,-10.0014906689886,5.9785196366098));
#9788=CARTESIAN_POINT('Ctrl Pts',(-16.6623836036609,-9.56305953449899,5.94917336408588));
#9789=CARTESIAN_POINT('Ctrl Pts',(-16.4846437757866,-9.1217262956008,5.91982709156197));
#9790=CARTESIAN_POINT('Ctrl Pts',(-16.1742579544333,-8.81432835748561,5.89048081903805));
#9791=CARTESIAN_POINT('Ctrl Pts',(-15.7824235646333,-8.42626590353074,5.85343376986171));
#9792=CARTESIAN_POINT('Ctrl Pts',(-15.179193796671,-8.2516535720841,5.81638672068537));
#9793=CARTESIAN_POINT('Ctrl Pts',(-14.6406549885415,-8.37040797887343,5.77933967150903));
#9794=CARTESIAN_POINT('Ctrl Pts',(-14.1021161804119,-8.48916238566276,5.74229262233269));
#9795=CARTESIAN_POINT('Ctrl Pts',(-13.6282683321152,-8.90128353068805,5.70524557315636));
#9796=CARTESIAN_POINT('Ctrl Pts',(-13.4359822379784,-9.4181517109175,5.66819852398001));
#9797=CARTESIAN_POINT('Ctrl Pts',(-13.2436961438415,-9.93501989114696,5.63115147480367));
#9798=CARTESIAN_POINT('Ctrl Pts',(-13.3329718038647,-10.5566351065806,5.59410442562733));
#9799=CARTESIAN_POINT('Ctrl Pts',(-13.6629495126592,-10.9984963620356,5.55705737645099));
#9800=CARTESIAN_POINT('Ctrl Pts',(-13.9929272214536,-11.4403576174907,5.52001032727465));
#9801=CARTESIAN_POINT('Ctrl Pts',(-14.5636069790195,-11.7024649129672,5.48296327809831));
#9802=CARTESIAN_POINT('Ctrl Pts',(-15.1137999417662,-11.6648569201785,5.44591622892197));
#9803=CARTESIAN_POINT('Ctrl Pts',(-15.6639929045129,-11.6272489273898,5.40886917974563));
#9804=CARTESIAN_POINT('Ctrl Pts',(-16.1936990724405,-11.2899256463359,5.37182213056929));
#9805=CARTESIAN_POINT('Ctrl Pts',(-16.4604824035133,-10.8072732748174,5.33477508139295));
#9806=CARTESIAN_POINT('Ctrl Pts',(-16.5955180341857,-10.5629729014716,5.31602326646523));
#9807=CARTESIAN_POINT('Ctrl Pts',(-16.663192795737,-10.2814391939682,5.29727145153752));
#9808=CARTESIAN_POINT('Ctrl Pts',(-16.6632775623115,-9.9999437523457,5.2785196366098));
#9809=CARTESIAN_POINT('Ctrl Pts',(-16.6657318647841,-9.99847819321684,5.47148036339021));
#9810=CARTESIAN_POINT('Ctrl Pts',(-16.661970020417,-10.4143252411811,5.49928516038066));
#9811=CARTESIAN_POINT('Ctrl Pts',(-16.5041909226578,-10.8327185346218,5.52708995737111));
#9812=CARTESIAN_POINT('Ctrl Pts',(-16.2224480983357,-11.1359223423689,5.55489475436156));
#9813=CARTESIAN_POINT('Ctrl Pts',(-15.8470545908295,-11.5399104160786,5.5919418035379));
#9814=CARTESIAN_POINT('Ctrl Pts',(-15.2515902895082,-11.7394044635228,5.62898885271425));
#9815=CARTESIAN_POINT('Ctrl Pts',(-14.7085874340879,-11.6431000067782,5.66603590189058));
#9816=CARTESIAN_POINT('Ctrl Pts',(-14.1655845786677,-11.5467955500336,5.70308295106692));
#9817=CARTESIAN_POINT('Ctrl Pts',(-13.6750431691484,-11.1546925891003,5.74013000024326));
#9818=CARTESIAN_POINT('Ctrl Pts',(-13.461474311529,-10.6462488903663,5.7771770494196));
#9819=CARTESIAN_POINT('Ctrl Pts',(-13.2479054539096,-10.1378051916323,5.81422409859594));
#9820=CARTESIAN_POINT('Ctrl Pts',(-13.3113091481901,-9.51302075509764,5.85127114777229));
#9821=CARTESIAN_POINT('Ctrl Pts',(-13.6226667771701,-9.05784708175693,5.88831819694863));
#9822=CARTESIAN_POINT('Ctrl Pts',(-13.9340244061501,-8.60267340841622,5.92536524612496));
#9823=CARTESIAN_POINT('Ctrl Pts',(-14.4933359698297,-8.31711049826945,5.9624122953013));
#9824=CARTESIAN_POINT('Ctrl Pts',(-15.044615621323,-8.3318548210974,5.99945934447764));
#9825=CARTESIAN_POINT('Ctrl Pts',(-15.5958952728164,-8.34659914392535,6.03650639365398));
#9826=CARTESIAN_POINT('Ctrl Pts',(-16.1391430121236,-8.66165069972803,6.07355344283032));
#9827=CARTESIAN_POINT('Ctrl Pts',(-16.4257250890118,-9.13281667594263,6.11060049200666));
#9828=CARTESIAN_POINT('Ctrl Pts',(-16.582706372449,-9.39090762308494,6.13089378246785));
#9829=CARTESIAN_POINT('Ctrl Pts',(-16.6626744024472,-9.6958411408748,6.15118707292903));
#9830=CARTESIAN_POINT('Ctrl Pts',(-16.6633787344493,-10.0004304228837,6.17148036339021));
#9831=CARTESIAN_POINT('Origin',(-15.,-10.,4.));
#9832=CARTESIAN_POINT('',(-16.6673099838652,-10.001299617498,6.87148036339021));
#9833=CARTESIAN_POINT('',(-16.6681788248613,-9.99913246376521,6.6785196366098));
#9834=CARTESIAN_POINT('',(-16.666,-10.,4.));
#9835=CARTESIAN_POINT('Ctrl Pts',(-16.6681788248613,-9.99913246376521,6.6785196366098));
#9836=CARTESIAN_POINT('Ctrl Pts',(-16.6684949259027,-9.94921615609046,6.67516937498693));
#9837=CARTESIAN_POINT('Ctrl Pts',(-16.6664486628489,-9.89932612429603,6.67181911336406));
#9838=CARTESIAN_POINT('Ctrl Pts',(-16.6619555807564,-9.84965743684369,6.66846885174119));
#9839=CARTESIAN_POINT('Ctrl Pts',(-16.612271271896,-9.30042322360766,6.63142180256485));
#9840=CARTESIAN_POINT('Ctrl Pts',(-16.2633938106262,-8.77825464556249,6.59437475338851));
#9841=CARTESIAN_POINT('Ctrl Pts',(-15.7749977417139,-8.5221375949982,6.55732770421217));
#9842=CARTESIAN_POINT('Ctrl Pts',(-15.2866016728016,-8.26602054443391,6.52028065503583));
#9843=CARTESIAN_POINT('Ctrl Pts',(-14.6586869962468,-8.27595502135049,6.48323360585949));
#9844=CARTESIAN_POINT('Ctrl Pts',(-14.1786377296675,-8.54739438937554,6.44618655668315));
#9845=CARTESIAN_POINT('Ctrl Pts',(-13.6985884630883,-8.8188337574006,6.40913950750681));
#9846=CARTESIAN_POINT('Ctrl Pts',(-13.3664046064846,-9.35177801653412,6.37209245833047));
#9847=CARTESIAN_POINT('Ctrl Pts',(-13.3341202049555,-9.90230902307224,6.33504540915413));
#9848=CARTESIAN_POINT('Ctrl Pts',(-13.3018358034264,-10.4528400296104,6.29799835997779));
#9849=CARTESIAN_POINT('Ctrl Pts',(-13.5694508569717,-11.0209577835531,6.26095131080145));
#9850=CARTESIAN_POINT('Ctrl Pts',(-14.0144832145534,-11.3466460666222,6.22390426162511));
#9851=CARTESIAN_POINT('Ctrl Pts',(-14.4595155721351,-11.6723343496913,6.18685721244877));
#9852=CARTESIAN_POINT('Ctrl Pts',(-15.0819652337531,-11.7555931618868,6.14981016327243));
#9853=CARTESIAN_POINT('Ctrl Pts',(-15.5969493099184,-11.5583165663653,6.11276311409609));
#9854=CARTESIAN_POINT('Ctrl Pts',(-16.1119333860836,-11.3610399708438,6.07571606491975));
#9855=CARTESIAN_POINT('Ctrl Pts',(-16.5194518767962,-10.8832279676053,6.03866901574341));
#9856=CARTESIAN_POINT('Ctrl Pts',(-16.6329916163336,-10.3435656777544,6.00162196656707));
#9857=CARTESIAN_POINT('Ctrl Pts',(-16.6565925290862,-10.2313888956821,5.99392118991465));
#9858=CARTESIAN_POINT('Ctrl Pts',(-16.6674912767693,-10.116539700903,5.98622041326222));
#9859=CARTESIAN_POINT('Ctrl Pts',(-16.6664295714326,-10.0014906689886,5.9785196366098));
#9860=CARTESIAN_POINT('Ctrl Pts',(-16.6633787344493,-10.0004304228837,6.17148036339021));
#9861=CARTESIAN_POINT('Ctrl Pts',(-16.6639602176958,-10.2518936021923,6.18823412210537));
#9862=CARTESIAN_POINT('Ctrl Pts',(-16.610516809841,-10.5031221558014,6.20498788082052));
#9863=CARTESIAN_POINT('Ctrl Pts',(-16.5017821786186,-10.7275639185705,6.22174163953568));
#9864=CARTESIAN_POINT('Ctrl Pts',(-16.2613407768679,-11.2238647883572,6.25878868871202));
#9865=CARTESIAN_POINT('Ctrl Pts',(-15.7505415588973,-11.5891861313041,6.29583573788836));
#9866=CARTESIAN_POINT('Ctrl Pts',(-15.2031672337665,-11.6563278030662,6.3328827870647));
#9867=CARTESIAN_POINT('Ctrl Pts',(-14.6557929086356,-11.7234694748282,6.36992983624104));
#9868=CARTESIAN_POINT('Ctrl Pts',(-14.0718434763445,-11.4924314754053,6.40697688541738));
#9869=CARTESIAN_POINT('Ctrl Pts',(-13.7185810400186,-11.0689549177826,6.44402393459372));
#9870=CARTESIAN_POINT('Ctrl Pts',(-13.3653186036927,-10.64547836016,6.48107098377006));
#9871=CARTESIAN_POINT('Ctrl Pts',(-13.242743163332,-10.0295632443375,6.5181180329464));
#9872=CARTESIAN_POINT('Ctrl Pts',(-13.4069550915532,-9.50310254240692,6.55516508212274));
#9873=CARTESIAN_POINT('Ctrl Pts',(-13.5711670197744,-8.97664184047631,6.59221213129908));
#9874=CARTESIAN_POINT('Ctrl Pts',(-14.0221663165775,-8.53963555243749,6.62925918047543));
#9875=CARTESIAN_POINT('Ctrl Pts',(-14.5535394869087,-8.392091269177,6.66630622965176));
#9876=CARTESIAN_POINT('Ctrl Pts',(-15.0849126572399,-8.24454698591652,6.7033532788281));
#9877=CARTESIAN_POINT('Ctrl Pts',(-15.6966597010992,-8.38646470743436,6.74040032800444));
#9878=CARTESIAN_POINT('Ctrl Pts',(-16.1087961519145,-8.75289449913704,6.77744737718078));
#9879=CARTESIAN_POINT('Ctrl Pts',(-16.4574916805962,-9.06291907883561,6.80879170591726));
#9880=CARTESIAN_POINT('Ctrl Pts',(-16.663299692646,-9.53365643270811,6.84013603465374));
#9881=CARTESIAN_POINT('Ctrl Pts',(-16.6673099838652,-10.001299617498,6.87148036339021));
#9882=CARTESIAN_POINT('Origin',(-15.,-10.,4.));
#9883=CARTESIAN_POINT('',(-16.6674570171079,-9.99879340680734,7.57148036339021));
#9884=CARTESIAN_POINT('',(-16.6638186297495,-9.99906044123799,7.37851963660979));
#9885=CARTESIAN_POINT('',(-16.666,-10.,4.));
#9886=CARTESIAN_POINT('',(-13.7309291201476,-8.9206413469515,8.));
#9887=CARTESIAN_POINT('Ctrl Pts',(-16.6674570171079,-9.99879340680734,7.57148036339021));
#9888=CARTESIAN_POINT('Ctrl Pts',(-16.6635089329096,-10.471496226622,7.60317909473112));
#9889=CARTESIAN_POINT('Ctrl Pts',(-16.4524517931744,-10.947171006763,7.63487782607203));
#9890=CARTESIAN_POINT('Ctrl Pts',(-16.0968414251746,-11.2574592188118,7.66657655741294));
#9891=CARTESIAN_POINT('Ctrl Pts',(-15.6812312656001,-11.6201003140335,7.70362360658928));
#9892=CARTESIAN_POINT('Ctrl Pts',(-15.0681737708883,-11.7568375153793,7.74067065576562));
#9893=CARTESIAN_POINT('Ctrl Pts',(-14.5382154198475,-11.6038879901502,7.77771770494196));
#9894=CARTESIAN_POINT('Ctrl Pts',(-14.0082570688068,-11.4509384649211,7.8147647541183));
#9895=CARTESIAN_POINT('Ctrl Pts',(-13.5613978614371,-11.0083022131172,7.85181180329464));
#9896=CARTESIAN_POINT('Ctrl Pts',(-13.402335136949,-10.4812300903389,7.88885885247098));
#9897=CARTESIAN_POINT('Ctrl Pts',(-13.2432724124609,-9.95415796756067,7.92590590164732));
#9898=CARTESIAN_POINT('Ctrl Pts',(-13.3720061708544,-9.34264997380806,7.96295295082366));
#9899=CARTESIAN_POINT('Ctrl Pts',(-13.7309291201476,-8.92064134695149,8.));
#9900=CARTESIAN_POINT('',(-16.,-8.66750009380863,8.));
#9901=CARTESIAN_POINT('Origin',(-15.,-10.,8.));
#9902=CARTESIAN_POINT('',(-16.2714530003192,-8.91876393899414,8.));
#9903=CARTESIAN_POINT('Origin',(-15.,-10.,8.));
#9904=CARTESIAN_POINT('Ctrl Pts',(-16.2714538290145,-8.91876328587891,8.));
#9905=CARTESIAN_POINT('Ctrl Pts',(-15.9205596240576,-8.50717209253843,7.96367382485347));
#9906=CARTESIAN_POINT('Ctrl Pts',(-15.3505268241097,-8.28122091268906,7.92734764970694));
#9907=CARTESIAN_POINT('Ctrl Pts',(-14.8130932124341,-8.34188937586933,7.89102147456041));
#9908=CARTESIAN_POINT('Ctrl Pts',(-14.2649945105902,-8.40376177310978,7.85397442538407));
#9909=CARTESIAN_POINT('Ctrl Pts',(-13.7508016625205,-8.76374232028908,7.81692737620773));
#9910=CARTESIAN_POINT('Ctrl Pts',(-13.5055195900293,-9.25757781397449,7.77988032703139));
#9911=CARTESIAN_POINT('Ctrl Pts',(-13.2602375175381,-9.75141330765989,7.74283327785505));
#9912=CARTESIAN_POINT('Ctrl Pts',(-13.2838662206256,-10.3791037478514,7.70578622867871));
#9913=CARTESIAN_POINT('Ctrl Pts',(-13.5657615293288,-10.8531100236876,7.66873917950237));
#9914=CARTESIAN_POINT('Ctrl Pts',(-13.8476568380319,-11.3271162995237,7.63169213032602));
#9915=CARTESIAN_POINT('Ctrl Pts',(-14.3878187523508,-11.6474384110046,7.59464508114969));
#9916=CARTESIAN_POINT('Ctrl Pts',(-14.9389380738973,-11.6676039864443,7.55759803197335));
#9917=CARTESIAN_POINT('Ctrl Pts',(-15.4900573954438,-11.6877695618841,7.52055098279701));
#9918=CARTESIAN_POINT('Ctrl Pts',(-16.052134124218,-11.4077786012828,7.48350393362067));
#9919=CARTESIAN_POINT('Ctrl Pts',(-16.3679621297839,-10.9557089721593,7.44645688444433));
#9920=CARTESIAN_POINT('Ctrl Pts',(-16.5610183107237,-10.6793723757226,7.42381113516615));
#9921=CARTESIAN_POINT('Ctrl Pts',(-16.6620634106456,-10.3387384131736,7.40116538588797));
#9922=CARTESIAN_POINT('Ctrl Pts',(-16.6638186297495,-9.99906044123799,7.37851963660979));
#9923=CARTESIAN_POINT('Origin',(15.,-10.,4.));
#9924=CARTESIAN_POINT('',(13.332808903179,-9.99865075154404,0.571480363390208));
#9925=CARTESIAN_POINT('',(13.3364072036082,-9.99933549113491,0.378519636609792));
#9926=CARTESIAN_POINT('',(13.334,-10.,4.));
#9927=CARTESIAN_POINT('',(16.6117095221421,-10.4218393251423,0.));
#9928=CARTESIAN_POINT('Ctrl Pts',(13.3364072036082,-9.99933549113491,0.378519636609792));
#9929=CARTESIAN_POINT('Ctrl Pts',(13.335429121529,-9.77385612213223,0.363487571935548));
#9930=CARTESIAN_POINT('Ctrl Pts',(13.378096681235,-9.54871085704481,0.348455507261303));
#9931=CARTESIAN_POINT('Ctrl Pts',(13.4661893677241,-9.34297029044533,0.333423442587059));
#9932=CARTESIAN_POINT('Ctrl Pts',(13.6832968748538,-8.83591546773436,0.296376393410719));
#9933=CARTESIAN_POINT('Ctrl Pts',(14.1763135429627,-8.44672347685267,0.25932934423438));
#9934=CARTESIAN_POINT('Ctrl Pts',(14.7201521567332,-8.35458602338615,0.222282295058041));
#9935=CARTESIAN_POINT('Ctrl Pts',(15.2639907705037,-8.26244856991963,0.185235245881701));
#9936=CARTESIAN_POINT('Ctrl Pts',(15.8586513299358,-8.46736565386832,0.14818819670536));
#9937=CARTESIAN_POINT('Ctrl Pts',(16.2306499484275,-8.87322647615437,0.111141147529019));
#9938=CARTESIAN_POINT('Ctrl Pts',(16.6026485669192,-9.27908729844041,0.0740940983526795));
#9939=CARTESIAN_POINT('Ctrl Pts',(16.7519852444706,-9.88589185906381,0.0370470491763399));
#9940=CARTESIAN_POINT('Ctrl Pts',(16.6117095221421,-10.4218393251423,0.));
#9941=CARTESIAN_POINT('',(14.324922814325,-11.5230977622533,0.));
#9942=CARTESIAN_POINT('Origin',(15.,-10.,0.));
#9943=CARTESIAN_POINT('Ctrl Pts',(14.3235906297078,-11.5258236994894,2.84494650060196E-15));
#9944=CARTESIAN_POINT('Ctrl Pts',(14.818318071977,-11.7444072143423,0.0363261751465322));
#9945=CARTESIAN_POINT('Ctrl Pts',(15.4299365508059,-11.700654408249,0.0726523502930616));
#9946=CARTESIAN_POINT('Ctrl Pts',(15.8878244848826,-11.4128103339302,0.108978525439591));
#9947=CARTESIAN_POINT('Ctrl Pts',(16.354798966577,-11.1192541438444,0.146025574615931));
#9948=CARTESIAN_POINT('Ctrl Pts',(16.6618809586961,-10.5718228333455,0.18307262379227));
#9949=CARTESIAN_POINT('Ctrl Pts',(16.6686052646603,-10.0204684891763,0.22011967296861));
#9950=CARTESIAN_POINT('Ctrl Pts',(16.6753295706245,-9.46911414500705,0.257166722144951));
#9951=CARTESIAN_POINT('Ctrl Pts',(16.3816961904339,-8.91383676716756,0.294213771321292));
#9952=CARTESIAN_POINT('Ctrl Pts',(15.922053673819,-8.60908166657342,0.331260820497633));
#9953=CARTESIAN_POINT('Ctrl Pts',(15.4624111572042,-8.30432656597928,0.368307869673972));
#9954=CARTESIAN_POINT('Ctrl Pts',(14.8367595041652,-8.25009374263046,0.405354918850311));
#9955=CARTESIAN_POINT('Ctrl Pts',(14.3314686216281,-8.47104689559278,0.44240196802665));
#9956=CARTESIAN_POINT('Ctrl Pts',(13.826177739091,-8.69200004855511,0.47944901720299));
#9957=CARTESIAN_POINT('Ctrl Pts',(13.441247627056,-9.18813917782859,0.51649606637933));
#9958=CARTESIAN_POINT('Ctrl Pts',(13.3528420869761,-9.73247249456812,0.55354311555567));
#9959=CARTESIAN_POINT('Ctrl Pts',(13.3385741752475,-9.8203233205136,0.559522198167183));
#9960=CARTESIAN_POINT('Ctrl Pts',(13.332029912926,-9.90942947246795,0.565501280778695));
#9961=CARTESIAN_POINT('Ctrl Pts',(13.332808903179,-9.99865075154404,0.571480363390208));
#9962=CARTESIAN_POINT('Origin',(15.,-10.,4.));
#9963=CARTESIAN_POINT('',(13.3366507554646,-9.99963522356343,1.27148036339021));
#9964=CARTESIAN_POINT('',(13.3350094287786,-10.0014379681814,1.07851963660979));
#9965=CARTESIAN_POINT('',(13.334,-10.,4.));
#9966=CARTESIAN_POINT('Ctrl Pts',(13.3350094287786,-10.0014379681814,1.07851963660979));
#9967=CARTESIAN_POINT('Ctrl Pts',(13.3382278453089,-9.61090143175114,1.05243653366026));
#9968=CARTESIAN_POINT('Ctrl Pts',(13.4753924362828,-9.21832997108139,1.02635343071072));
#9969=CARTESIAN_POINT('Ctrl Pts',(13.7262226675361,-8.92195568147024,1.00027032776118));
#9970=CARTESIAN_POINT('Ctrl Pts',(14.0824885585281,-8.5010014375266,0.963223278584839));
#9971=CARTESIAN_POINT('Ctrl Pts',(14.6680617783195,-8.27411389904732,0.926176229408499));
#9972=CARTESIAN_POINT('Ctrl Pts',(15.2149469785867,-8.34515454403535,0.889129180232159));
#9973=CARTESIAN_POINT('Ctrl Pts',(15.761832178854,-8.41619518902339,0.852082131055819));
#9974=CARTESIAN_POINT('Ctrl Pts',(16.270029359597,-8.78516401747873,0.815035081879478));
#9975=CARTESIAN_POINT('Ctrl Pts',(16.5069274603671,-9.28315343747998,0.777988032703138));
#9976=CARTESIAN_POINT('Ctrl Pts',(16.7438255611371,-9.78114285748121,0.740940983526799));
#9977=CARTESIAN_POINT('Ctrl Pts',(16.7094245819342,-10.4081528690283,0.703893934350459));
#9978=CARTESIAN_POINT('Ctrl Pts',(16.4195064837655,-10.8772867275589,0.66684688517412));
#9979=CARTESIAN_POINT('Ctrl Pts',(16.1295883855967,-11.3464205860894,0.629799835997779));
#9980=CARTESIAN_POINT('Ctrl Pts',(15.584153168462,-11.6576782916034,0.592752786821439));
#9981=CARTESIAN_POINT('Ctrl Pts',(15.0327634293889,-11.6684612152136,0.555705737645099));
#9982=CARTESIAN_POINT('Ctrl Pts',(14.4813736903159,-11.6792441388238,0.518658688468759));
#9983=CARTESIAN_POINT('Ctrl Pts',(13.9240294293046,-11.3895522805303,0.481611639292419));
#9984=CARTESIAN_POINT('Ctrl Pts',(13.6159564718742,-10.9322475241134,0.444564590116079));
#9985=CARTESIAN_POINT('Ctrl Pts',(13.4328859835592,-10.6604969434577,0.422549605613984));
#9986=CARTESIAN_POINT('Ctrl Pts',(13.3378396390242,-10.3295579137833,0.400534621111888));
#9987=CARTESIAN_POINT('Ctrl Pts',(13.3364072036082,-9.99933549113491,0.378519636609792));
#9988=CARTESIAN_POINT('Ctrl Pts',(13.332808903179,-9.99865075154404,0.571480363390208));
#9989=CARTESIAN_POINT('Ctrl Pts',(13.3368566216514,-10.4622542665498,0.602548329955035));
#9990=CARTESIAN_POINT('Ctrl Pts',(13.5386288752517,-10.9289661622094,0.633616296519862));
#9991=CARTESIAN_POINT('Ctrl Pts',(13.8819529433812,-11.2388249495348,0.664684263084689));
#9992=CARTESIAN_POINT('Ctrl Pts',(14.2913503079907,-11.6083165835564,0.701731312261029));
#9993=CARTESIAN_POINT('Ctrl Pts',(14.9020260053343,-11.7547723473939,0.73877836143737));
#9994=CARTESIAN_POINT('Ctrl Pts',(15.4344828856238,-11.6111839655915,0.77582541061371));
#9995=CARTESIAN_POINT('Ctrl Pts',(15.9669397659133,-11.4675955837891,0.81287245979005));
#9996=CARTESIAN_POINT('Ctrl Pts',(16.4211778291486,-11.0339630563467,0.849919508966388));
#9997=CARTESIAN_POINT('Ctrl Pts',(16.5893028175547,-10.5087402588661,0.886966558142728));
#9998=CARTESIAN_POINT('Ctrl Pts',(16.7574278059609,-9.98351746138546,0.924013607319068));
#9999=CARTESIAN_POINT('Ctrl Pts',(16.6394397195377,-9.36670439386655,0.961060656495409));
#10000=CARTESIAN_POINT('Ctrl Pts',(16.2893385866089,-8.94060996175609,0.99810770567175));
#10001=CARTESIAN_POINT('Ctrl Pts',(15.93923745368,-8.51451552964562,1.03515475484809));
#10002=CARTESIAN_POINT('Ctrl Pts',(15.3570232742455,-8.27913973294359,1.07220180402443));
#10003=CARTESIAN_POINT('Ctrl Pts',(14.8091643748095,-8.34220645059644,1.10924885320077));
#10004=CARTESIAN_POINT('Ctrl Pts',(14.2613054753736,-8.4052731682493,1.14629590237711));
#10005=CARTESIAN_POINT('Ctrl Pts',(13.7478018559363,-8.76678240025705,1.18334295155345));
#10006=CARTESIAN_POINT('Ctrl Pts',(13.5036737629058,-9.26128004979684,1.22039000072979));
#10007=CARTESIAN_POINT('Ctrl Pts',(13.3914507646209,-9.48859517845444,1.2374201216166));
#10008=CARTESIAN_POINT('Ctrl Pts',(13.3361505793704,-9.74401261814188,1.2544502425034));
#10009=CARTESIAN_POINT('Ctrl Pts',(13.3366507554646,-9.99963522356343,1.27148036339021));
#10010=CARTESIAN_POINT('Origin',(15.,-10.,4.));
#10011=CARTESIAN_POINT('',(13.3341441093425,-10.001523795318,1.97148036339021));
#10012=CARTESIAN_POINT('',(13.3312584258872,-9.99997573739076,1.7785196366098));
#10013=CARTESIAN_POINT('',(13.334,-10.,4.));
#10014=CARTESIAN_POINT('Ctrl Pts',(13.3312589065494,-9.99997574164457,1.7785196366098));
#10015=CARTESIAN_POINT('Ctrl Pts',(13.3311402696763,-9.44720220187264,1.74138549538496));
#10016=CARTESIAN_POINT('Ctrl Pts',(13.633172680189,-8.89454120416279,1.70425135416013));
#10017=CARTESIAN_POINT('Ctrl Pts',(14.0982990508631,-8.595851335138,1.6671172129353));
#10018=CARTESIAN_POINT('Ctrl Pts',(14.5623345437871,-8.29786199429832,1.63007016375896));
#10019=CARTESIAN_POINT('Ctrl Pts',(15.1886983610305,-8.25265388018618,1.59302311458262));
#10020=CARTESIAN_POINT('Ctrl Pts',(15.6907163532175,-8.48091822226867,1.55597606540628));
#10021=CARTESIAN_POINT('Ctrl Pts',(16.1927343454045,-8.70918256435115,1.51892901622994));
#10022=CARTESIAN_POINT('Ctrl Pts',(16.5704065125352,-9.21091936262827,1.4818819670536));
#10023=CARTESIAN_POINT('Ctrl Pts',(16.6508794054907,-9.75649288727719,1.44483491787726));
#10024=CARTESIAN_POINT('Ctrl Pts',(16.7313522984462,-10.3020664119261,1.40778786870092));
#10025=CARTESIAN_POINT('Ctrl Pts',(16.5146259172266,-10.8914766629468,1.37074081952458));
#10026=CARTESIAN_POINT('Ctrl Pts',(16.0998923475637,-11.2549636062132,1.33369377034824));
#10027=CARTESIAN_POINT('Ctrl Pts',(15.6851587779009,-11.6184505494795,1.2966467211719));
#10028=CARTESIAN_POINT('Ctrl Pts',(15.072418019795,-11.7560141849915,1.25959967199556));
#10029=CARTESIAN_POINT('Ctrl Pts',(14.5421080391536,-11.6046916700352,1.22255262281922));
#10030=CARTESIAN_POINT('Ctrl Pts',(14.0117980585123,-11.453369155079,1.18550557364288));
#10031=CARTESIAN_POINT('Ctrl Pts',(13.5639188553357,-11.0131604896544,1.14845852446654));
#10032=CARTESIAN_POINT('Ctrl Pts',(13.4034585348436,-10.4855456822382,1.1114114752902));
#10033=CARTESIAN_POINT('Ctrl Pts',(13.3559708572951,-10.3293999025988,1.1004475290634));
#10034=CARTESIAN_POINT('Ctrl Pts',(13.3336565780138,-10.165598712143,1.08948358283659));
#10035=CARTESIAN_POINT('Ctrl Pts',(13.3350094287786,-10.0014379681814,1.07851963660979));
#10036=CARTESIAN_POINT('Ctrl Pts',(13.3366507554646,-9.99963522356343,1.27148036339021));
#10037=CARTESIAN_POINT('Ctrl Pts',(13.3372386543453,-10.3000898941977,1.29149729167974));
#10038=CARTESIAN_POINT('Ctrl Pts',(13.4149162640182,-10.6008280068514,1.31151421996928));
#10039=CARTESIAN_POINT('Ctrl Pts',(13.5678609198539,-10.8565494916407,1.33153114825881));
#10040=CARTESIAN_POINT('Ctrl Pts',(13.8509287364562,-11.3298352168729,1.36857819743515));
#10041=CARTESIAN_POINT('Ctrl Pts',(14.3918169362847,-11.6489206002655,1.40562524661149));
#10042=CARTESIAN_POINT('Ctrl Pts',(14.9429716267943,-11.6677669773384,1.44267229578783));
#10043=CARTESIAN_POINT('Ctrl Pts',(15.4941263173039,-11.6866133544114,1.47971934496417));
#10044=CARTESIAN_POINT('Ctrl Pts',(16.0555474984946,-11.4052207251646,1.51676639414051));
#10045=CARTESIAN_POINT('Ctrl Pts',(16.3702838225975,-10.9523767230522,1.55381344331685));
#10046=CARTESIAN_POINT('Ctrl Pts',(16.6850201467003,-10.4995327209398,1.59086049249319));
#10047=CARTESIAN_POINT('Ctrl Pts',(16.7530716137152,-9.87523734596178,1.62790754166953));
#10048=CARTESIAN_POINT('Ctrl Pts',(16.5432923975969,-9.36521835878357,1.66495459084587));
#10049=CARTESIAN_POINT('Ctrl Pts',(16.3335131814787,-8.85519937160537,1.70200164002221));
#10050=CARTESIAN_POINT('Ctrl Pts',(15.8459032822273,-8.45945677222701,1.73904868919855));
#10051=CARTESIAN_POINT('Ctrl Pts',(15.3036321193532,-8.3591140693806,1.77609573837489));
#10052=CARTESIAN_POINT('Ctrl Pts',(14.761360956479,-8.25877136653418,1.81314278755123));
#10053=CARTESIAN_POINT('Ctrl Pts',(14.1644285299821,-8.45382856021971,1.85018983672757));
#10054=CARTESIAN_POINT('Ctrl Pts',(13.7860390074197,-8.85501185765043,1.88723688590391));
#10055=CARTESIAN_POINT('Ctrl Pts',(13.4992248982105,-9.15910333804621,1.91531804506601));
#10056=CARTESIAN_POINT('Ctrl Pts',(13.3379731658201,-9.58162320501827,1.94339920422811));
#10057=CARTESIAN_POINT('Ctrl Pts',(13.3341441093425,-10.001523795318,1.97148036339021));
#10058=CARTESIAN_POINT('Origin',(15.,-10.,4.));
#10059=CARTESIAN_POINT('',(13.3314909130637,-9.99943625433425,2.67148036339021));
#10060=CARTESIAN_POINT('',(13.3350798878256,-9.99857774548763,2.47851963660979));
#10061=CARTESIAN_POINT('',(13.334,-10.,4.));
#10062=CARTESIAN_POINT('Ctrl Pts',(13.3350798878256,-9.99857774548763,2.47851963660979));
#10063=CARTESIAN_POINT('Ctrl Pts',(13.3337247030062,-9.83179020445009,2.46738150628601));
#10064=CARTESIAN_POINT('Ctrl Pts',(13.3567684529751,-9.66536860128073,2.45624337596222));
#10065=CARTESIAN_POINT('Ctrl Pts',(13.4057542707778,-9.50696974162459,2.44510524563843));
#10066=CARTESIAN_POINT('Ctrl Pts',(13.5686882595461,-8.98011198609755,2.40805819646209));
#10067=CARTESIAN_POINT('Ctrl Pts',(14.0186257820356,-8.54201183282465,2.37101114728576));
#10068=CARTESIAN_POINT('Ctrl Pts',(14.5496393266922,-8.39317905803324,2.33396409810942));
#10069=CARTESIAN_POINT('Ctrl Pts',(15.0806528713488,-8.24434628324183,2.29691704893308));
#10070=CARTESIAN_POINT('Ctrl Pts',(15.6927424381725,-8.38478088693191,2.25986999975674));
#10071=CARTESIAN_POINT('Ctrl Pts',(16.1057667357084,-8.75020873407366,2.2228229505804));
#10072=CARTESIAN_POINT('Ctrl Pts',(16.5187910332443,-9.11563658121541,2.18577590140406));
#10073=CARTESIAN_POINT('Ctrl Pts',(16.7327500614925,-9.70605767180883,2.14872885222772));
#10074=CARTESIAN_POINT('Ctrl Pts',(16.6497189958645,-10.2512479305517,2.11168180305138));
#10075=CARTESIAN_POINT('Ctrl Pts',(16.5666879302365,-10.7964381892946,2.07463475387504));
#10076=CARTESIAN_POINT('Ctrl Pts',(16.1866667707325,-11.296397616187,2.0375877046987));
#10077=CARTESIAN_POINT('Ctrl Pts',(15.6835837031669,-11.5223046908978,2.00054065552236));
#10078=CARTESIAN_POINT('Ctrl Pts',(15.1805006356014,-11.7482117656085,1.96349360634602));
#10079=CARTESIAN_POINT('Ctrl Pts',(14.5543556599743,-11.7000664881376,1.92644655716968));
#10080=CARTESIAN_POINT('Ctrl Pts',(14.0917229282246,-11.3999039494764,1.88939950799334));
#10081=CARTESIAN_POINT('Ctrl Pts',(13.630177776544,-11.100447047862,1.85243955086549));
#10082=CARTESIAN_POINT('Ctrl Pts',(13.3313769869357,-10.550156401746,1.81547959373764));
#10083=CARTESIAN_POINT('Ctrl Pts',(13.3312589065494,-9.99997574164457,1.7785196366098));
#10084=CARTESIAN_POINT('Ctrl Pts',(13.3341441093425,-10.001523795318,1.97148036339021));
#10085=CARTESIAN_POINT('Ctrl Pts',(13.332921549439,-10.1355917120949,1.98044625340445));
#10086=CARTESIAN_POINT('Ctrl Pts',(13.3477471050693,-10.2693926123545,1.98941214341869));
#10087=CARTESIAN_POINT('Ctrl Pts',(13.3796577910855,-10.3989865385901,1.99837803343293));
#10088=CARTESIAN_POINT('Ctrl Pts',(13.5115127159413,-10.9344685209231,2.03542508260927));
#10089=CARTESIAN_POINT('Ctrl Pts',(13.9350691842808,-11.3981230844133,2.07247213178561));
#10090=CARTESIAN_POINT('Ctrl Pts',(14.4564737723188,-11.5777447085202,2.10951918096195));
#10091=CARTESIAN_POINT('Ctrl Pts',(14.9778783603568,-11.757366332627,2.14656623013829));
#10092=CARTESIAN_POINT('Ctrl Pts',(15.5971310680934,-11.6529550173506,2.18361327931463));
#10093=CARTESIAN_POINT('Ctrl Pts',(16.0308121730685,-11.312297753733,2.22066032849097));
#10094=CARTESIAN_POINT('Ctrl Pts',(16.4644932780436,-10.9716404901154,2.25770737766731));
#10095=CARTESIAN_POINT('Ctrl Pts',(16.7126027802573,-10.3947372781565,2.29475442684365));
#10096=CARTESIAN_POINT('Ctrl Pts',(16.661585864872,-9.84562531584823,2.33180147601999));
#10097=CARTESIAN_POINT('Ctrl Pts',(16.6105689494867,-9.29651335353996,2.36884852519633));
#10098=CARTESIAN_POINT('Ctrl Pts',(16.2604256165023,-8.7751926408823,2.40589557437267));
#10099=CARTESIAN_POINT('Ctrl Pts',(15.7714095479698,-8.52026136158418,2.44294262354901));
#10100=CARTESIAN_POINT('Ctrl Pts',(15.2823934794373,-8.26533008228607,2.47998967272535));
#10101=CARTESIAN_POINT('Ctrl Pts',(14.6545046753566,-8.2767882363475,2.51703672190169));
#10102=CARTESIAN_POINT('Ctrl Pts',(14.1751154292343,-8.54939165370295,2.55408377107803));
#10103=CARTESIAN_POINT('Ctrl Pts',(13.6957261831121,-8.8219950710584,2.59113082025437));
#10104=CARTESIAN_POINT('Ctrl Pts',(13.3648364949483,-9.35574375170787,2.62817786943071));
#10105=CARTESIAN_POINT('Ctrl Pts',(13.3338880340578,-9.90635147533067,2.66522491860705));
#10106=CARTESIAN_POINT('Ctrl Pts',(13.3321461374468,-9.93734176370615,2.6673100668681));
#10107=CARTESIAN_POINT('Ctrl Pts',(13.3313544140885,-9.96838545925023,2.66939521512916));
#10108=CARTESIAN_POINT('Ctrl Pts',(13.3314909130637,-9.99943625433425,2.67148036339021));
#10109=CARTESIAN_POINT('Origin',(15.,-10.,4.));
#10110=CARTESIAN_POINT('',(13.335810245754,-9.99883056901517,3.37148036339021));
#10111=CARTESIAN_POINT('',(13.336290211156,-10.0008527825146,3.17851963660979));
#10112=CARTESIAN_POINT('',(13.334,-10.,4.));
#10113=CARTESIAN_POINT('Ctrl Pts',(13.336290211156,-10.0008527825146,3.17851963660979));
#10114=CARTESIAN_POINT('Ctrl Pts',(13.3378338117211,-9.66797335838089,3.15633046801071));
#10115=CARTESIAN_POINT('Ctrl Pts',(13.4345606860051,-9.33426795934119,3.13414129941163));
#10116=CARTESIAN_POINT('Ctrl Pts',(13.6203848998586,-9.06119200316891,3.11195213081255));
#10117=CARTESIAN_POINT('Ctrl Pts',(13.9306371185501,-8.60526422326959,3.07490508163621));
#10118=CARTESIAN_POINT('Ctrl Pts',(14.4892540658804,-8.31834502654515,3.03785803245988));
#10119=CARTESIAN_POINT('Ctrl Pts',(15.0405678077089,-8.33175165747664,3.00081098328354));
#10120=CARTESIAN_POINT('Ctrl Pts',(15.5918815495374,-8.34515828840813,2.9637639341072));
#10121=CARTESIAN_POINT('Ctrl Pts',(16.1358920858641,-8.65889074699554,2.92671688493086));
#10122=CARTESIAN_POINT('Ctrl Pts',(16.4236165482283,-9.12935988890904,2.88966983575452));
#10123=CARTESIAN_POINT('Ctrl Pts',(16.7113410105926,-9.59982903082254,2.85262278657817));
#10124=CARTESIAN_POINT('Ctrl Pts',(16.7427793989944,-10.2270348560621,2.81557573740184));
#10125=CARTESIAN_POINT('Ctrl Pts',(16.5035429844033,-10.7239176567056,2.77852868822549));
#10126=CARTESIAN_POINT('Ctrl Pts',(16.2643065698122,-11.220800457349,2.74148163904916));
#10127=CARTESIAN_POINT('Ctrl Pts',(15.7543953522281,-11.5873602333962,2.70443458987282));
#10128=CARTESIAN_POINT('Ctrl Pts',(15.2071856163145,-11.6558298219649,2.66738754069648));
#10129=CARTESIAN_POINT('Ctrl Pts',(14.6599758804009,-11.7242994105336,2.63034049152014));
#10130=CARTESIAN_POINT('Ctrl Pts',(14.0754676261578,-11.4946788116238,2.5932934423438));
#10131=CARTESIAN_POINT('Ctrl Pts',(13.7211787265599,-11.0720608332783,2.55624639316746));
#10132=CARTESIAN_POINT('Ctrl Pts',(13.4734061629112,-10.7765022085018,2.5303374743149));
#10133=CARTESIAN_POINT('Ctrl Pts',(13.3382322457616,-10.3865499401683,2.50442855546235));
#10134=CARTESIAN_POINT('Ctrl Pts',(13.3350798878256,-9.99857774548763,2.47851963660979));
#10135=CARTESIAN_POINT('Ctrl Pts',(13.3314909130637,-9.99943625433425,2.67148036339021));
#10136=CARTESIAN_POINT('Ctrl Pts',(13.3337796057835,-10.5200682119484,2.7064422643055));
#10137=CARTESIAN_POINT('Ctrl Pts',(13.5970248523073,-11.0426961045957,2.74140416522078));
#10138=CARTESIAN_POINT('Ctrl Pts',(14.0177536614366,-11.3490334538225,2.77636606613607));
#10139=CARTESIAN_POINT('Ctrl Pts',(14.4635749833231,-11.6736409420954,2.81341311531241));
#10140=CARTESIAN_POINT('Ctrl Pts',(15.0862248607134,-11.755389152045,2.85046016448875));
#10141=CARTESIAN_POINT('Ctrl Pts',(15.60072875322,-11.5568635438935,2.88750721366509));
#10142=CARTESIAN_POINT('Ctrl Pts',(16.1152326457267,-11.3583379357421,2.92455426284143));
#10143=CARTESIAN_POINT('Ctrl Pts',(16.5215905533498,-10.8795385094896,2.96160131201776));
#10144=CARTESIAN_POINT('Ctrl Pts',(16.6338204946098,-10.3396022977084,2.99864836119411));
#10145=CARTESIAN_POINT('Ctrl Pts',(16.7460504358698,-9.79966608592732,3.03569541037045));
#10146=CARTESIAN_POINT('Ctrl Pts',(16.5641524107667,-9.19859308861758,3.07274245954679));
#10147=CARTESIAN_POINT('Ctrl Pts',(16.1713775496498,-8.81148253467369,3.10978950872313));
#10148=CARTESIAN_POINT('Ctrl Pts',(15.778602688533,-8.42437198072981,3.14683655789947));
#10149=CARTESIAN_POINT('Ctrl Pts',(15.1749509914024,-8.25122387015177,3.18388360707581));
#10150=CARTESIAN_POINT('Ctrl Pts',(14.6367019071036,-8.37128467038591,3.22093065625215));
#10151=CARTESIAN_POINT('Ctrl Pts',(14.0984528228048,-8.49134547062004,3.25797770542849));
#10152=CARTESIAN_POINT('Ctrl Pts',(13.6256063513377,-8.90461518166635,3.29502475460483));
#10153=CARTESIAN_POINT('Ctrl Pts',(13.4345749755091,-9.42194842625029,3.33207180378117));
#10154=CARTESIAN_POINT('Ctrl Pts',(13.366838844212,-9.60538506029802,3.34520799031751));
#10155=CARTESIAN_POINT('Ctrl Pts',(13.3345347092875,-9.80190537509914,3.35834417685386));
#10156=CARTESIAN_POINT('Ctrl Pts',(13.335810245754,-9.99883056901517,3.37148036339021));
#10157=CARTESIAN_POINT('Origin',(15.,-10.,4.));
#10158=CARTESIAN_POINT('',(13.3357192381005,-10.0012124487014,4.07148036339021));
#10159=CARTESIAN_POINT('',(13.3319678875119,-10.0009660455274,3.8785196366098));
#10160=CARTESIAN_POINT('',(13.334,-10.,4.));
#10161=CARTESIAN_POINT('Ctrl Pts',(13.3319678875119,-10.0009660455274,3.8785196366098));
#10162=CARTESIAN_POINT('Ctrl Pts',(13.3353869932426,-9.50559826735267,3.84527942973542));
#10163=CARTESIAN_POINT('Ctrl Pts',(13.5702060950421,-9.00741586198988,3.81203922286105));
#10164=CARTESIAN_POINT('Ctrl Pts',(13.9562882145892,-8.69793856196637,3.77879901598667));
#10165=CARTESIAN_POINT('Ctrl Pts',(14.3865864772631,-8.35301830330904,3.74175196681034));
#10166=CARTESIAN_POINT('Ctrl Pts',(15.0047785911423,-8.2425012022264,3.704704917634));
#10167=CARTESIAN_POINT('Ctrl Pts',(15.527930246067,-8.41696875119106,3.66765786845766));
#10168=CARTESIAN_POINT('Ctrl Pts',(16.0510819009917,-8.59143630015572,3.63061081928132));
#10169=CARTESIAN_POINT('Ctrl Pts',(16.4791930969619,-9.05088849916767,3.59356377010497));
#10170=CARTESIAN_POINT('Ctrl Pts',(16.616325802445,-9.58504315914936,3.55651672092863));
#10171=CARTESIAN_POINT('Ctrl Pts',(16.7534585079282,-10.1191978191311,3.51946967175229));
#10172=CARTESIAN_POINT('Ctrl Pts',(16.5996127229243,-10.7280549400825,3.48242262257596));
#10173=CARTESIAN_POINT('Ctrl Pts',(16.2252006220181,-11.1329526535695,3.44537557339962));
#10174=CARTESIAN_POINT('Ctrl Pts',(15.850788521112,-11.5378503670565,3.40832852422328));
#10175=CARTESIAN_POINT('Ctrl Pts',(15.2558101043037,-11.7387886730791,3.37128147504693));
#10176=CARTESIAN_POINT('Ctrl Pts',(14.712575231494,-11.6438020811096,3.33423442587059));
#10177=CARTESIAN_POINT('Ctrl Pts',(14.1693403586842,-11.54881548914,3.29718737669425));
#10178=CARTESIAN_POINT('Ctrl Pts',(13.6778490298729,-11.1579039991783,3.26014032751792));
#10179=CARTESIAN_POINT('Ctrl Pts',(13.4630471104936,-10.6499800726604,3.22309327834158));
#10180=CARTESIAN_POINT('Ctrl Pts',(13.3768998643064,-10.4462749676569,3.20823539776431));
#10181=CARTESIAN_POINT('Ctrl Pts',(13.3352566152936,-10.2237490441893,3.19337751718705));
#10182=CARTESIAN_POINT('Ctrl Pts',(13.336290211156,-10.0008527825146,3.17851963660979));
#10183=CARTESIAN_POINT('Ctrl Pts',(13.335810245754,-9.99883056901517,3.37148036339021));
#10184=CARTESIAN_POINT('Ctrl Pts',(13.3381320137313,-10.3572794422137,3.3953912260302));
#10185=CARTESIAN_POINT('Ctrl Pts',(13.4517110307273,-10.717069773939,3.41930208867019));
#10186=CARTESIAN_POINT('Ctrl Pts',(13.6653762209856,-11.0017377389844,3.44321295131018));
#10187=CARTESIAN_POINT('Ctrl Pts',(13.9964251224806,-11.442797029013,3.48026000048652));
#10188=CARTESIAN_POINT('Ctrl Pts',(14.5677392056608,-11.7035188309486,3.51730704966286));
#10189=CARTESIAN_POINT('Ctrl Pts',(15.1178393083377,-11.6645759299679,3.55435409883921));
#10190=CARTESIAN_POINT('Ctrl Pts',(15.6679394110145,-11.6256330289872,3.59140114801555));
#10191=CARTESIAN_POINT('Ctrl Pts',(16.196825533188,-11.2870254250901,3.62844819719189));
#10192=CARTESIAN_POINT('Ctrl Pts',(16.4624369517103,-10.8037271250179,3.66549524636823));
#10193=CARTESIAN_POINT('Ctrl Pts',(16.7280483702325,-10.3204288249458,3.70254229554457));
#10194=CARTESIAN_POINT('Ctrl Pts',(16.7303850851034,-9.69243982869853,3.73958934472091));
#10195=CARTESIAN_POINT('Ctrl Pts',(16.4683776281186,-9.20717828583092,3.77663639389725));
#10196=CARTESIAN_POINT('Ctrl Pts',(16.2063701711338,-8.72191674296332,3.81368344307359));
#10197=CARTESIAN_POINT('Ctrl Pts',(15.6800185422933,-8.37938265347533,3.85073049224993));
#10198=CARTESIAN_POINT('Ctrl Pts',(15.1302234772481,-8.33634709894435,3.88777754142627));
#10199=CARTESIAN_POINT('Ctrl Pts',(14.5804284122028,-8.29331154441336,3.92482459060261));
#10200=CARTESIAN_POINT('Ctrl Pts',(14.0071899109527,-8.54977452483937,3.96187163977895));
#10201=CARTESIAN_POINT('Ctrl Pts',(13.6728679037955,-8.98835800381711,3.99891868895529));
#10202=CARTESIAN_POINT('Ctrl Pts',(13.4545962269312,-9.2746997622177,4.02310591376693));
#10203=CARTESIAN_POINT('Ctrl Pts',(13.338162810448,-9.63867046299276,4.04729313857857));
#10204=CARTESIAN_POINT('Ctrl Pts',(13.3357192381005,-10.0012124487014,4.07148036339021));
#10205=CARTESIAN_POINT('Origin',(15.,-10.,4.));
#10206=CARTESIAN_POINT('',(13.3314357387427,-10.0004924312937,4.77148036339021));
#10207=CARTESIAN_POINT('',(13.3333641526241,-9.99853839723902,4.5785196366098));
#10208=CARTESIAN_POINT('',(13.334,-10.,4.));
#10209=CARTESIAN_POINT('Ctrl Pts',(13.3333641526241,-9.99853839723902,4.5785196366098));
#10210=CARTESIAN_POINT('Ctrl Pts',(13.3323717813096,-9.89034515242106,4.57127544063647));
#10211=CARTESIAN_POINT('Ctrl Pts',(13.3420055133055,-9.78232785263767,4.56403124466314));
#10212=CARTESIAN_POINT('Ctrl Pts',(13.3629080587333,-9.67653708828116,4.55678704868981));
#10213=CARTESIAN_POINT('Ctrl Pts',(13.4698043424929,-9.13551974640515,4.51973999951347));
#10214=CARTESIAN_POINT('Ctrl Pts',(13.8714175336596,-8.6527337027222,4.48269295033713));
#10215=CARTESIAN_POINT('Ctrl Pts',(14.3839372136889,-8.44914058575823,4.44564590116079));
#10216=CARTESIAN_POINT('Ctrl Pts',(14.8964568937183,-8.24554746879426,4.40859885198445));
#10217=CARTESIAN_POINT('Ctrl Pts',(15.5198830626101,-8.32114727854928,4.37155180280811));
#10218=CARTESIAN_POINT('Ctrl Pts',(15.9688858866921,-8.64133947654767,4.33450475363177));
#10219=CARTESIAN_POINT('Ctrl Pts',(16.417888710774,-8.96153167454607,4.29745770445543));
#10220=CARTESIAN_POINT('Ctrl Pts',(16.692468190046,-9.52631626078785,4.26041065527909));
#10221=CARTESIAN_POINT('Ctrl Pts',(16.6669547247066,-10.0772024947589,4.22336360610275));
#10222=CARTESIAN_POINT('Ctrl Pts',(16.6414412593673,-10.62808872873,4.18631655692641));
#10223=CARTESIAN_POINT('Ctrl Pts',(16.3158348494168,-11.1650766104304,4.14926950775008));
#10224=CARTESIAN_POINT('Ctrl Pts',(15.8391591121324,-11.4423974015313,4.11222245857374));
#10225=CARTESIAN_POINT('Ctrl Pts',(15.362483374848,-11.7197181926323,4.0751754093974));
#10226=CARTESIAN_POINT('Ctrl Pts',(14.7347383102298,-11.7373718931338,4.03812836022106));
#10227=CARTESIAN_POINT('Ctrl Pts',(14.2432304251484,-11.4872787532933,4.00108131104471));
#10228=CARTESIAN_POINT('Ctrl Pts',(13.751722540067,-11.2371856134528,3.96403426186837));
#10229=CARTESIAN_POINT('Ctrl Pts',(13.3964518345225,-10.7193456332703,3.92698721269203));
#10230=CARTESIAN_POINT('Ctrl Pts',(13.3400186874845,-10.170763935063,3.88994016351569));
#10231=CARTESIAN_POINT('Ctrl Pts',(13.3342197886207,-10.1143933451982,3.88613332121373));
#10232=CARTESIAN_POINT('Ctrl Pts',(13.3315763136454,-10.0576981537274,3.88232647891176));
#10233=CARTESIAN_POINT('Ctrl Pts',(13.3319678875119,-10.0009660455274,3.8785196366098));
#10234=CARTESIAN_POINT('Ctrl Pts',(13.3357192381005,-10.0012124487014,4.07148036339021));
#10235=CARTESIAN_POINT('Ctrl Pts',(13.3344200435276,-10.1939681822487,4.08434018775491));
#10236=CARTESIAN_POINT('Ctrl Pts',(13.3653437139473,-10.3863200439156,4.09720001211961));
#10237=CARTESIAN_POINT('Ctrl Pts',(13.4303165819644,-10.5663859959084,4.1100598364843));
#10238=CARTESIAN_POINT('Ctrl Pts',(13.6174927803551,-11.0851265314924,4.14710688566065));
#10239=CARTESIAN_POINT('Ctrl Pts',(14.0872506902009,-11.501903625131,4.18415393483699));
#10240=CARTESIAN_POINT('Ctrl Pts',(14.6245914022956,-11.6259666398754,4.22120098401333));
#10241=CARTESIAN_POINT('Ctrl Pts',(15.1619321143903,-11.7500296546197,4.25824803318967));
#10242=CARTESIAN_POINT('Ctrl Pts',(15.7668556287338,-11.5813785904697,4.295295082366));
#10243=CARTESIAN_POINT('Ctrl Pts',(16.162500410882,-11.19720170561,4.33234213154234));
#10244=CARTESIAN_POINT('Ctrl Pts',(16.5581451930302,-10.8130248207503,4.36938918071868));
#10245=CARTESIAN_POINT('Ctrl Pts',(16.7445112429831,-10.2133221151808,4.40643622989503));
#10246=CARTESIAN_POINT('Ctrl Pts',(16.6363025037439,-9.67256566237146,4.44348327907137));
#10247=CARTESIAN_POINT('Ctrl Pts',(16.5280937645046,-9.13180920956211,4.4805303282477));
#10248=CARTESIAN_POINT('Ctrl Pts',(16.1253102360732,-8.64999900951287,4.51757737742404));
#10249=CARTESIAN_POINT('Ctrl Pts',(15.6122979772257,-8.44765006641306,4.55462442660038));
#10250=CARTESIAN_POINT('Ctrl Pts',(15.0992857183783,-8.24530112331325,4.59167147577672));
#10251=CARTESIAN_POINT('Ctrl Pts',(14.4760447291148,-8.32241343716287,4.62871852495306));
#10252=CARTESIAN_POINT('Ctrl Pts',(14.0278200900524,-8.64369422625152,4.6657655741294));
#10253=CARTESIAN_POINT('Ctrl Pts',(13.6014795823874,-8.94928879376472,4.70100383721634));
#10254=CARTESIAN_POINT('Ctrl Pts',(13.3334826207238,-9.47579130585967,4.73624210030328));
#10255=CARTESIAN_POINT('Ctrl Pts',(13.3314357387427,-10.0004924312937,4.77148036339021));
#10256=CARTESIAN_POINT('Origin',(15.,-10.,4.));
#10257=CARTESIAN_POINT('',(13.3342680725317,-9.99847819315956,5.47148036339021));
#10258=CARTESIAN_POINT('',(13.3367226502574,-9.99994375235263,5.2785196366098));
#10259=CARTESIAN_POINT('',(13.334,-10.,4.));
#10260=CARTESIAN_POINT('Ctrl Pts',(13.3367226502574,-9.99994375235263,5.2785196366098));
#10261=CARTESIAN_POINT('Ctrl Pts',(13.3366399476421,-9.72530236931467,5.26022440236118));
#10262=CARTESIAN_POINT('Ctrl Pts',(13.4008958576234,-9.45069741139684,5.24192916811256));
#10263=CARTESIAN_POINT('Ctrl Pts',(13.5297031735473,-9.21074369088521,5.22363393386393));
#10264=CARTESIAN_POINT('Ctrl Pts',(13.7905323546587,-8.72484790168481,5.18658688468759));
#10265=CARTESIAN_POINT('Ctrl Pts',(14.3160512106056,-8.38103770500959,5.14953983551125));
#10266=CARTESIAN_POINT('Ctrl Pts',(14.8657401494705,-8.33666823153406,5.11249278633491));
#10267=CARTESIAN_POINT('Ctrl Pts',(15.4154290883355,-8.29229875805853,5.07544573715857));
#10268=CARTESIAN_POINT('Ctrl Pts',(15.9892881101184,-8.54737000778269,5.03839868798223));
#10269=CARTESIAN_POINT('Ctrl Pts',(16.3246732845184,-8.98514091189926,5.00135163880589));
#10270=CARTESIAN_POINT('Ctrl Pts',(16.6600584589185,-9.42291181601583,4.96430458962955));
#10271=CARTESIAN_POINT('Ctrl Pts',(16.7569697859359,-10.0433823745248,4.92725754045321));
#10272=CARTESIAN_POINT('Ctrl Pts',(16.5710528669398,-10.5625754782171,4.89021049127687));
#10273=CARTESIAN_POINT('Ctrl Pts',(16.3851359479437,-11.0817685819094,4.85316344210053));
#10274=CARTESIAN_POINT('Ctrl Pts',(15.9163907829341,-11.499684230785,4.81611639292419));
#10275=CARTESIAN_POINT('Ctrl Pts',(15.3793527678201,-11.6250506936619,4.77906934374785));
#10276=CARTESIAN_POINT('Ctrl Pts',(14.842314752706,-11.7504171565388,4.74202229457151));
#10277=CARTESIAN_POINT('Ctrl Pts',(14.2369838874874,-11.5832344334171,4.70497524539517));
#10278=CARTESIAN_POINT('Ctrl Pts',(13.8404081430543,-11.2000187518216,4.66792819621883));
#10279=CARTESIAN_POINT('Ctrl Pts',(13.52137899072,-10.8917372298759,4.63812534301582));
#10280=CARTESIAN_POINT('Ctrl Pts',(13.3374467998521,-10.4436488559758,4.60832248981281));
#10281=CARTESIAN_POINT('Ctrl Pts',(13.3333641526241,-9.99853839723902,4.5785196366098));
#10282=CARTESIAN_POINT('Ctrl Pts',(13.3314357387427,-10.0004924312937,4.77148036339021));
#10283=CARTESIAN_POINT('Ctrl Pts',(13.3313306719395,-10.0274254300751,4.77328914947962));
#10284=CARTESIAN_POINT('Ctrl Pts',(13.3319263268189,-10.0543536825872,4.77509793556902));
#10285=CARTESIAN_POINT('Ctrl Pts',(13.3332372565238,-10.0812470687196,4.77690672165842));
#10286=CARTESIAN_POINT('Ctrl Pts',(13.3600873509191,-10.6320698577713,4.81395377083476));
#10287=CARTESIAN_POINT('Ctrl Pts',(13.6869958285712,-11.1682661715471,4.8510008200111));
#10288=CARTESIAN_POINT('Ctrl Pts',(14.1643431415556,-11.444429556671,4.88804786918744));
#10289=CARTESIAN_POINT('Ctrl Pts',(14.6416904545399,-11.7205929417949,4.92509491836378));
#10290=CARTESIAN_POINT('Ctrl Pts',(15.2694766028563,-11.7367233982669,4.96214196754013));
#10291=CARTESIAN_POINT('Ctrl Pts',(15.7603762764363,-11.4854383351005,4.99918901671647));
#10292=CARTESIAN_POINT('Ctrl Pts',(16.2512759500163,-11.2341532719342,5.0362360658928));
#10293=CARTESIAN_POINT('Ctrl Pts',(16.6052891488598,-10.7154526891295,5.07328311506914));
#10294=CARTESIAN_POINT('Ctrl Pts',(16.6603910299587,-10.1667355896657,5.11033016424548));
#10295=CARTESIAN_POINT('Ctrl Pts',(16.7154929110576,-9.61801849020194,5.14737721342182));
#10296=CARTESIAN_POINT('Ctrl Pts',(16.4716834744118,-9.03928487407907,5.18442426259816));
#10297=CARTESIAN_POINT('Ctrl Pts',(16.0405494795664,-8.69540967732856,5.2214713117745));
#10298=CARTESIAN_POINT('Ctrl Pts',(15.6094154847211,-8.35153448057806,5.25851836095084));
#10299=CARTESIAN_POINT('Ctrl Pts',(14.9909569316761,-8.24251770319993,5.29556541012718));
#10300=CARTESIAN_POINT('Ctrl Pts',(14.468230074541,-8.41825416861712,5.33261245930352));
#10301=CARTESIAN_POINT('Ctrl Pts',(13.945503217406,-8.59399063403432,5.36965950847986));
#10302=CARTESIAN_POINT('Ctrl Pts',(13.518508056181,-9.05448034224686,5.40670655765621));
#10303=CARTESIAN_POINT('Ctrl Pts',(13.3826718353368,-9.58896625778836,5.44375360683255));
#10304=CARTESIAN_POINT('Ctrl Pts',(13.3487843156306,-9.72230626005756,5.45299585901843));
#10305=CARTESIAN_POINT('Ctrl Pts',(13.3330176438504,-9.86025156147491,5.46223811120432));
#10306=CARTESIAN_POINT('Ctrl Pts',(13.3342680725317,-9.99847819315956,5.47148036339021));
#10307=CARTESIAN_POINT('Origin',(15.,-10.,4.));
#10308=CARTESIAN_POINT('',(13.3366212029652,-10.0004304228509,6.17148036339021));
#10309=CARTESIAN_POINT('',(13.33357064153,-10.0014906687784,5.9785196366098));
#10310=CARTESIAN_POINT('',(13.334,-10.,4.));
#10311=CARTESIAN_POINT('Ctrl Pts',(13.33357064153,-10.0014906687784,5.9785196366098));
#10312=CARTESIAN_POINT('Ctrl Pts',(13.3376166087855,-9.56305959032262,5.94917336408589));
#10313=CARTESIAN_POINT('Ctrl Pts',(13.5153564139545,-9.12172640784843,5.91982709156197));
#10314=CARTESIAN_POINT('Ctrl Pts',(13.8257421956427,-8.81432850902488,5.89048081903805));
#10315=CARTESIAN_POINT('Ctrl Pts',(14.2175765353692,-8.42626610467219,5.85343376986171));
#10316=CARTESIAN_POINT('Ctrl Pts',(14.8208062262297,-8.25165379552422,5.81638672068537));
#10317=CARTESIAN_POINT('Ctrl Pts',(15.3593449655314,-8.37040818713264,5.77933967150903));
#10318=CARTESIAN_POINT('Ctrl Pts',(15.8978837048331,-8.48916257874107,5.74229262233269));
#10319=CARTESIAN_POINT('Ctrl Pts',(16.371731492576,-8.90128367110589,5.70524557315635));
#10320=CARTESIAN_POINT('Ctrl Pts',(16.5640175621394,-9.41815178528104,5.66819852398002));
#10321=CARTESIAN_POINT('Ctrl Pts',(16.7563036317028,-9.93501989945619,5.63115147480367));
#10322=CARTESIAN_POINT('Ctrl Pts',(16.6670279830868,-10.5566350354417,5.59410442562733));
#10323=CARTESIAN_POINT('Ctrl Pts',(16.3370503164634,-10.9984962344251,5.55705737645099));
#10324=CARTESIAN_POINT('Ctrl Pts',(16.0070726498399,-11.4403574334086,5.52001032727465));
#10325=CARTESIAN_POINT('Ctrl Pts',(15.436392965209,-11.7024646953901,5.48296327809831));
#10326=CARTESIAN_POINT('Ctrl Pts',(14.886200072778,-11.6648567074084,5.44591622892197));
#10327=CARTESIAN_POINT('Ctrl Pts',(14.336007180347,-11.6272487194266,5.40886917974563));
#10328=CARTESIAN_POINT('Ctrl Pts',(13.8063010801158,-11.2899254814817,5.37182213056929));
#10329=CARTESIAN_POINT('Ctrl Pts',(13.5395177831381,-10.8072731716464,5.33477508139295));
#10330=CARTESIAN_POINT('Ctrl Pts',(13.4044821697233,-10.5629728295224,5.31602326646523));
#10331=CARTESIAN_POINT('Ctrl Pts',(13.336807416821,-10.2814391579995,5.29727145153752));
#10332=CARTESIAN_POINT('Ctrl Pts',(13.3367226502574,-9.99994375235263,5.2785196366098));
#10333=CARTESIAN_POINT('Ctrl Pts',(13.3342680725317,-9.99847819315956,5.47148036339021));
#10334=CARTESIAN_POINT('Ctrl Pts',(13.3380299170405,-10.4143252567718,5.49928516038066));
#10335=CARTESIAN_POINT('Ctrl Pts',(13.4958090207374,-10.8327185659559,5.52708995737111));
#10336=CARTESIAN_POINT('Ctrl Pts',(13.7775518556619,-11.135922385114,5.55489475436156));
#10337=CARTESIAN_POINT('Ctrl Pts',(14.1529453772945,-11.5399104740277,5.5919418035379));
#10338=CARTESIAN_POINT('Ctrl Pts',(14.7484097010232,-11.7394045289846,5.62898885271425));
#10339=CARTESIAN_POINT('Ctrl Pts',(15.291412576878,-11.6431000686136,5.66603590189058));
#10340=CARTESIAN_POINT('Ctrl Pts',(15.8344154527327,-11.5467956082426,5.70308295106692));
#10341=CARTESIAN_POINT('Ctrl Pts',(16.3249568807135,-11.1546926325437,5.74013000024326));
#10342=CARTESIAN_POINT('Ctrl Pts',(16.5385257463691,-10.6462489146804,5.7771770494196));
#10343=CARTESIAN_POINT('Ctrl Pts',(16.7520946120246,-10.1378051968171,5.81422409859594));
#10344=CARTESIAN_POINT('Ctrl Pts',(16.688690915355,-9.51302073678948,5.85127114777228));
#10345=CARTESIAN_POINT('Ctrl Pts',(16.3773332746596,-9.05784704631197,5.88831819694862));
#10346=CARTESIAN_POINT('Ctrl Pts',(16.0659756339641,-8.60267335583447,5.92536524612496));
#10347=CARTESIAN_POINT('Ctrl Pts',(15.5066640492429,-8.31711043490708,5.9624122953013));
#10348=CARTESIAN_POINT('Ctrl Pts',(14.9553843770011,-8.33185475830429,5.99945934447764));
#10349=CARTESIAN_POINT('Ctrl Pts',(14.4041047047594,-8.34659908170151,6.03650639365398));
#10350=CARTESIAN_POINT('Ctrl Pts',(13.8608569449971,-8.66165064942335,6.07355344283032));
#10351=CARTESIAN_POINT('Ctrl Pts',(13.5742748573298,-9.13281664334238,6.11060049200666));
#10352=CARTESIAN_POINT('Ctrl Pts',(13.4172935679881,-9.39090760018266,6.13089378246785));
#10353=CARTESIAN_POINT('Ctrl Pts',(13.3373255349887,-9.69584112940636,6.15118707292903));
#10354=CARTESIAN_POINT('Ctrl Pts',(13.3366212029652,-10.0004304228509,6.17148036339021));
#10355=CARTESIAN_POINT('Origin',(15.,-10.,4.));
#10356=CARTESIAN_POINT('',(13.3326899541194,-10.0012996150481,6.87148036339021));
#10357=CARTESIAN_POINT('',(13.331821388128,-9.99913246339926,6.6785196366098));
#10358=CARTESIAN_POINT('',(13.334,-10.,4.));
#10359=CARTESIAN_POINT('Ctrl Pts',(13.331821388128,-9.99913246339926,6.6785196366098));
#10360=CARTESIAN_POINT('Ctrl Pts',(13.3315052870993,-9.9492161620323,6.67516937498693));
#10361=CARTESIAN_POINT('Ctrl Pts',(13.3335515498683,-9.89932613655299,6.67181911336406));
#10362=CARTESIAN_POINT('Ctrl Pts',(13.338044631369,-9.84965745540188,6.66846885174119));
#10363=CARTESIAN_POINT('Ctrl Pts',(13.3877289336859,-9.30042331184456,6.63142180256485));
#10364=CARTESIAN_POINT('Ctrl Pts',(13.7366063508799,-8.77825480177775,6.59437475338851));
#10365=CARTESIAN_POINT('Ctrl Pts',(14.225002357486,-8.52213778422821,6.55732770421217));
#10366=CARTESIAN_POINT('Ctrl Pts',(14.7133983640921,-8.26602076667867,6.52028065503583));
#10367=CARTESIAN_POINT('Ctrl Pts',(15.3413129601104,-8.2759552416464,6.48323360585949));
#10368=CARTESIAN_POINT('Ctrl Pts',(15.8213621652753,-8.54739457482633,6.44618655668316));
#10369=CARTESIAN_POINT('Ctrl Pts',(16.3014113704402,-8.81883390800626,6.40913950750682));
#10370=CARTESIAN_POINT('Ctrl Pts',(16.6335951847516,-9.35177809939841,6.37209245833047));
#10371=CARTESIAN_POINT('Ctrl Pts',(16.6658795821906,-9.90230903566246,6.33504540915413));
#10372=CARTESIAN_POINT('Ctrl Pts',(16.6981639796295,-10.4528399719265,6.29799835997779));
#10373=CARTESIAN_POINT('Ctrl Pts',(16.4305489601959,-11.0209576530625,6.26095131080145));
#10374=CARTESIAN_POINT('Ctrl Pts',(15.9855166594699,-11.3466458944622,6.22390426162511));
#10375=CARTESIAN_POINT('Ctrl Pts',(15.5404843587439,-11.672334135862,6.18685721244877));
#10376=CARTESIAN_POINT('Ctrl Pts',(14.9180347767255,-11.7555929375255,6.14981016327243));
#10377=CARTESIAN_POINT('Ctrl Pts',(14.403050766387,-11.5583163672411,6.11276311409609));
#10378=CARTESIAN_POINT('Ctrl Pts',(13.8880667560485,-11.3610397969568,6.07571606491975));
#10379=CARTESIAN_POINT('Ctrl Pts',(13.48054831739,-10.8832278547246,6.03866901574341));
#10380=CARTESIAN_POINT('Ctrl Pts',(13.3670085923569,-10.3435656338298,6.00162196656707));
#10381=CARTESIAN_POINT('Ctrl Pts',(13.3434076826193,-10.231388866091,5.99392118991465));
#10382=CARTESIAN_POINT('Ctrl Pts',(13.3325089363286,-10.1165396859889,5.98622041326223));
#10383=CARTESIAN_POINT('Ctrl Pts',(13.33357064153,-10.0014906687784,5.9785196366098));
#10384=CARTESIAN_POINT('Ctrl Pts',(13.3366212029652,-10.0004304228509,6.17148036339021));
#10385=CARTESIAN_POINT('Ctrl Pts',(13.336039719701,-10.2518936116005,6.18823412210537));
#10386=CARTESIAN_POINT('Ctrl Pts',(13.389483129569,-10.503122174652,6.20498788082052));
#10387=CARTESIAN_POINT('Ctrl Pts',(13.4982177648784,-10.7275639458888,6.22174163953568));
#10388=CARTESIAN_POINT('Ctrl Pts',(13.7386591756668,-11.2238648344,6.25878868871202));
#10389=CARTESIAN_POINT('Ctrl Pts',(14.2494584128161,-11.5891861913062,6.29583573788837));
#10390=CARTESIAN_POINT('Ctrl Pts',(14.7968327585657,-11.6563278655082,6.33288278706471));
#10391=CARTESIAN_POINT('Ctrl Pts',(15.3442071043154,-11.7234695397102,6.36992983624105));
#10392=CARTESIAN_POINT('Ctrl Pts',(15.9281565586655,-11.4924315312079,6.40697688541738));
#10393=CARTESIAN_POINT('Ctrl Pts',(16.2814190082463,-11.0689549578054,6.44402393459372));
#10394=CARTESIAN_POINT('Ctrl Pts',(16.6346814578271,-10.6454783844028,6.48107098377006));
#10395=CARTESIAN_POINT('Ctrl Pts',(16.7572569026387,-10.0295632461,6.5181180329464));
#10396=CARTESIAN_POINT('Ctrl Pts',(16.5930449683129,-9.50310252407789,6.55516508212274));
#10397=CARTESIAN_POINT('Ctrl Pts',(16.4288330339871,-8.97664180205576,6.59221213129908));
#10398=CARTESIAN_POINT('Ctrl Pts',(15.9778337205239,-8.53963549631433,6.62925918047542));
#10399=CARTESIAN_POINT('Ctrl Pts',(15.4464605300519,-8.39209120799975,6.66630622965176));
#10400=CARTESIAN_POINT('Ctrl Pts',(14.9150873395799,-8.24454691968518,6.7033532788281));
#10401=CARTESIAN_POINT('Ctrl Pts',(14.303340272099,-8.38646464879746,6.74040032800445));
#10402=CARTESIAN_POINT('Ctrl Pts',(13.8912038060524,-8.75289445340972,6.77744737718078));
#10403=CARTESIAN_POINT('Ctrl Pts',(13.5425082644839,-9.06291904403068,6.80879170591726));
#10404=CARTESIAN_POINT('Ctrl Pts',(13.3367002455534,-9.53365641263032,6.84013603465373));
#10405=CARTESIAN_POINT('Ctrl Pts',(13.3326899541194,-10.0012996150481,6.87148036339021));
#10406=CARTESIAN_POINT('Origin',(15.,-10.,4.));
#10407=CARTESIAN_POINT('',(13.3325429336747,-9.99879337075124,7.57148036339021));
#10408=CARTESIAN_POINT('',(13.3361815844527,-9.99906045492932,7.3785196366098));
#10409=CARTESIAN_POINT('',(13.334,-10.,4.));
#10410=CARTESIAN_POINT('',(16.2690708798524,-8.9206413469515,8.));
#10411=CARTESIAN_POINT('Ctrl Pts',(13.3325429336747,-9.99879337075124,7.57148036339021));
#10412=CARTESIAN_POINT('Ctrl Pts',(13.3364909776232,-10.4714962597792,7.60317909473112));
#10413=CARTESIAN_POINT('Ctrl Pts',(13.5475480484014,-10.9471711688739,7.63487782607203));
#10414=CARTESIAN_POINT('Ctrl Pts',(13.9031584757476,-11.2574593537338,7.66657655741294));
#10415=CARTESIAN_POINT('Ctrl Pts',(14.3187687046815,-11.6201004171794,7.70362360658928));
#10416=CARTESIAN_POINT('Ctrl Pts',(14.931826444004,-11.7568373734716,7.74067065576562));
#10417=CARTESIAN_POINT('Ctrl Pts',(15.4617847126295,-11.603887923119,7.77771770494196));
#10418=CARTESIAN_POINT('Ctrl Pts',(15.9917429812551,-11.4509384727664,7.8147647541183));
#10419=CARTESIAN_POINT('Ctrl Pts',(16.4386017791837,-11.008302615769,7.85181180329464));
#10420=CARTESIAN_POINT('Ctrl Pts',(16.5976644911563,-10.4812304910294,7.88885885247098));
#10421=CARTESIAN_POINT('Ctrl Pts',(16.756727203129,-9.95415836628982,7.92590590164732));
#10422=CARTESIAN_POINT('Ctrl Pts',(16.6279938291456,-9.34264997380806,7.96295295082366));
#10423=CARTESIAN_POINT('Ctrl Pts',(16.2690708798524,-8.92064134695149,8.));
#10424=CARTESIAN_POINT('',(16.,-8.66750009380863,8.));
#10425=CARTESIAN_POINT('Origin',(15.,-10.,8.));
#10426=CARTESIAN_POINT('',(13.7285472376402,-8.91876346821723,8.));
#10427=CARTESIAN_POINT('Origin',(15.,-10.,8.));
#10428=CARTESIAN_POINT('Ctrl Pts',(13.7285464165792,-8.9187628208919,8.));
#10429=CARTESIAN_POINT('Ctrl Pts',(14.0794406943795,-8.50717132356286,7.96367382485347));
#10430=CARTESIAN_POINT('Ctrl Pts',(14.6494732896009,-8.28122126317251,7.92734764970694));
#10431=CARTESIAN_POINT('Ctrl Pts',(15.1869067713614,-8.34188994522698,7.89102147456041));
#10432=CARTESIAN_POINT('Ctrl Pts',(15.735005340712,-8.40376256568508,7.85397442538407));
#10433=CARTESIAN_POINT('Ctrl Pts',(16.2491981340985,-8.76374239939929,7.81692737620773));
#10434=CARTESIAN_POINT('Ctrl Pts',(16.4944801949704,-9.25757769375947,7.77988032703139));
#10435=CARTESIAN_POINT('Ctrl Pts',(16.7397622558424,-9.75141298811966,7.74283327785505));
#10436=CARTESIAN_POINT('Ctrl Pts',(16.7161335841998,-10.3791037431258,7.70578622867871));
#10437=CARTESIAN_POINT('Ctrl Pts',(16.4342383093536,-10.8531100403582,7.66873917950237));
#10438=CARTESIAN_POINT('Ctrl Pts',(16.1523430345073,-11.3271163375905,7.63169213032603));
#10439=CARTESIAN_POINT('Ctrl Pts',(15.6121811564573,-11.6474381770491,7.59464508114969));
#10440=CARTESIAN_POINT('Ctrl Pts',(15.0610619021163,-11.6676037010972,7.55759803197335));
#10441=CARTESIAN_POINT('Ctrl Pts',(14.5099426477752,-11.6877692251453,7.52055098279701));
#10442=CARTESIAN_POINT('Ctrl Pts',(13.9478660171431,-11.407778433783,7.48350393362067));
#10443=CARTESIAN_POINT('Ctrl Pts',(13.6320380558773,-10.9557088910527,7.44645688444433));
#10444=CARTESIAN_POINT('Ctrl Pts',(13.4389819020169,-10.6793723474257,7.42381113516615));
#10445=CARTESIAN_POINT('Ctrl Pts',(13.3379368090562,-10.3387384067309,7.40116538588797));
#10446=CARTESIAN_POINT('Ctrl Pts',(13.3361815844527,-9.99906045492932,7.3785196366098));
#10447=CARTESIAN_POINT('Origin',(15.,-10.,9.54592528053767));
#10448=CARTESIAN_POINT('',(12.9482189085318,-9.99918043241852,0.154074719462319));
#10449=CARTESIAN_POINT('',(12.9434420405202,-10.0015653531237,0.0959252805376758));
#10450=CARTESIAN_POINT('',(12.94525,-9.99999999999991,9.54592528053767));
#10451=CARTESIAN_POINT('',(13.6609982804014,-8.44145197141315,1.11022302462516E-15));
#10452=CARTESIAN_POINT('Ctrl Pts',(12.9434420405202,-10.0015653531237,0.0959252805376757));
#10453=CARTESIAN_POINT('Ctrl Pts',(12.948189590265,-9.4149504982262,0.0639501870251168));
#10454=CARTESIAN_POINT('Ctrl Pts',(13.2136828890534,-8.82575586659749,0.0319750935125577));
#10455=CARTESIAN_POINT('Ctrl Pts',(13.6609982804014,-8.44145197141313,-1.11022302462516E-15));
#10456=CARTESIAN_POINT('',(14.6157705213662,-7.97768900275326,1.06453246059332E-15));
#10457=CARTESIAN_POINT('Origin',(15.,-10.,0.));
#10458=CARTESIAN_POINT('Ctrl Pts',(12.9482189085318,-9.99918043241852,0.154074719462319));
#10459=CARTESIAN_POINT('Ctrl Pts',(12.947012597516,-9.72108695495263,0.139042654788076));
#10460=CARTESIAN_POINT('Ctrl Pts',(13.1268058099709,-8.77236641039839,0.0876844149673037));
#10461=CARTESIAN_POINT('Ctrl Pts',(13.9605770103796,-8.10301207949468,0.0363261751465313));
#10462=CARTESIAN_POINT('Ctrl Pts',(14.615770327818,-7.97768772784116,8.78610335527941E-16));
#10463=CARTESIAN_POINT('Origin',(15.,-10.,9.54592528053767));
#10464=CARTESIAN_POINT('',(12.9464949722586,-10.0017735084758,0.854074719462319));
#10465=CARTESIAN_POINT('',(12.9437809686717,-9.99833591340643,0.795925280537676));
#10466=CARTESIAN_POINT('',(12.94525,-9.99999999999991,9.54592528053767));
#10467=CARTESIAN_POINT('Ctrl Pts',(12.9437809686717,-9.99833591340643,0.795925280537676));
#10468=CARTESIAN_POINT('Ctrl Pts',(12.9428202062333,-9.88829544330943,0.789946197926164));
#10469=CARTESIAN_POINT('Ctrl Pts',(13.0009023236625,-9.09745398140138,0.746920066138311));
#10470=CARTESIAN_POINT('Ctrl Pts',(14.0270251243106,-7.77487708517042,0.666846885174118));
#10471=CARTESIAN_POINT('Ctrl Pts',(16.3419550176155,-7.97554015919684,0.555705737645099));
#10472=CARTESIAN_POINT('Ctrl Pts',(17.4284073368472,-10.0300831221902,0.444564590116078));
#10473=CARTESIAN_POINT('Ctrl Pts',(16.2921947498604,-12.0555954005474,0.333423442587058));
#10474=CARTESIAN_POINT('Ctrl Pts',(13.9727681426279,-12.2024165492448,0.222282295058038));
#10475=CARTESIAN_POINT('Ctrl Pts',(12.9909165518555,-10.866791374719,0.143116241041578));
#10476=CARTESIAN_POINT('Ctrl Pts',(12.9426889743311,-10.0946154183123,0.100997236201457));
#10477=CARTESIAN_POINT('Ctrl Pts',(12.9434420405202,-10.0015653531237,0.0959252805376757));
#10478=CARTESIAN_POINT('Ctrl Pts',(12.9464949722586,-10.0017735084758,0.854074719462319));
#10479=CARTESIAN_POINT('Ctrl Pts',(12.950464384843,-9.52010787328362,0.827991616512784));
#10480=CARTESIAN_POINT('Ctrl Pts',(13.3599169395246,-8.34823555313923,0.764861464386909));
#10481=CARTESIAN_POINT('Ctrl Pts',(15.3128190350351,-7.59155964248331,0.664684263084691));
#10482=CARTESIAN_POINT('Ctrl Pts',(17.1931638558005,-8.95675538126231,0.553543115555674));
#10483=CARTESIAN_POINT('Ctrl Pts',(17.0658792003075,-11.2767112418142,0.442401968026652));
#10484=CARTESIAN_POINT('Ctrl Pts',(15.0477525273048,-12.4283740936836,0.331260820497633));
#10485=CARTESIAN_POINT('Ctrl Pts',(13.2644774636808,-11.5014779126907,0.235151737642855));
#10486=CARTESIAN_POINT('Ctrl Pts',(12.9499855932083,-10.4064580572305,0.176089703964416));
#10487=CARTESIAN_POINT('Ctrl Pts',(12.9482189085318,-9.99918043241852,0.154074719462319));
#10488=CARTESIAN_POINT('Origin',(15.,-10.,9.54592528053767));
#10489=CARTESIAN_POINT('',(12.9418692906557,-9.99997008111884,1.55407471946232));
#10490=CARTESIAN_POINT('',(12.9485192915911,-9.99955010541237,1.49592528053768));
#10491=CARTESIAN_POINT('',(12.94525,-9.99999999999991,9.54592528053767));
#10492=CARTESIAN_POINT('Ctrl Pts',(12.9485192915911,-9.99955010541237,1.49592528053768));
#10493=CARTESIAN_POINT('Ctrl Pts',(12.9479024027379,-9.68427966814349,1.47889515965087));
#10494=CARTESIAN_POINT('Ctrl Pts',(13.1644766450531,-8.68397852586288,1.42481798958772));
#10495=CARTESIAN_POINT('Ctrl Pts',(14.7222622974566,-7.58728928450919,1.33369377034824));
#10496=CARTESIAN_POINT('Ctrl Pts',(16.8764722347793,-8.45818679640628,1.22255262281922));
#10497=CARTESIAN_POINT('Ctrl Pts',(17.3130316956038,-10.7404136580229,1.1114114752902));
#10498=CARTESIAN_POINT('Ctrl Pts',(15.632337229038,-12.3448670237413,1.00027032776118));
#10499=CARTESIAN_POINT('Ctrl Pts',(13.4943745863678,-11.8321285059805,0.89510826284367));
#10500=CARTESIAN_POINT('Ctrl Pts',(12.948773195281,-10.5701182198038,0.826993247102503));
#10501=CARTESIAN_POINT('Ctrl Pts',(12.9437809686717,-9.99833591340643,0.795925280537676));
#10502=CARTESIAN_POINT('Ctrl Pts',(12.9418692906557,-9.99997008111884,1.55407471946232));
#10503=CARTESIAN_POINT('Ctrl Pts',(12.9418689474861,-9.99837112568582,1.55398762741383));
#10504=CARTESIAN_POINT('Ctrl Pts',(12.9425947611461,-9.31661188450496,1.516853486189));
#10505=CARTESIAN_POINT('Ctrl Pts',(13.6876865848533,-7.95643655777695,1.44267229578783));
#10506=CARTESIAN_POINT('Ctrl Pts',(16.0052515070878,-7.78916517877589,1.33153114825881));
#10507=CARTESIAN_POINT('Ctrl Pts',(17.4026498601701,-9.64560639052843,1.22039000072979));
#10508=CARTESIAN_POINT('Ctrl Pts',(16.6007557452642,-11.8264420086883,1.10924885320077));
#10509=CARTESIAN_POINT('Ctrl Pts',(14.3335965506935,-12.3354315886432,0.998107705671752));
#10510=CARTESIAN_POINT('Ctrl Pts',(13.0653413219675,-11.0888969478397,0.913049661092266));
#10511=CARTESIAN_POINT('Ctrl Pts',(12.9448264427814,-10.2042400682928,0.865038665689123));
#10512=CARTESIAN_POINT('Ctrl Pts',(12.9464949722586,-10.0017735084758,0.854074719462319));
#10513=CARTESIAN_POINT('Origin',(15.,-10.,9.54592528053767));
#10514=CARTESIAN_POINT('',(12.9465818724548,-9.99824587187305,2.25407471946232));
#10515=CARTESIAN_POINT('',(12.9454277362974,-10.001879362803,2.19592528053768));
#10516=CARTESIAN_POINT('',(12.94525,-9.99999999999991,9.54592528053767));
#10517=CARTESIAN_POINT('Ctrl Pts',(12.9454277362974,-10.001879362803,2.19592528053768));
#10518=CARTESIAN_POINT('Ctrl Pts',(12.9501502775923,-9.48399776741373,2.16784412137558));
#10519=CARTESIAN_POINT('Ctrl Pts',(13.4114067583102,-8.27539043040156,2.10271591303714));
#10520=CARTESIAN_POINT('Ctrl Pts',(15.4418987567046,-7.61189477590683,2.00054065552236));
#10521=CARTESIAN_POINT('Ctrl Pts',(17.2460700180853,-9.07615427063553,1.88939950799333));
#10522=CARTESIAN_POINT('Ctrl Pts',(16.9942775477693,-11.3860658944101,1.77825836046432));
#10523=CARTESIAN_POINT('Ctrl Pts',(14.9170023279882,-12.42722706778,1.6671172129353));
#10524=CARTESIAN_POINT('Ctrl Pts',(13.2223586797308,-11.4275084228001,1.57300618629309));
#10525=CARTESIAN_POINT('Ctrl Pts',(12.9492443727587,-10.3701138716103,1.51594220882721));
#10526=CARTESIAN_POINT('Ctrl Pts',(12.9485192915911,-9.99955010541237,1.49592528053768));
#10527=CARTESIAN_POINT('Ctrl Pts',(12.9465818724548,-9.99824587187305,2.25407471946232));
#10528=CARTESIAN_POINT('Ctrl Pts',(12.9449104642869,-9.79253956938397,2.24293658913854));
#10529=CARTESIAN_POINT('Ctrl Pts',(13.067863238549,-8.90457654972051,2.19475140963841));
#10530=CARTESIAN_POINT('Ctrl Pts',(14.3445560924207,-7.66147210297657,2.10951918096195));
#10531=CARTESIAN_POINT('Ctrl Pts',(16.6093058597035,-8.18108435135386,1.99837803343293));
#10532=CARTESIAN_POINT('Ctrl Pts',(17.4009606855609,-10.3656601062701,1.88723688590391));
#10533=CARTESIAN_POINT('Ctrl Pts',(15.9948709901991,-12.2155249905566,1.77609573837489));
#10534=CARTESIAN_POINT('Ctrl Pts',(13.6799312363543,-12.0375256116339,1.66504168289436));
#10535=CARTESIAN_POINT('Ctrl Pts',(12.9420149243134,-10.6785317325855,1.59103467659017));
#10536=CARTESIAN_POINT('Ctrl Pts',(12.9418692906557,-9.99997008111884,1.55407471946232));
#10537=CARTESIAN_POINT('Origin',(15.,-10.,9.54592528053767));
#10538=CARTESIAN_POINT('',(12.9480746166703,-10.0010517736324,2.95407471946232));
#10539=CARTESIAN_POINT('',(12.9421554343443,-9.9993047080392,2.89592528053767));
#10540=CARTESIAN_POINT('',(12.94525,-9.99999999999991,9.54592528053767));
#10541=CARTESIAN_POINT('Ctrl Pts',(12.9421554343443,-9.9993047080392,2.89592528053768));
#10542=CARTESIAN_POINT('Ctrl Pts',(12.9419870842427,-9.96100841680338,2.89384013227662));
#10543=CARTESIAN_POINT('Ctrl Pts',(12.9603125383811,-9.24246220617618,2.85470793483923));
#10544=CARTESIAN_POINT('Ctrl Pts',(13.7994831701705,-7.88882009045181,2.7785286882255));
#10545=CARTESIAN_POINT('Ctrl Pts',(16.122690589471,-7.84642457654237,2.66738754069648));
#10546=CARTESIAN_POINT('Ctrl Pts',(17.4182314300163,-9.77532685925541,2.55624639316745));
#10547=CARTESIAN_POINT('Ctrl Pts',(16.5002188255622,-11.9098860575253,2.44510524563844));
#10548=CARTESIAN_POINT('Ctrl Pts',(14.2089652219215,-12.2962110576408,2.33396409810941));
#10549=CARTESIAN_POINT('Ctrl Pts',(13.0377585044605,-11.0141261883668,2.2509041097425));
#10550=CARTESIAN_POINT('Ctrl Pts',(12.9439199001859,-10.1672311347101,2.20489117055192));
#10551=CARTESIAN_POINT('Ctrl Pts',(12.9454277362974,-10.001879362803,2.19592528053768));
#10552=CARTESIAN_POINT('Ctrl Pts',(12.9480746166703,-10.0010517736324,2.95407471946232));
#10553=CARTESIAN_POINT('Ctrl Pts',(12.9499784061428,-9.59049715374129,2.93188555086324));
#10554=CARTESIAN_POINT('Ctrl Pts',(13.2684549392389,-8.4917607441522,2.87264933308783));
#10555=CARTESIAN_POINT('Ctrl Pts',(15.0590413951949,-7.57207216315973,2.77636606613607));
#10556=CARTESIAN_POINT('Ctrl Pts',(17.0718967064505,-8.73289167567321,2.66522491860705));
#10557=CARTESIAN_POINT('Ctrl Pts',(17.1882196870663,-11.053572052764,2.55408377107803));
#10558=CARTESIAN_POINT('Ctrl Pts',(15.3015328785473,-12.4098542253325,2.44294262354901));
#10559=CARTESIAN_POINT('Ctrl Pts',(13.3555719234122,-11.6453950124307,2.34293960634377));
#10560=CARTESIAN_POINT('Ctrl Pts',(12.950469812112,-10.4767487932537,2.27998363831488));
#10561=CARTESIAN_POINT('Ctrl Pts',(12.9465818724548,-9.99824587187305,2.25407471946232));
#10562=CARTESIAN_POINT('Origin',(15.,-10.,9.54592528053767));
#10563=CARTESIAN_POINT('',(12.9427437076021,-10.0011914658147,3.65407471946232));
#10564=CARTESIAN_POINT('',(12.9474826545396,-9.9985576900864,3.59592528053768));
#10565=CARTESIAN_POINT('',(12.94525,-9.99999999999991,9.54592528053767));
#10566=CARTESIAN_POINT('Ctrl Pts',(12.9474826545396,-9.9985576900864,3.59592528053768));
#10567=CARTESIAN_POINT('Ctrl Pts',(12.9459094801371,-9.75568131421667,3.58278909400133));
#10568=CARTESIAN_POINT('Ctrl Pts',(13.0981153708669,-8.82974568304574,3.53260585828864));
#10569=CARTESIAN_POINT('Ctrl Pts',(14.4712648408794,-7.62960754320777,3.44537557339961));
#10570=CARTESIAN_POINT('Ctrl Pts',(16.7047942370601,-8.27026074886842,3.3342344258706));
#10571=CARTESIAN_POINT('Ctrl Pts',(17.3778223890662,-10.4942488783201,3.22309327834157));
#10572=CARTESIAN_POINT('Ctrl Pts',(15.8742859352451,-12.2658211251852,3.11195213081256));
#10573=CARTESIAN_POINT('Ctrl Pts',(13.6136853347311,-11.9690250296368,3.00289613154459));
#10574=CARTESIAN_POINT('Ctrl Pts',(12.9449781782615,-10.6414226641662,2.93088718145296));
#10575=CARTESIAN_POINT('Ctrl Pts',(12.9421554343443,-9.9993047080392,2.89592528053768));
#10576=CARTESIAN_POINT('Ctrl Pts',(12.9427437076021,-10.0011914658147,3.65407471946232));
#10577=CARTESIAN_POINT('Ctrl Pts',(12.9469606388747,-9.39023291707249,3.62083451258795));
#10578=CARTESIAN_POINT('Ctrl Pts',(13.5593537346582,-8.09100528547459,3.55054725653724));
#10579=CARTESIAN_POINT('Ctrl Pts',(15.7683367683932,-7.69609503710994,3.44321295131019));
#10580=CARTESIAN_POINT('Ctrl Pts',(17.3523610419581,-9.39608196253575,3.33207180378117));
#10581=CARTESIAN_POINT('Ctrl Pts',(16.7831270202232,-11.6488715830789,3.22093065625215));
#10582=CARTESIAN_POINT('Ctrl Pts',(14.5816890215374,-12.3923493459239,3.10978950872313));
#10583=CARTESIAN_POINT('Ctrl Pts',(13.1262237587042,-11.234733613704,3.02083752979318));
#10584=CARTESIAN_POINT('Ctrl Pts',(12.9467998380999,-10.2759593928858,2.96893260003958));
#10585=CARTESIAN_POINT('Ctrl Pts',(12.9480746166703,-10.0010517736324,2.95407471946232));
#10586=CARTESIAN_POINT('Origin',(15.,-10.,9.54592528053767));
#10587=CARTESIAN_POINT('',(12.9444657818754,-9.9981973419728,4.35407471946232));
#10588=CARTESIAN_POINT('',(12.9473704108566,-10.0014953655277,4.29592528053768));
#10589=CARTESIAN_POINT('',(12.94525,-9.99999999999991,9.54592528053767));
#10590=CARTESIAN_POINT('Ctrl Pts',(12.9473704108566,-10.0014953655277,4.29592528053768));
#10591=CARTESIAN_POINT('Ctrl Pts',(12.9503841745306,-9.5543566229498,4.27173805572604));
#10592=CARTESIAN_POINT('Ctrl Pts',(13.3139392105709,-8.41788407722688,4.21050378173806));
#10593=CARTESIAN_POINT('Ctrl Pts',(15.1895240638759,-7.57876025621427,4.11222245857373));
#10594=CARTESIAN_POINT('Ctrl Pts',(17.1370408874533,-8.84614666745458,4.00108131104471));
#10595=CARTESIAN_POINT('Ctrl Pts',(17.1283949723014,-11.1697248007781,3.8899401635157));
#10596=CARTESIAN_POINT('Ctrl Pts',(15.1715004473266,-12.4225830974903,3.77879901598667));
#10597=CARTESIAN_POINT('Ctrl Pts',(13.3074684623944,-11.5719235526181,3.680794054994));
#10598=CARTESIAN_POINT('Ctrl Pts',(12.9503461916053,-10.4406482196211,3.61983614317767));
#10599=CARTESIAN_POINT('Ctrl Pts',(12.9474826545396,-9.9985576900864,3.59592528053768));
#10600=CARTESIAN_POINT('Ctrl Pts',(12.9444657818754,-9.9981973419728,4.35407471946232));
#10601=CARTESIAN_POINT('Ctrl Pts',(12.9432418473265,-9.86475792433196,4.346830523489));
#10602=CARTESIAN_POINT('Ctrl Pts',(13.0158869348842,-9.0502318191971,4.30253927833933));
#10603=CARTESIAN_POINT('Ctrl Pts',(14.1033972880174,-7.74291713830186,4.22120098401333));
#10604=CARTESIAN_POINT('Ctrl Pts',(16.4100928231865,-8.02263870329727,4.1100598364843));
#10605=CARTESIAN_POINT('Ctrl Pts',(17.4260451371735,-10.1123586227095,3.99891868895528));
#10606=CARTESIAN_POINT('Ctrl Pts',(16.2212916482552,-12.0992299010838,3.88777754142627));
#10607=CARTESIAN_POINT('Ctrl Pts',(13.8986160692799,-12.1645491227624,3.77663639389725));
#10608=CARTESIAN_POINT('Ctrl Pts',(12.9772494572038,-10.8215718924642,3.6987354532426));
#10609=CARTESIAN_POINT('Ctrl Pts',(12.9422607625827,-10.0711616334762,3.65788156176429));
#10610=CARTESIAN_POINT('Ctrl Pts',(12.9427437076021,-10.0011914658147,3.65407471946232));
#10611=CARTESIAN_POINT('Origin',(15.,-10.,9.54592528053767));
#10612=CARTESIAN_POINT('',(12.9486079625549,-9.99993062733875,5.05407471946232));
#10613=CARTESIAN_POINT('',(12.9420873854632,-10.0006073368552,4.99592528053768));
#10614=CARTESIAN_POINT('',(12.94525,-9.99999999999991,9.54592528053767));
#10615=CARTESIAN_POINT('Ctrl Pts',(12.9420873854632,-10.0006073368552,4.99592528053768));
#10616=CARTESIAN_POINT('Ctrl Pts',(12.9446118937168,-9.353470699709,4.96068701745075));
#10617=CARTESIAN_POINT('Ctrl Pts',(13.6226427058774,-8.02142229265111,4.88840170518746));
#10618=CARTESIAN_POINT('Ctrl Pts',(15.8911235009165,-7.74074787289641,4.77906934374785));
#10619=CARTESIAN_POINT('Ctrl Pts',(17.381434644454,-9.52346007316861,4.66792819621884));
#10620=CARTESIAN_POINT('Ctrl Pts',(16.6918746664094,-11.7423780820561,4.55678704868981));
#10621=CARTESIAN_POINT('Ctrl Pts',(14.453639508371,-12.3663920809676,4.4456459011608));
#10622=CARTESIAN_POINT('Ctrl Pts',(13.0937812261127,-11.1599030133838,4.35869197844341));
#10623=CARTESIAN_POINT('Ctrl Pts',(12.9457680578861,-10.2392293652314,4.30878510490238));
#10624=CARTESIAN_POINT('Ctrl Pts',(12.9473704108566,-10.0014953655277,4.29592528053768));
#10625=CARTESIAN_POINT('Ctrl Pts',(12.9486079625549,-9.99993062733875,5.05407471946232));
#10626=CARTESIAN_POINT('Ctrl Pts',(12.9485059618353,-9.66120350741247,5.03577948521371));
#10627=CARTESIAN_POINT('Ctrl Pts',(13.1882325310432,-8.63670467970468,4.98043720178874));
#10628=CARTESIAN_POINT('Ctrl Pts',(14.8046014971482,-7.57922762469993,4.88804786918745));
#10629=CARTESIAN_POINT('Ctrl Pts',(16.9278971004046,-8.52299890387884,4.77690672165843));
#10630=CARTESIAN_POINT('Ctrl Pts',(17.2864719188719,-10.8187585919275,4.6657655741294));
#10631=CARTESIAN_POINT('Ctrl Pts',(15.5521007403545,-12.3650590352537,4.55462442660039));
#10632=CARTESIAN_POINT('Ctrl Pts',(13.4583451014116,-11.7867971467844,4.45072747504469));
#10633=CARTESIAN_POINT('Ctrl Pts',(12.9495010876326,-10.547171360634,4.38387757266534));
#10634=CARTESIAN_POINT('Ctrl Pts',(12.9444657818754,-9.9981973419728,4.35407471946232));
#10635=CARTESIAN_POINT('Origin',(15.,-10.,9.54592528053767));
#10636=CARTESIAN_POINT('',(12.9447204535917,-10.0018385064059,5.75407471946232));
#10637=CARTESIAN_POINT('',(12.9455806254709,-9.99812308967269,5.69592528053768));
#10638=CARTESIAN_POINT('',(12.94525,-9.99999999999991,9.54592528053767));
#10639=CARTESIAN_POINT('Ctrl Pts',(12.9455806254709,-9.99812308967269,5.69592528053768));
#10640=CARTESIAN_POINT('Ctrl Pts',(12.9440384175881,-9.82764219444215,5.68668302835179));
#10641=CARTESIAN_POINT('Ctrl Pts',(13.0414312127959,-8.97553601260769,5.64039372698956));
#10642=CARTESIAN_POINT('Ctrl Pts',(14.2260750561177,-7.69796580272048,5.55705737645098));
#10643=CARTESIAN_POINT('Ctrl Pts',(16.5143902635653,-8.10133115083163,5.44591622892198));
#10644=CARTESIAN_POINT('Ctrl Pts',(17.4164924963646,-10.2426628994423,5.33477508139295));
#10645=CARTESIAN_POINT('Ctrl Pts',(16.1066330359978,-12.161870623064,5.22363393386394));
#10646=CARTESIAN_POINT('Ctrl Pts',(13.7838054461059,-12.1021874500104,5.1124927863349));
#10647=CARTESIAN_POINT('Ctrl Pts',(12.9577392822528,-10.7472711285552,5.03658990189283));
#10648=CARTESIAN_POINT('Ctrl Pts',(12.9419578020214,-10.0338249714567,4.99773406662709));
#10649=CARTESIAN_POINT('Ctrl Pts',(12.9420873854632,-10.0006073368552,4.99592528053768));
#10650=CARTESIAN_POINT('Ctrl Pts',(12.9447204535917,-10.0018385064059,5.75407471946232));
#10651=CARTESIAN_POINT('Ctrl Pts',(12.9497105203494,-9.46110245691194,5.72472844693841));
#10652=CARTESIAN_POINT('Ctrl Pts',(13.4456630876723,-8.22963759351343,5.65833512523816));
#10653=CARTESIAN_POINT('Ctrl Pts',(15.522981873134,-7.62833192925066,5.55489475436156));
#10654=CARTESIAN_POINT('Ctrl Pts',(17.2762329089047,-9.15319233958071,5.44375360683254));
#10655=CARTESIAN_POINT('Ctrl Pts',(16.9459103296842,-11.4531869986434,5.33261245930353));
#10656=CARTESIAN_POINT('Ctrl Pts',(14.8343783693084,-12.4229917343393,5.2214713117745));
#10657=CARTESIAN_POINT('Ctrl Pts',(13.1970788393113,-11.3803396321578,5.12862539849411));
#10658=CARTESIAN_POINT('Ctrl Pts',(12.9487125088312,-10.3471111103838,5.07282653439004));
#10659=CARTESIAN_POINT('Ctrl Pts',(12.9486079625549,-9.99993062733875,5.05407471946232));
#10660=CARTESIAN_POINT('Origin',(15.,-10.,9.54592528053767));
#10661=CARTESIAN_POINT('',(12.942563023563,-9.9989300295135,6.45407471946233));
#10662=CARTESIAN_POINT('',(12.9484828432129,-10.0005308591555,6.39592528053768));
#10663=CARTESIAN_POINT('',(12.94525,-9.99999999999991,9.54592528053767));
#10664=CARTESIAN_POINT('Ctrl Pts',(12.9484828432129,-10.0005308591555,6.39592528053768));
#10665=CARTESIAN_POINT('Ctrl Pts',(12.9493515264214,-9.62486768346204,6.3756319900765));
#10666=CARTESIAN_POINT('Ctrl Pts',(13.2280330621889,-8.56220125234328,6.31829165043898));
#10667=CARTESIAN_POINT('Ctrl Pts',(14.9350675128906,-7.57222224150645,6.2239042616251));
#10668=CARTESIAN_POINT('Ctrl Pts',(17.0045371624213,-8.62881361925355,6.1127631140961));
#10669=CARTESIAN_POINT('Ctrl Pts',(17.2391327429709,-10.94053487239,6.00162196656707));
#10670=CARTESIAN_POINT('Ctrl Pts',(15.4241147373104,-12.3913276502725,5.89048081903805));
#10671=CARTESIAN_POINT('Ctrl Pts',(13.4040950937302,-11.7145752509565,5.78858192369492));
#10672=CARTESIAN_POINT('Ctrl Pts',(12.950220271332,-10.5110052949291,5.72373007752813));
#10673=CARTESIAN_POINT('Ctrl Pts',(12.9455806254709,-9.99812308967269,5.69592528053768));
#10674=CARTESIAN_POINT('Ctrl Pts',(12.942563023563,-9.9989300295135,6.45407471946233));
#10675=CARTESIAN_POINT('Ctrl Pts',(12.9421731624654,-9.93736609179818,6.45072445783946));
#10676=CARTESIAN_POINT('Ctrl Pts',(12.9726043659186,-9.19542153869923,6.41032714704025));
#10677=CARTESIAN_POINT('Ctrl Pts',(13.8720874984692,-7.84915564699463,6.3328827870647));
#10678=CARTESIAN_POINT('Ctrl Pts',(16.1953903487128,-7.88591350252874,6.22174163953568));
#10679=CARTESIAN_POINT('Ctrl Pts',(17.4244804311674,-9.85782300540329,6.11060049200668));
#10680=CARTESIAN_POINT('Ctrl Pts',(16.4342968275999,-11.959875475957,5.99945934447763));
#10681=CARTESIAN_POINT('Ctrl Pts',(14.1312146931719,-12.2679355408755,5.88831819694863));
#10682=CARTESIAN_POINT('Ctrl Pts',(13.0215194433613,-10.9668271926417,5.80652332194351));
#10683=CARTESIAN_POINT('Ctrl Pts',(12.9434110065554,-10.1437334452495,5.76177549611475));
#10684=CARTESIAN_POINT('Ctrl Pts',(12.9447204535917,-10.0018385064059,5.75407471946232));
#10685=CARTESIAN_POINT('Origin',(15.,-10.,9.54592528053767));
#10686=CARTESIAN_POINT('',(12.9479406426496,-9.99884121834684,7.15407471946232));
#10687=CARTESIAN_POINT('',(12.9436342636416,-10.0016028715607,7.09592528053768));
#10688=CARTESIAN_POINT('',(12.94525,-9.99999999999991,9.54592528053767));
#10689=CARTESIAN_POINT('Ctrl Pts',(12.9436342636416,-10.0016028715607,7.09592528053768));
#10690=CARTESIAN_POINT('Ctrl Pts',(12.9485803298624,-9.42483824360876,7.06458095180121));
#10691=CARTESIAN_POINT('Ctrl Pts',(13.5024258720897,-8.15804701499923,6.99618957388838));
#10692=CARTESIAN_POINT('Ctrl Pts',(15.6497677058271,-7.65989035373928,6.89075114679923));
#10693=CARTESIAN_POINT('Ctrl Pts',(17.3184787010345,-9.27682680041793,6.77960999927021));
#10694=CARTESIAN_POINT('Ctrl Pts',(16.8649458764968,-11.5557312969865,6.66846885174119));
#10695=CARTESIAN_POINT('Ctrl Pts',(14.7043153699076,-12.4105788623587,6.55732770421217));
#10696=CARTESIAN_POINT('Ctrl Pts',(13.1594334243237,-11.3056861225605,6.46647984714433));
#10697=CARTESIAN_POINT('Ctrl Pts',(12.9477656747032,-10.3106713075848,6.41267903925284));
#10698=CARTESIAN_POINT('Ctrl Pts',(12.9484828432129,-10.0005308591555,6.39592528053768));
#10699=CARTESIAN_POINT('Ctrl Pts',(12.9479406426496,-9.99884121834684,7.15407471946232));
#10700=CARTESIAN_POINT('Ctrl Pts',(12.9465639668134,-9.73242150920767,7.13967341956416));
#10701=CARTESIAN_POINT('Ctrl Pts',(13.1185706050062,-8.78234603046162,7.08822507048967));
#10702=CARTESIAN_POINT('Ctrl Pts',(14.5523165742456,-7.61298740370139,6.99972967223882));
#10703=CARTESIAN_POINT('Ctrl Pts',(16.7627158202625,-8.32932372056038,6.88858852470981));
#10704=CARTESIAN_POINT('Ctrl Pts',(17.3596103902574,-10.5749548405481,6.77744737718078));
#10705=CARTESIAN_POINT('Ctrl Pts',(15.7966027972857,-12.2942827529436,6.66630622965177));
#10706=CARTESIAN_POINT('Ctrl Pts',(13.5735166885531,-11.9249990288555,6.55851534374561));
#10707=CARTESIAN_POINT('Ctrl Pts',(12.9464842297429,-10.6181374716992,6.4877715070158));
#10708=CARTESIAN_POINT('Ctrl Pts',(12.942563023563,-9.9989300295135,6.45407471946233));
#10709=CARTESIAN_POINT('Origin',(15.,-10.,9.54592528053767));
#10710=CARTESIAN_POINT('',(12.9473113312417,-10.0024712008536,7.85407471946232));
#10711=CARTESIAN_POINT('',(12.9434529369556,-9.99851181185547,7.79592528053768));
#10712=CARTESIAN_POINT('',(12.94525,-9.99999999999991,9.54592528053767));
#10713=CARTESIAN_POINT('',(14.4698297828114,-11.9851743256717,8.));
#10714=CARTESIAN_POINT('Ctrl Pts',(14.4698297828114,-11.9851743256717,8.));
#10715=CARTESIAN_POINT('Ctrl Pts',(13.8096927451188,-11.8088749487748,7.96295295082366));
#10716=CARTESIAN_POINT('Ctrl Pts',(13.0749951173004,-11.1129906421843,7.91431119064443));
#10717=CARTESIAN_POINT('Ctrl Pts',(12.9456876260347,-10.2167165909839,7.86566943046521));
#10718=CARTESIAN_POINT('Ctrl Pts',(12.9473113312417,-10.0024712008536,7.85407471946232));
#10719=CARTESIAN_POINT('',(15.5312697408697,-11.9887498021333,8.));
#10720=CARTESIAN_POINT('Origin',(15.,-10.,8.));
#10721=CARTESIAN_POINT('Ctrl Pts',(15.5312701240486,-11.9887510481705,8.));
#10722=CARTESIAN_POINT('Ctrl Pts',(14.8865854870743,-12.1601151282119,7.96367382485347));
#10723=CARTESIAN_POINT('Ctrl Pts',(13.5069338574846,-11.8405010530347,7.89564891836603));
#10724=CARTESIAN_POINT('Ctrl Pts',(12.948322230655,-10.581516770577,7.82762401187859));
#10725=CARTESIAN_POINT('Ctrl Pts',(12.9434529369556,-9.99851181185547,7.79592528053768));
#10726=CARTESIAN_POINT('Origin',(-15.,10.,9.54592528053767));
#10727=CARTESIAN_POINT('',(-17.051781505051,10.0008196635194,0.154074719462318));
#10728=CARTESIAN_POINT('',(-17.0565587168069,9.99843575839028,0.0959252805376745));
#10729=CARTESIAN_POINT('',(-17.05475,10.0000000000001,9.54592528053767));
#10730=CARTESIAN_POINT('',(-16.3390017195986,11.5585480285869,0.));
#10731=CARTESIAN_POINT('Ctrl Pts',(-17.0565587168069,9.99843575839027,0.0959252805376745));
#10732=CARTESIAN_POINT('Ctrl Pts',(-17.0518110208044,10.5850503744189,0.0639501870251164));
#10733=CARTESIAN_POINT('Ctrl Pts',(-16.7863171109466,11.1742441334025,0.0319750935125583));
#10734=CARTESIAN_POINT('Ctrl Pts',(-16.3390017195986,11.5585480285869,0.));
#10735=CARTESIAN_POINT('',(-15.3842290273038,12.0223109749866,-1.12886049415522E-15));
#10736=CARTESIAN_POINT('Origin',(-15.,10.,0.));
#10737=CARTESIAN_POINT('Ctrl Pts',(-17.051781505051,10.0008196635194,0.154074719462318));
#10738=CARTESIAN_POINT('Ctrl Pts',(-17.0529878932198,10.2789132148305,0.139042654788076));
#10739=CARTESIAN_POINT('Ctrl Pts',(-16.8731947834857,11.2276339555148,0.0876844149673036));
#10740=CARTESIAN_POINT('Ctrl Pts',(-16.0394222823928,11.8969878319988,0.0363261751465303));
#10741=CARTESIAN_POINT('Ctrl Pts',(-15.384229221931,12.022312258029,-5.35595873207839E-16));
#10742=CARTESIAN_POINT('Origin',(-15.,10.,9.54592528053767));
#10743=CARTESIAN_POINT('',(-17.0535052107051,9.99822649184017,0.854074719462319));
#10744=CARTESIAN_POINT('',(-17.0562188773561,10.0016641224949,0.795925280537675));
#10745=CARTESIAN_POINT('',(-17.05475,10.0000000000001,9.54592528053767));
#10746=CARTESIAN_POINT('Ctrl Pts',(-17.0562188773561,10.0016641224949,0.795925280537675));
#10747=CARTESIAN_POINT('Ctrl Pts',(-17.0571796395141,10.1117045841504,0.789946197926163));
#10748=CARTESIAN_POINT('Ctrl Pts',(-16.9990975224492,10.9025459743661,0.746920066138311));
#10749=CARTESIAN_POINT('Ctrl Pts',(-15.9729747466193,12.225122550715,0.66684688517412));
#10750=CARTESIAN_POINT('Ctrl Pts',(-13.6580451964401,12.0244599984212,0.555705737645099));
#10751=CARTESIAN_POINT('Ctrl Pts',(-12.5715926312396,9.9699163594395,0.444564590116078));
#10752=CARTESIAN_POINT('Ctrl Pts',(-13.7078058101514,7.94440559808363,0.333423442587059));
#10753=CARTESIAN_POINT('Ctrl Pts',(-16.0272308405357,7.79758227864481,0.222282295058039));
#10754=CARTESIAN_POINT('Ctrl Pts',(-17.0090843242089,9.13320995690963,0.143116241041577));
#10755=CARTESIAN_POINT('Ctrl Pts',(-17.0573118061957,9.90538573109153,0.100997236201456));
#10756=CARTESIAN_POINT('Ctrl Pts',(-17.0565587168069,9.99843575839027,0.0959252805376745));
#10757=CARTESIAN_POINT('Ctrl Pts',(-17.0535052107051,9.99822649184017,0.854074719462319));
#10758=CARTESIAN_POINT('Ctrl Pts',(-17.0495358029268,10.4798921752139,0.827991616512783));
#10759=CARTESIAN_POINT('Ctrl Pts',(-16.6400832266998,11.6517646154016,0.764861464386908));
#10760=CARTESIAN_POINT('Ctrl Pts',(-14.6871808849242,12.408440519574,0.664684263084692));
#10761=CARTESIAN_POINT('Ctrl Pts',(-12.8068360443054,11.0432447977232,0.553543115555672));
#10762=CARTESIAN_POINT('Ctrl Pts',(-12.9341204463425,8.72328850320409,0.442401968026654));
#10763=CARTESIAN_POINT('Ctrl Pts',(-14.9522477729176,7.57162591585277,0.331260820497632));
#10764=CARTESIAN_POINT('Ctrl Pts',(-16.7355222628146,8.49852169035672,0.235151737642854));
#10765=CARTESIAN_POINT('Ctrl Pts',(-17.0500147073812,9.59354193055857,0.176089703964416));
#10766=CARTESIAN_POINT('Ctrl Pts',(-17.051781505051,10.0008196635194,0.154074719462318));
#10767=CARTESIAN_POINT('Origin',(-15.,10.,9.54592528053767));
#10768=CARTESIAN_POINT('',(-17.0581308917344,10.0000299187367,1.55407471946232));
#10769=CARTESIAN_POINT('',(-17.0514805469147,10.0004498953059,1.49592528053768));
#10770=CARTESIAN_POINT('',(-17.05475,10.0000000000001,9.54592528053767));
#10771=CARTESIAN_POINT('Ctrl Pts',(-17.0514805469147,10.0004498953059,1.49592528053768));
#10772=CARTESIAN_POINT('Ctrl Pts',(-17.0520974357427,10.3157203081079,1.47889515965087));
#10773=CARTESIAN_POINT('Ctrl Pts',(-16.8355232105105,11.3160213722625,1.42481798958772));
#10774=CARTESIAN_POINT('Ctrl Pts',(-15.277737680073,12.4127105190431,1.33369377034824));
#10775=CARTESIAN_POINT('Ctrl Pts',(-13.1235279142844,11.5418130937198,1.22255262281922));
#10776=CARTESIAN_POINT('Ctrl Pts',(-12.6869684838201,9.25958637970326,1.1114114752902));
#10777=CARTESIAN_POINT('Ctrl Pts',(-14.3676628265377,7.65513319733112,1.00027032776118));
#10778=CARTESIAN_POINT('Ctrl Pts',(-16.5056252839035,8.16787157989892,0.895108262843672));
#10779=CARTESIAN_POINT('Ctrl Pts',(-17.0512266522036,9.42988185995992,0.826993247102503));
#10780=CARTESIAN_POINT('Ctrl Pts',(-17.0562188773561,10.0016641224949,0.795925280537675));
#10781=CARTESIAN_POINT('Ctrl Pts',(-17.0581308917344,10.0000299187367,1.55407471946232));
#10782=CARTESIAN_POINT('Ctrl Pts',(-17.0581312349042,10.0016288743118,1.55398762741383));
#10783=CARTESIAN_POINT('Ctrl Pts',(-17.0574054212678,10.6833881760579,1.516853486189));
#10784=CARTESIAN_POINT('Ctrl Pts',(-16.3123135322607,12.0435636244015,1.44267229578783));
#10785=CARTESIAN_POINT('Ctrl Pts',(-13.9947484023904,12.2108350155113,1.33153114825881));
#10786=CARTESIAN_POINT('Ctrl Pts',(-12.5973499293358,10.3543936440402,1.22039000072979));
#10787=CARTESIAN_POINT('Ctrl Pts',(-13.3992441080921,8.17355782375309,1.10924885320077));
#10788=CARTESIAN_POINT('Ctrl Pts',(-15.6664035170272,7.66456821418318,0.998107705671752));
#10789=CARTESIAN_POINT('Ctrl Pts',(-16.9346588395231,8.91110294463132,0.913049661092267));
#10790=CARTESIAN_POINT('Ctrl Pts',(-17.055173738162,9.79575991177017,0.865038665689123));
#10791=CARTESIAN_POINT('Ctrl Pts',(-17.0535052107051,9.99822649184017,0.854074719462319));
#10792=CARTESIAN_POINT('Origin',(-15.,10.,9.54592528053767));
#10793=CARTESIAN_POINT('',(-17.0534183096233,10.0017541282783,2.25407471946232));
#10794=CARTESIAN_POINT('',(-17.054572101898,9.99812063734445,2.19592528053768));
#10795=CARTESIAN_POINT('',(-17.05475,10.0000000000001,9.54592528053767));
#10796=CARTESIAN_POINT('Ctrl Pts',(-17.054572101898,9.99812063734445,2.19592528053768));
#10797=CARTESIAN_POINT('Ctrl Pts',(-17.0498495609752,10.5160021919663,2.16784412137558));
#10798=CARTESIAN_POINT('Ctrl Pts',(-16.5885931165834,11.7246094338528,2.10271591303714));
#10799=CARTESIAN_POINT('Ctrl Pts',(-14.5581012780927,12.3881050358458,2.00054065552236));
#10800=CARTESIAN_POINT('Ctrl Pts',(-12.7539301588106,10.9238456569314,1.88939950799334));
#10801=CARTESIAN_POINT('Ctrl Pts',(-13.0057226092633,8.61393421415536,1.77825836046432));
#10802=CARTESIAN_POINT('Ctrl Pts',(-15.0829976655305,7.57277312445451,1.6671172129353));
#10803=CARTESIAN_POINT('Ctrl Pts',(-16.7776411801768,8.57249168811958,1.57300618629308));
#10804=CARTESIAN_POINT('Ctrl Pts',(-17.0507554657768,9.6298861578658,1.51594220882721));
#10805=CARTESIAN_POINT('Ctrl Pts',(-17.0514805469147,10.0004498953059,1.49592528053768));
#10806=CARTESIAN_POINT('Ctrl Pts',(-17.0534183096233,10.0017541282783,2.25407471946232));
#10807=CARTESIAN_POINT('Ctrl Pts',(-17.0550897179391,10.2074604490073,2.24293658913854));
#10808=CARTESIAN_POINT('Ctrl Pts',(-16.9321369327745,11.0954235474083,2.19475140963841));
#10809=CARTESIAN_POINT('Ctrl Pts',(-15.655443965717,12.3385281044116,2.10951918096195));
#10810=CARTESIAN_POINT('Ctrl Pts',(-13.3906939975623,11.8189158098855,1.99837803343293));
#10811=CARTESIAN_POINT('Ctrl Pts',(-12.5990391016035,9.63433986139397,1.88723688590391));
#10812=CARTESIAN_POINT('Ctrl Pts',(-14.0051289214666,7.7844748128269,1.77609573837489));
#10813=CARTESIAN_POINT('Ctrl Pts',(-16.3200688809162,7.96247420798835,1.66504168289436));
#10814=CARTESIAN_POINT('Ctrl Pts',(-17.0579852579768,9.3214682069898,1.59103467659017));
#10815=CARTESIAN_POINT('Ctrl Pts',(-17.0581308917344,10.0000299187367,1.55407471946232));
#10816=CARTESIAN_POINT('Origin',(-15.,10.,9.54592528053767));
#10817=CARTESIAN_POINT('',(-17.0519255652782,9.99894822627429,2.95407471946232));
#10818=CARTESIAN_POINT('',(-17.0578444035932,10.0006952919057,2.89592528053767));
#10819=CARTESIAN_POINT('',(-17.05475,10.0000000000001,9.54592528053767));
#10820=CARTESIAN_POINT('Ctrl Pts',(-17.0578444035932,10.0006952919057,2.89592528053767));
#10821=CARTESIAN_POINT('Ctrl Pts',(-17.0580127536815,10.0389915801255,2.89384013227662));
#10822=CARTESIAN_POINT('Ctrl Pts',(-17.0396873009863,10.7575377341649,2.85470793483923));
#10823=CARTESIAN_POINT('Ctrl Pts',(-16.2005167352846,12.1111797432876,2.7785286882255));
#10824=CARTESIAN_POINT('Ctrl Pts',(-13.8773094989449,12.1535752538516,2.66738754069648));
#10825=CARTESIAN_POINT('Ctrl Pts',(-12.5817687604279,10.2246731230589,2.55624639316746));
#10826=CARTESIAN_POINT('Ctrl Pts',(-13.4997812925854,8.09011409287,2.44510524563844));
#10827=CARTESIAN_POINT('Ctrl Pts',(-15.7910347157817,7.70378912322181,2.33396409810942));
#10828=CARTESIAN_POINT('Ctrl Pts',(-16.9622413410058,8.98587389146773,2.2509041097425));
#10829=CARTESIAN_POINT('Ctrl Pts',(-17.0560799378907,9.83276887845376,2.20489117055192));
#10830=CARTESIAN_POINT('Ctrl Pts',(-17.054572101898,9.99812063734445,2.19592528053768));
#10831=CARTESIAN_POINT('Ctrl Pts',(-17.0519255652782,9.99894822627429,2.95407471946232));
#10832=CARTESIAN_POINT('Ctrl Pts',(-17.0500217756369,10.4095028825701,2.93188555086324));
#10833=CARTESIAN_POINT('Ctrl Pts',(-16.7315452143008,11.5082393895864,2.87264933308783));
#10834=CARTESIAN_POINT('Ctrl Pts',(-14.9409585995702,12.4279280521305,2.77636606613606));
#10835=CARTESIAN_POINT('Ctrl Pts',(-12.9281031098292,11.2671084366828,2.66522491860705));
#10836=CARTESIAN_POINT('Ctrl Pts',(-12.8117801189011,8.94642785381579,2.55408377107803));
#10837=CARTESIAN_POINT('Ctrl Pts',(-14.6984670947123,7.59014556097653,2.44294262354901));
#10838=CARTESIAN_POINT('Ctrl Pts',(-16.6444282224071,8.35460484167498,2.34293960634377));
#10839=CARTESIAN_POINT('Ctrl Pts',(-17.0495303696222,9.52325116446895,2.27998363831488));
#10840=CARTESIAN_POINT('Ctrl Pts',(-17.0534183096233,10.0017541282783,2.25407471946232));
#10841=CARTESIAN_POINT('Origin',(-15.,10.,9.54592528053767));
#10842=CARTESIAN_POINT('',(-17.0572564748192,9.99880853407964,3.65407471946232));
#10843=CARTESIAN_POINT('',(-17.0525171838174,10.0014423098,3.59592528053768));
#10844=CARTESIAN_POINT('',(-17.05475,10.0000000000001,9.54592528053767));
#10845=CARTESIAN_POINT('Ctrl Pts',(-17.0525171838174,10.0014423098,3.59592528053768));
#10846=CARTESIAN_POINT('Ctrl Pts',(-17.054090358096,10.2443186665424,3.58278909400133));
#10847=CARTESIAN_POINT('Ctrl Pts',(-16.9018844793529,11.1702542247926,3.53260585828864));
#10848=CARTESIAN_POINT('Ctrl Pts',(-15.5287351174808,12.3703922701155,3.44537557339962));
#10849=CARTESIAN_POINT('Ctrl Pts',(-13.2952058971985,11.7297391149084,3.33423442587059));
#10850=CARTESIAN_POINT('Ctrl Pts',(-12.6221777981957,9.50575116060393,3.22309327834158));
#10851=CARTESIAN_POINT('Ctrl Pts',(-14.125714133608,7.73417905325592,3.11195213081255));
#10852=CARTESIAN_POINT('Ctrl Pts',(-16.3863145560916,8.03097512543151,3.00289613154459));
#10853=CARTESIAN_POINT('Ctrl Pts',(-17.0550216598983,9.35857738634755,2.93088718145296));
#10854=CARTESIAN_POINT('Ctrl Pts',(-17.0578444035932,10.0006952919057,2.89592528053767));
#10855=CARTESIAN_POINT('Ctrl Pts',(-17.0572564748192,9.99880853407964,3.65407471946232));
#10856=CARTESIAN_POINT('Ctrl Pts',(-17.0530395431727,10.6097671369969,3.62083451258795));
#10857=CARTESIAN_POINT('Ctrl Pts',(-16.440646393087,11.9089948838,3.55054725653724));
#10858=CARTESIAN_POINT('Ctrl Pts',(-14.2316631634768,12.3039051671823,3.44321295131019));
#10859=CARTESIAN_POINT('Ctrl Pts',(-12.647638749453,10.6039180910149,3.33207180378117));
#10860=CARTESIAN_POINT('Ctrl Pts',(-13.2168728216632,8.35112827071217,3.22093065625215));
#10861=CARTESIAN_POINT('Ctrl Pts',(-15.4183110155551,7.60765044194128,3.10978950872313));
#10862=CARTESIAN_POINT('Ctrl Pts',(-16.8737764074476,8.76526627680962,3.02083752979319));
#10863=CARTESIAN_POINT('Ctrl Pts',(-17.0532003439618,9.72404058264425,2.96893260003958));
#10864=CARTESIAN_POINT('Ctrl Pts',(-17.0519255652782,9.99894822627429,2.95407471946232));
#10865=CARTESIAN_POINT('Origin',(-15.,10.,9.54592528053767));
#10866=CARTESIAN_POINT('',(-17.0555344003932,10.001802658187,4.35407471946232));
#10867=CARTESIAN_POINT('',(-17.0526294274916,9.99850463459006,4.29592528053768));
#10868=CARTESIAN_POINT('',(-17.05475,10.0000000000001,9.54592528053767));
#10869=CARTESIAN_POINT('Ctrl Pts',(-17.0526294274916,9.99850463459006,4.29592528053768));
#10870=CARTESIAN_POINT('Ctrl Pts',(-17.0496156640549,10.4456433419542,4.27173805572604));
#10871=CARTESIAN_POINT('Ctrl Pts',(-16.6860606566458,11.5821157981759,4.21050378173806));
#10872=CARTESIAN_POINT('Ctrl Pts',(-14.8104759510498,12.4212395531045,4.11222245857373));
#10873=CARTESIAN_POINT('Ctrl Pts',(-12.8629592808463,11.1538532416754,4.00108131104471));
#10874=CARTESIAN_POINT('Ctrl Pts',(-12.8716051953172,8.83027529134189,3.8899401635157));
#10875=CARTESIAN_POINT('Ctrl Pts',(-14.8284995661796,7.57741709329663,3.77879901598667));
#10876=CARTESIAN_POINT('Ctrl Pts',(-16.6925314043128,8.42807657117643,3.68079405499401));
#10877=CARTESIAN_POINT('Ctrl Pts',(-17.0496536469772,9.55935181508152,3.61983614317767));
#10878=CARTESIAN_POINT('Ctrl Pts',(-17.0525171838174,10.0014423098,3.59592528053768));
#10879=CARTESIAN_POINT('Ctrl Pts',(-17.0555344003932,10.001802658187,4.35407471946232));
#10880=CARTESIAN_POINT('Ctrl Pts',(-17.0567583350506,10.1352420876602,4.346830523489));
#10881=CARTESIAN_POINT('Ctrl Pts',(-16.9841132410514,10.9497682650209,4.30253927833933));
#10882=CARTESIAN_POINT('Ctrl Pts',(-15.8966027914863,12.2570830618385,4.22120098401332));
#10883=CARTESIAN_POINT('Ctrl Pts',(-13.5899070517775,11.9773614720396,4.11005983648431));
#10884=CARTESIAN_POINT('Ctrl Pts',(-12.5739546477039,9.8876413673274,3.99891868895528));
#10885=CARTESIAN_POINT('Ctrl Pts',(-13.7787082434502,7.90076991277298,3.88777754142627));
#10886=CARTESIAN_POINT('Ctrl Pts',(-16.1013840283822,7.83545068530234,3.77663639389724));
#10887=CARTESIAN_POINT('Ctrl Pts',(-17.0227507221578,9.1784280346853,3.6987354532426));
#10888=CARTESIAN_POINT('Ctrl Pts',(-17.0577394198814,9.92883836021378,3.65788156176429));
#10889=CARTESIAN_POINT('Ctrl Pts',(-17.0572564748192,9.99880853407964,3.65407471946232));
#10890=CARTESIAN_POINT('Origin',(-15.,10.,9.54592528053767));
#10891=CARTESIAN_POINT('',(-17.0513922193463,10.0000693726672,5.05407471946232));
#10892=CARTESIAN_POINT('',(-17.0579124524689,9.99939266319272,4.99592528053768));
#10893=CARTESIAN_POINT('',(-17.05475,10.0000000000001,9.54592528053767));
#10894=CARTESIAN_POINT('Ctrl Pts',(-17.0579124524689,9.99939266319272,4.99592528053768));
#10895=CARTESIAN_POINT('Ctrl Pts',(-17.0553879444141,10.6465292493746,4.96068701745074));
#10896=CARTESIAN_POINT('Ctrl Pts',(-16.3773571856509,11.9785775515288,4.88840170518747));
#10897=CARTESIAN_POINT('Ctrl Pts',(-14.1088765692626,12.2592519491796,4.77906934374786));
#10898=CARTESIAN_POINT('Ctrl Pts',(-12.6185655430924,10.4765398893022,4.66792819621883));
#10899=CARTESIAN_POINT('Ctrl Pts',(-13.3081254668317,8.25762205516231,4.55678704868981));
#10900=CARTESIAN_POINT('Ctrl Pts',(-15.5463604486011,7.63360810539413,4.44564590116079));
#10901=CARTESIAN_POINT('Ctrl Pts',(-16.9062186237658,8.84009707796262,4.35869197844341));
#10902=CARTESIAN_POINT('Ctrl Pts',(-17.0542317803359,9.76077065360876,4.30878510490238));
#10903=CARTESIAN_POINT('Ctrl Pts',(-17.0526294274916,9.99850463459006,4.29592528053768));
#10904=CARTESIAN_POINT('Ctrl Pts',(-17.0513922193463,10.0000693726672,5.05407471946232));
#10905=CARTESIAN_POINT('Ctrl Pts',(-17.051494220075,10.3387965226292,5.0357794852137));
#10906=CARTESIAN_POINT('Ctrl Pts',(-16.8117676296103,11.3632954411821,4.98043720178875));
#10907=CARTESIAN_POINT('Ctrl Pts',(-15.195398520178,12.4207725899548,4.88804786918745));
#10908=CARTESIAN_POINT('Ctrl Pts',(-13.0721027286448,11.4770012270902,4.77690672165843));
#10909=CARTESIAN_POINT('Ctrl Pts',(-12.7135278783817,9.18124133547139,4.66576557412941));
#10910=CARTESIAN_POINT('Ctrl Pts',(-14.4478992106895,7.63494075503149,4.55462442660039));
#10911=CARTESIAN_POINT('Ctrl Pts',(-16.5416550352902,8.21320269477644,4.45072747504469));
#10912=CARTESIAN_POINT('Ctrl Pts',(-17.0504990941895,9.45282859084715,4.38387757266534));
#10913=CARTESIAN_POINT('Ctrl Pts',(-17.0555344003932,10.001802658187,4.35407471946232));
#10914=CARTESIAN_POINT('Origin',(-15.,10.,9.54592528053767));
#10915=CARTESIAN_POINT('',(-17.0552797286464,9.99816149341417,5.75407471946232));
#10916=CARTESIAN_POINT('',(-17.0544192127363,10.0018769101795,5.69592528053768));
#10917=CARTESIAN_POINT('',(-17.05475,10.0000000000001,9.54592528053767));
#10918=CARTESIAN_POINT('Ctrl Pts',(-17.0544192127363,10.0018769101795,5.69592528053768));
#10919=CARTESIAN_POINT('Ctrl Pts',(-17.0559614204976,10.172357791985,5.68668302835179));
#10920=CARTESIAN_POINT('Ctrl Pts',(-16.9585686329592,11.0244639067171,5.64039372698956));
#10921=CARTESIAN_POINT('Ctrl Pts',(-15.7739248829336,12.3020340159819,5.557057376451));
#10922=CARTESIAN_POINT('Ctrl Pts',(-13.485609855698,11.8986686996438,5.44591622892196));
#10923=CARTESIAN_POINT('Ctrl Pts',(-12.5835076939429,9.75733711966703,5.33477508139296));
#10924=CARTESIAN_POINT('Ctrl Pts',(-13.8933670511534,7.83812954719161,5.22363393386392));
#10925=CARTESIAN_POINT('Ctrl Pts',(-16.2161944581144,7.89781271554394,5.11249278633492));
#10926=CARTESIAN_POINT('Ctrl Pts',(-17.0422605569119,9.25272893029508,5.03658990189283));
#10927=CARTESIAN_POINT('Ctrl Pts',(-17.0580420359005,9.96617503120721,4.99773406662709));
#10928=CARTESIAN_POINT('Ctrl Pts',(-17.0579124524689,9.99939266319272,4.99592528053768));
#10929=CARTESIAN_POINT('Ctrl Pts',(-17.0552797286464,9.99816149341417,5.75407471946232));
#10930=CARTESIAN_POINT('Ctrl Pts',(-17.050289661447,10.5388975908579,5.72472844693841));
#10931=CARTESIAN_POINT('Ctrl Pts',(-16.5543370501663,11.7703625634938,5.65833512523816));
#10932=CARTESIAN_POINT('Ctrl Pts',(-14.4770180804847,12.3716682810349,5.55489475436156));
#10933=CARTESIAN_POINT('Ctrl Pts',(-12.7237668892609,10.8468077355158,5.44375360683255));
#10934=CARTESIAN_POINT('Ctrl Pts',(-13.0540894977656,8.54681287249504,5.33261245930352));
#10935=CARTESIAN_POINT('Ctrl Pts',(-15.1656216453787,7.57700805081118,5.22147131177451));
#10936=CARTESIAN_POINT('Ctrl Pts',(-16.8029213205572,8.61966024544381,5.1286253984941));
#10937=CARTESIAN_POINT('Ctrl Pts',(-17.0512876730606,9.65288885883676,5.07282653439004));
#10938=CARTESIAN_POINT('Ctrl Pts',(-17.0513922193463,10.0000693726672,5.05407471946232));
#10939=CARTESIAN_POINT('Origin',(-15.,10.,9.54592528053767));
#10940=CARTESIAN_POINT('',(-17.0574371586977,10.0010699701727,6.45407471946232));
#10941=CARTESIAN_POINT('',(-17.0515169952491,9.99946914075972,6.39592528053768));
#10942=CARTESIAN_POINT('',(-17.05475,10.0000000000001,9.54592528053767));
#10943=CARTESIAN_POINT('Ctrl Pts',(-17.0515169952491,9.99946914075972,6.39592528053768));
#10944=CARTESIAN_POINT('Ctrl Pts',(-17.050648312096,10.3751322869369,6.3756319900765));
#10945=CARTESIAN_POINT('Ctrl Pts',(-16.7719667982161,11.4377986346686,6.31829165043897));
#10946=CARTESIAN_POINT('Ctrl Pts',(-15.0649324820269,12.4277775671245,6.22390426162511));
#10947=CARTESIAN_POINT('Ctrl Pts',(-12.9954629954269,11.3711862728547,6.11276311409609));
#10948=CARTESIAN_POINT('Ctrl Pts',(-12.7608674333771,9.05946520162959,6.00162196656707));
#10949=CARTESIAN_POINT('Ctrl Pts',(-14.5758852960858,7.60867253808055,5.89048081903805));
#10950=CARTESIAN_POINT('Ctrl Pts',(-16.5959047805884,8.285424884061,5.78858192369492));
#10951=CARTESIAN_POINT('Ctrl Pts',(-17.0497795672411,9.48899474531162,5.72373007752813));
#10952=CARTESIAN_POINT('Ctrl Pts',(-17.0544192127363,10.0018769101795,5.69592528053768));
#10953=CARTESIAN_POINT('Ctrl Pts',(-17.0574371586977,10.0010699701727,6.45407471946233));
#10954=CARTESIAN_POINT('Ctrl Pts',(-17.0578270198062,10.0626339132856,6.45072445783946));
#10955=CARTESIAN_POINT('Ctrl Pts',(-17.027395813414,10.8045785315454,6.41032714704025));
#10956=CARTESIAN_POINT('Ctrl Pts',(-16.1279126020198,12.1508445448559,6.33288278706471));
#10957=CARTESIAN_POINT('Ctrl Pts',(-13.8046095450231,12.114086684316,6.22174163953567));
#10958=CARTESIAN_POINT('Ctrl Pts',(-12.5755193539972,10.1421770075384,6.11060049200667));
#10959=CARTESIAN_POINT('Ctrl Pts',(-13.5657030451356,8.04012435007543,5.99945934447765));
#10960=CARTESIAN_POINT('Ctrl Pts',(-15.8687853839106,7.73206425811983,5.88831819694862));
#10961=CARTESIAN_POINT('Ctrl Pts',(-16.9784807320684,9.03317272161465,5.80652332194352));
#10962=CARTESIAN_POINT('Ctrl Pts',(-17.0565891757986,9.85626654198804,5.76177549611475));
#10963=CARTESIAN_POINT('Ctrl Pts',(-17.0552797286464,9.99816149341417,5.75407471946232));
#10964=CARTESIAN_POINT('Origin',(-15.,10.,9.54592528053767));
#10965=CARTESIAN_POINT('',(-17.0520595406494,10.0011587933795,7.15407471946233));
#10966=CARTESIAN_POINT('',(-17.0563655762952,9.99839712210779,7.09592528053768));
#10967=CARTESIAN_POINT('',(-17.05475,10.0000000000001,9.54592528053767));
#10968=CARTESIAN_POINT('Ctrl Pts',(-17.0563655762952,9.99839712210779,7.09592528053768));
#10969=CARTESIAN_POINT('Ctrl Pts',(-17.0514195106288,10.575161704561,7.0645809518012));
#10970=CARTESIAN_POINT('Ctrl Pts',(-16.4975740071439,11.8419528502525,6.99618957388838));
#10971=CARTESIAN_POINT('Ctrl Pts',(-14.3502323469365,12.3401094557021,6.89075114679924));
#10972=CARTESIAN_POINT('Ctrl Pts',(-12.6815214807272,10.7231731461125,6.77960999927021));
#10973=CARTESIAN_POINT('Ctrl Pts',(-13.1350542708035,8.44426882360712,6.66846885174119));
#10974=CARTESIAN_POINT('Ctrl Pts',(-15.2956846065833,7.58942132854296,6.55732770421217));
#10975=CARTESIAN_POINT('Ctrl Pts',(-16.8405664307791,8.69431397998541,6.46647984714433));
#10976=CARTESIAN_POINT('Ctrl Pts',(-17.0522341637131,9.68932871669844,6.41267903925284));
#10977=CARTESIAN_POINT('Ctrl Pts',(-17.0515169952491,9.99946914075972,6.39592528053768));
#10978=CARTESIAN_POINT('Ctrl Pts',(-17.0520595406494,10.0011587933795,7.15407471946232));
#10979=CARTESIAN_POINT('Ctrl Pts',(-17.0534362134906,10.2675785134614,7.13967341956416));
#10980=CARTESIAN_POINT('Ctrl Pts',(-16.8814295491932,11.2176540291726,7.08822507048967));
#10981=CARTESIAN_POINT('Ctrl Pts',(-15.447683477411,12.3870128478829,6.99972967223881));
#10982=CARTESIAN_POINT('Ctrl Pts',(-13.2372840161297,11.670676405265,6.88858852470981));
#10983=CARTESIAN_POINT('Ctrl Pts',(-12.6403894048645,9.42504512087116,6.77744737718078));
#10984=CARTESIAN_POINT('Ctrl Pts',(-14.2033971295295,7.70571703676082,6.66630622965177));
#10985=CARTESIAN_POINT('Ctrl Pts',(-16.4264834392857,8.07500080390432,6.55851534374561));
#10986=CARTESIAN_POINT('Ctrl Pts',(-17.0535159524081,9.38186247369755,6.4877715070158));
#10987=CARTESIAN_POINT('Ctrl Pts',(-17.0574371586977,10.0010699701727,6.45407471946233));
#10988=CARTESIAN_POINT('Origin',(-15.,10.,9.54592528053767));
#10989=CARTESIAN_POINT('',(-17.052688542414,9.99752997529134,7.85407471946233));
#10990=CARTESIAN_POINT('',(-17.056546936061,10.0014880949897,7.79592528053768));
#10991=CARTESIAN_POINT('',(-17.05475,10.0000000000001,9.54592528053767));
#10992=CARTESIAN_POINT('',(-15.5301702171886,8.01482567432828,8.));
#10993=CARTESIAN_POINT('Ctrl Pts',(-15.5301702171886,8.01482567432828,8.));
#10994=CARTESIAN_POINT('Ctrl Pts',(-16.1903072548812,8.1911250512252,7.96295295082366));
#10995=CARTESIAN_POINT('Ctrl Pts',(-16.9250045409916,8.88701144695482,7.91431119064444));
#10996=CARTESIAN_POINT('Ctrl Pts',(-17.0543121964904,9.78328481586603,7.86566943046521));
#10997=CARTESIAN_POINT('Ctrl Pts',(-17.052688542414,9.99752997529134,7.85407471946233));
#10998=CARTESIAN_POINT('',(-14.4687306105943,8.01125000725434,8.));
#10999=CARTESIAN_POINT('Origin',(-15.,10.,8.));
#11000=CARTESIAN_POINT('Ctrl Pts',(-14.4687302296836,8.0112487681312,8.));
#11001=CARTESIAN_POINT('Ctrl Pts',(-15.1134150435372,7.83988452957895,7.96367382485347));
#11002=CARTESIAN_POINT('Ctrl Pts',(-16.4930655292016,8.15949974734112,7.89564891836604));
#11003=CARTESIAN_POINT('Ctrl Pts',(-17.0516775383829,9.41848331501726,7.82762401187859));
#11004=CARTESIAN_POINT('Ctrl Pts',(-17.056546936061,10.0014880949897,7.79592528053768));
#11005=CARTESIAN_POINT('Origin',(15.,10.,9.54592528053767));
#11006=CARTESIAN_POINT('',(12.9482186935975,10.0008196174515,0.15407471946232));
#11007=CARTESIAN_POINT('',(12.943442368457,9.99843416552646,0.0959252805376746));
#11008=CARTESIAN_POINT('',(12.94525,10.0000000000001,9.54592528053767));
#11009=CARTESIAN_POINT('',(13.6609982804014,11.5585480285869,0.));
#11010=CARTESIAN_POINT('Ctrl Pts',(12.943442368457,9.99843416552646,0.0959252805376745));
#11011=CARTESIAN_POINT('Ctrl Pts',(12.9481898548418,10.5850491239192,0.0639501870251164));
#11012=CARTESIAN_POINT('Ctrl Pts',(13.2136828890534,11.1742441334025,0.0319750935125583));
#11013=CARTESIAN_POINT('Ctrl Pts',(13.6609982804014,11.5585480285869,0.));
#11014=CARTESIAN_POINT('',(14.6157707560785,12.0223109855879,-5.36454528360574E-16));
#11015=CARTESIAN_POINT('Origin',(15.,10.,0.));
#11016=CARTESIAN_POINT('Ctrl Pts',(12.9482186935975,10.0008196174515,0.15407471946232));
#11017=CARTESIAN_POINT('Ctrl Pts',(12.9470123424645,10.2789131332973,0.139042654788077));
#11018=CARTESIAN_POINT('Ctrl Pts',(13.1268055014811,11.2276337797824,0.0876844149673041));
#11019=CARTESIAN_POINT('Ctrl Pts',(13.9605773780345,11.8969878744382,0.0363261751465303));
#11020=CARTESIAN_POINT('Ctrl Pts',(14.6157705619694,12.0223122647246,-5.44540541130845E-16));
#11021=CARTESIAN_POINT('Origin',(15.,10.,9.54592528053767));
#11022=CARTESIAN_POINT('',(12.9464948772178,9.99822649168832,0.85407471946232));
#11023=CARTESIAN_POINT('',(12.9437809019177,10.0016640710788,0.795925280537675));
#11024=CARTESIAN_POINT('',(12.94525,10.0000000000001,9.54592528053767));
#11025=CARTESIAN_POINT('Ctrl Pts',(12.9437809019177,10.0016640710788,0.795925280537675));
#11026=CARTESIAN_POINT('Ctrl Pts',(12.9428201393579,10.1117045448354,0.789946197926163));
#11027=CARTESIAN_POINT('Ctrl Pts',(13.0009022569502,10.90254603781,0.746920066138311));
#11028=CARTESIAN_POINT('Ctrl Pts',(14.0270250684493,12.2251230724266,0.66684688517412));
#11029=CARTESIAN_POINT('Ctrl Pts',(16.3419551102441,12.024459772841,0.555705737645098));
#11030=CARTESIAN_POINT('Ctrl Pts',(17.4284073232916,9.96991710195404,0.444564590116078));
#11031=CARTESIAN_POINT('Ctrl Pts',(16.2921949921082,7.9444041673974,0.333423442587059));
#11032=CARTESIAN_POINT('Ctrl Pts',(13.9727677026847,7.79758395766853,0.222282295058038));
#11033=CARTESIAN_POINT('Ctrl Pts',(12.9909169312602,9.13320804851158,0.143116241041577));
#11034=CARTESIAN_POINT('Ctrl Pts',(12.9426893123183,9.90538408392121,0.100997236201456));
#11035=CARTESIAN_POINT('Ctrl Pts',(12.943442368457,9.99843416552646,0.0959252805376745));
#11036=CARTESIAN_POINT('Ctrl Pts',(12.9464948772178,9.99822649168832,0.85407471946232));
#11037=CARTESIAN_POINT('Ctrl Pts',(12.9504642873018,10.4798921519117,0.827991616512784));
#11038=CARTESIAN_POINT('Ctrl Pts',(13.3599168531639,11.6517645344229,0.764861464386909));
#11039=CARTESIAN_POINT('Ctrl Pts',(15.3128190766481,12.4084404416678,0.664684263084692));
#11040=CARTESIAN_POINT('Ctrl Pts',(17.1931639076296,11.0432447117585,0.553543115555672));
#11041=CARTESIAN_POINT('Ctrl Pts',(17.0658793839574,8.72328862566383,0.442401968026654));
#11042=CARTESIAN_POINT('Ctrl Pts',(15.0477523711852,7.57162591137588,0.331260820497632));
#11043=CARTESIAN_POINT('Ctrl Pts',(13.2644776059679,8.49852188099848,0.235151737642855));
#11044=CARTESIAN_POINT('Ctrl Pts',(12.9499854370273,9.59354193643066,0.176089703964417));
#11045=CARTESIAN_POINT('Ctrl Pts',(12.9482186935975,10.0008196174515,0.15407471946232));
#11046=CARTESIAN_POINT('Origin',(15.,10.,9.54592528053767));
#11047=CARTESIAN_POINT('',(12.9418691959132,10.000029918806,1.55407471946232));
#11048=CARTESIAN_POINT('',(12.9485192215913,10.0004498942776,1.49592528053768));
#11049=CARTESIAN_POINT('',(12.94525,10.0000000000001,9.54592528053767));
#11050=CARTESIAN_POINT('Ctrl Pts',(12.9485192215913,10.0004498942776,1.49592528053768));
#11051=CARTESIAN_POINT('Ctrl Pts',(12.947902332727,10.3157203421523,1.47889515965087));
#11052=CARTESIAN_POINT('Ctrl Pts',(13.1644765824467,11.3160215182978,1.42481798958772));
#11053=CARTESIAN_POINT('Ctrl Pts',(14.7222622877187,12.4127108006303,1.33369377034824));
#11054=CARTESIAN_POINT('Ctrl Pts',(16.8764722993871,11.541813251237,1.22255262281922));
#11055=CARTESIAN_POINT('Ctrl Pts',(17.3130317733822,9.25958632559344,1.1114114752902));
#11056=CARTESIAN_POINT('Ctrl Pts',(15.6323372531142,7.65513288048749,1.00027032776118));
#11057=CARTESIAN_POINT('Ctrl Pts',(13.4943745301596,8.16787145671535,0.895108262843671));
#11058=CARTESIAN_POINT('Ctrl Pts',(12.9487731291581,9.42988174566537,0.826993247102503));
#11059=CARTESIAN_POINT('Ctrl Pts',(12.9437809019177,10.0016640710788,0.795925280537675));
#11060=CARTESIAN_POINT('Ctrl Pts',(12.9418691959133,10.000029918806,1.55407471946232));
#11061=CARTESIAN_POINT('Ctrl Pts',(12.9418688527435,10.0016288743128,1.55398762741383));
#11062=CARTESIAN_POINT('Ctrl Pts',(12.9425946663912,10.6833881469544,1.516853486189));
#11063=CARTESIAN_POINT('Ctrl Pts',(13.6876865240177,12.0435635368564,1.44267229578783));
#11064=CARTESIAN_POINT('Ctrl Pts',(16.0052515541106,12.2108349221453,1.33153114825881));
#11065=CARTESIAN_POINT('Ctrl Pts',(17.402649969509,10.3543936274306,1.22039000072979));
#11066=CARTESIAN_POINT('Ctrl Pts',(16.6007558214423,8.1735579042694,1.10924885320077));
#11067=CARTESIAN_POINT('Ctrl Pts',(14.333596515509,7.6645683089416,0.998107705671753));
#11068=CARTESIAN_POINT('Ctrl Pts',(13.0653412380888,8.91110299629741,0.913049661092268));
#11069=CARTESIAN_POINT('Ctrl Pts',(12.9448263487916,9.79575992134947,0.865038665689124));
#11070=CARTESIAN_POINT('Ctrl Pts',(12.9464948772178,9.99822649168832,0.85407471946232));
#11071=CARTESIAN_POINT('Origin',(15.,10.,9.54592528053767));
#11072=CARTESIAN_POINT('',(12.9465817778743,10.0017541282055,2.25407471946232));
#11073=CARTESIAN_POINT('',(12.9454276661632,9.99812063713314,2.19592528053768));
#11074=CARTESIAN_POINT('',(12.94525,10.0000000000001,9.54592528053767));
#11075=CARTESIAN_POINT('Ctrl Pts',(12.9454276661632,9.99812063713314,2.19592528053768));
#11076=CARTESIAN_POINT('Ctrl Pts',(12.9501502076194,10.516002250193,2.16784412137558));
#11077=CARTESIAN_POINT('Ctrl Pts',(13.4114067040829,11.7246096284375,2.10271591303714));
#11078=CARTESIAN_POINT('Ctrl Pts',(15.4418987717874,12.3881053056886,2.00054065552236));
#11079=CARTESIAN_POINT('Ctrl Pts',(17.2460700947607,10.9238457607613,1.88939950799334));
#11080=CARTESIAN_POINT('Ctrl Pts',(16.9942776158352,8.61393405853105,1.77825836046432));
#11081=CARTESIAN_POINT('Ctrl Pts',(14.9170023251788,7.57277284889803,1.6671172129353));
#11082=CARTESIAN_POINT('Ctrl Pts',(13.2223586190082,8.57249152911901,1.57300618629308));
#11083=CARTESIAN_POINT('Ctrl Pts',(12.9492443027719,9.62988611561382,1.51594220882721));
#11084=CARTESIAN_POINT('Ctrl Pts',(12.9485192215913,10.0004498942776,1.49592528053768));
#11085=CARTESIAN_POINT('Ctrl Pts',(12.9465817778743,10.0017541282055,2.25407471946232));
#11086=CARTESIAN_POINT('Ctrl Pts',(12.9449103696296,10.2074604401693,2.24293658913854));
#11087=CARTESIAN_POINT('Ctrl Pts',(13.067863149555,11.095423500733,2.19475140963841));
#11088=CARTESIAN_POINT('Ctrl Pts',(14.3445560622211,12.3385280047513,2.10951918096195));
#11089=CARTESIAN_POINT('Ctrl Pts',(16.6093059338468,11.8189157324019,1.99837803343293));
#11090=CARTESIAN_POINT('Ctrl Pts',(17.4009607961183,9.63433987693309,1.88723688590391));
#11091=CARTESIAN_POINT('Ctrl Pts',(15.9948710360845,7.78447490731078,1.77609573837489));
#11092=CARTESIAN_POINT('Ctrl Pts',(13.6799311754379,7.96247429466911,1.66504168289436));
#11093=CARTESIAN_POINT('Ctrl Pts',(12.9420148296229,9.32146823602665,1.59103467659017));
#11094=CARTESIAN_POINT('Ctrl Pts',(12.9418691959133,10.000029918806,1.55407471946232));
#11095=CARTESIAN_POINT('Origin',(15.,10.,9.54592528053767));
#11096=CARTESIAN_POINT('',(12.9480745221571,9.99894822631912,2.95407471946232));
#11097=CARTESIAN_POINT('',(12.9421553640983,10.0006952919847,2.89592528053768));
#11098=CARTESIAN_POINT('',(12.94525,10.0000000000001,9.54592528053767));
#11099=CARTESIAN_POINT('Ctrl Pts',(12.9421553640983,10.0006952919847,2.89592528053768));
#11100=CARTESIAN_POINT('Ctrl Pts',(12.941987013991,10.0389915845278,2.89384013227662));
#11101=CARTESIAN_POINT('Ctrl Pts',(12.9603124687549,10.7575378196829,2.85470793483923));
#11102=CARTESIAN_POINT('Ctrl Pts',(13.79948312919,12.1111799816138,2.77852868822549));
#11103=CARTESIAN_POINT('Ctrl Pts',(16.1226906277949,12.1535754969733,2.66738754069648));
#11104=CARTESIAN_POINT('Ctrl Pts',(17.4182315125643,10.2246731484105,2.55624639316745));
#11105=CARTESIAN_POINT('Ctrl Pts',(16.5002188767733,8.09011387728591,2.44510524563844));
#11106=CARTESIAN_POINT('Ctrl Pts',(14.208965194919,7.70378886396441,2.33396409810942));
#11107=CARTESIAN_POINT('Ctrl Pts',(13.0377584374779,8.9858737770289,2.2509041097425));
#11108=CARTESIAN_POINT('Ctrl Pts',(12.9439198300002,9.83276885958405,2.20489117055192));
#11109=CARTESIAN_POINT('Ctrl Pts',(12.9454276661632,9.99812063713314,2.19592528053768));
#11110=CARTESIAN_POINT('Ctrl Pts',(12.9480745221571,9.99894822631912,2.95407471946232));
#11111=CARTESIAN_POINT('Ctrl Pts',(12.9499783117173,10.4095028651207,2.93188555086324));
#11112=CARTESIAN_POINT('Ctrl Pts',(13.2684548594827,11.5082393253183,2.87264933308783));
#11113=CARTESIAN_POINT('Ctrl Pts',(15.0590413979142,12.4279279486728,2.77636606613607));
#11114=CARTESIAN_POINT('Ctrl Pts',(17.071896801884,11.2671083826901,2.66522491860705));
#11115=CARTESIAN_POINT('Ctrl Pts',(17.1882197878565,8.94642789870889,2.55408377107803));
#11116=CARTESIAN_POINT('Ctrl Pts',(15.3015328924376,7.59014566366572,2.44294262354901));
#11117=CARTESIAN_POINT('Ctrl Pts',(13.3555718476664,8.35460491178446,2.34293960634377));
#11118=CARTESIAN_POINT('Ctrl Pts',(12.9504697177102,9.52325118478529,2.27998363831488));
#11119=CARTESIAN_POINT('Ctrl Pts',(12.9465817778743,10.0017541282055,2.25407471946232));
#11120=CARTESIAN_POINT('Origin',(15.,10.,9.54592528053767));
#11121=CARTESIAN_POINT('',(12.9427436128433,9.99880853413039,3.65407471946232));
#11122=CARTESIAN_POINT('',(12.9474825844755,10.0014423099628,3.59592528053768));
#11123=CARTESIAN_POINT('',(12.94525,10.0000000000001,9.54592528053767));
#11124=CARTESIAN_POINT('Ctrl Pts',(12.9474825844755,10.0014423099628,3.59592528053768));
#11125=CARTESIAN_POINT('Ctrl Pts',(12.9459094100193,10.2443186941233,3.58278909400133));
#11126=CARTESIAN_POINT('Ctrl Pts',(13.0981153059447,11.1702543569017,3.53260585828864));
#11127=CARTESIAN_POINT('Ctrl Pts',(14.4712648228307,12.3703925377072,3.44537557339962));
#11128=CARTESIAN_POINT('Ctrl Pts',(16.7047942952545,11.7297393101775,3.33423442587059));
#11129=CARTESIAN_POINT('Ctrl Pts',(17.3778224702348,9.50575110480829,3.22309327834158));
#11130=CARTESIAN_POINT('Ctrl Pts',(15.8742859650895,7.73417879746959,3.11195213081255));
#11131=CARTESIAN_POINT('Ctrl Pts',(13.6136852874083,8.03097490314885,3.00289613154459));
#11132=CARTESIAN_POINT('Ctrl Pts',(12.9449781081118,9.35857731393861,2.93088718145296));
#11133=CARTESIAN_POINT('Ctrl Pts',(12.9421553640983,10.0006952919847,2.89592528053768));
#11134=CARTESIAN_POINT('Ctrl Pts',(12.9427436128433,9.99880853413039,3.65407471946232));
#11135=CARTESIAN_POINT('Ctrl Pts',(12.9469605443102,10.6097671110138,3.62083451258795));
#11136=CARTESIAN_POINT('Ctrl Pts',(13.5593536683009,11.9089948024551,3.55054725653724));
#11137=CARTESIAN_POINT('Ctrl Pts',(15.7683368037833,12.3039050690097,3.44321295131019));
#11138=CARTESIAN_POINT('Ctrl Pts',(17.3523611503097,10.6039180652812,3.33207180378117));
#11139=CARTESIAN_POINT('Ctrl Pts',(16.7831271023553,8.35112834097283,3.22093065625215));
#11140=CARTESIAN_POINT('Ctrl Pts',(14.5816890022697,7.60765054388266,3.10978950872313));
#11141=CARTESIAN_POINT('Ctrl Pts',(13.1262236723966,8.76526632942327,3.02083752979318));
#11142=CARTESIAN_POINT('Ctrl Pts',(12.9467997435279,9.72404059440326,2.96893260003958));
#11143=CARTESIAN_POINT('Ctrl Pts',(12.9480745221571,9.99894822631912,2.95407471946232));
#11144=CARTESIAN_POINT('Origin',(15.,10.,9.54592528053767));
#11145=CARTESIAN_POINT('',(12.944465687196,10.0018026581102,4.35407471946232));
#11146=CARTESIAN_POINT('',(12.9473703407886,9.99850463442125,4.29592528053768));
#11147=CARTESIAN_POINT('',(12.94525,10.0000000000001,9.54592528053767));
#11148=CARTESIAN_POINT('Ctrl Pts',(12.9473703407886,9.99850463442125,4.29592528053768));
#11149=CARTESIAN_POINT('Ctrl Pts',(12.9503841045655,10.4456433922625,4.27173805572604));
#11150=CARTESIAN_POINT('Ctrl Pts',(13.3139391530161,11.5821159767798,4.21050378173806));
#11151=CARTESIAN_POINT('Ctrl Pts',(15.1895240703454,12.4212398264365,4.11222245857373));
#11152=CARTESIAN_POINT('Ctrl Pts',(17.1370409604027,11.1538533719331,4.00108131104472));
#11153=CARTESIAN_POINT('Ctrl Pts',(17.1283950449557,8.83027515929254,3.88994016351569));
#11154=CARTESIAN_POINT('Ctrl Pts',(15.1715004531809,7.57741681981306,3.77879901598667));
#11155=CARTESIAN_POINT('Ctrl Pts',(13.3074684046186,8.42807639372317,3.680794054994));
#11156=CARTESIAN_POINT('Ctrl Pts',(12.9503461216389,9.55935176533709,3.61983614317767));
#11157=CARTESIAN_POINT('Ctrl Pts',(12.9474825844755,10.0014423099628,3.59592528053768));
#11158=CARTESIAN_POINT('Ctrl Pts',(12.944465687196,10.0018026581102,4.35407471946232));
#11159=CARTESIAN_POINT('Ctrl Pts',(12.9432417525907,10.1352420818974,4.346830523489));
#11160=CARTESIAN_POINT('Ctrl Pts',(13.0158868434944,10.9497682245499,4.30253927833933));
#11161=CARTESIAN_POINT('Ctrl Pts',(14.1033972467191,12.2570829656611,4.22120098401333));
#11162=CARTESIAN_POINT('Ctrl Pts',(16.4100928881365,11.9773613877815,4.11005983648431));
#11163=CARTESIAN_POINT('Ctrl Pts',(17.4260452489189,9.88764137211515,3.99891868895528));
#11164=CARTESIAN_POINT('Ctrl Pts',(16.2212917045089,7.90077000222407,3.88777754142627));
#11165=CARTESIAN_POINT('Ctrl Pts',(13.8986160185493,7.83545077753679,3.77663639389725));
#11166=CARTESIAN_POINT('Ctrl Pts',(12.9772493640344,9.17842806969361,3.6987354532426));
#11167=CARTESIAN_POINT('Ctrl Pts',(12.9422606678017,9.92883836324606,3.65788156176429));
#11168=CARTESIAN_POINT('Ctrl Pts',(12.9427436128433,9.99880853413039,3.65407471946232));
#11169=CARTESIAN_POINT('Origin',(15.,10.,9.54592528053767));
#11170=CARTESIAN_POINT('',(12.9486078680663,10.0000693726643,5.05407471946232));
#11171=CARTESIAN_POINT('',(12.9420873152149,9.99939266312408,4.99592528053768));
#11172=CARTESIAN_POINT('',(12.94525,10.0000000000001,9.54592528053767));
#11173=CARTESIAN_POINT('Ctrl Pts',(12.9420873152149,9.99939266312408,4.99592528053768));
#11174=CARTESIAN_POINT('Ctrl Pts',(12.9446118235547,10.6465293223607,4.96068701745075));
#11175=CARTESIAN_POINT('Ctrl Pts',(13.6226426588603,11.9785777748891,4.88840170518747));
#11176=CARTESIAN_POINT('Ctrl Pts',(15.8911235313356,12.2592522042247,4.77906934374785));
#11177=CARTESIAN_POINT('Ctrl Pts',(17.381434725746,10.4765399430985,4.66792819621883));
#11178=CARTESIAN_POINT('Ctrl Pts',(16.6918747241627,8.25762185846654,4.55678704868982));
#11179=CARTESIAN_POINT('Ctrl Pts',(14.4536394897207,7.63360783825394,4.44564590116079));
#11180=CARTESIAN_POINT('Ctrl Pts',(13.0937811610426,8.84009694702206,4.35869197844341));
#11181=CARTESIAN_POINT('Ctrl Pts',(12.9457679877634,9.76077062660234,4.30878510490238));
#11182=CARTESIAN_POINT('Ctrl Pts',(12.9473703407886,9.99850463442125,4.29592528053768));
#11183=CARTESIAN_POINT('Ctrl Pts',(12.9486078680663,10.0000693726643,5.05407471946232));
#11184=CARTESIAN_POINT('Ctrl Pts',(12.9485058673419,10.3387965081927,5.0357794852137));
#11185=CARTESIAN_POINT('Ctrl Pts',(13.1882324475917,11.36329538309,4.98043720178874));
#11186=CARTESIAN_POINT('Ctrl Pts',(14.8046014881481,12.4207724868025,4.88804786918745));
#11187=CARTESIAN_POINT('Ctrl Pts',(16.9278971892049,11.4770011641531,4.77690672165842));
#11188=CARTESIAN_POINT('Ctrl Pts',(17.2864720241886,9.18124137035986,4.66576557412941));
#11189=CARTESIAN_POINT('Ctrl Pts',(15.5521007657847,7.63494085580992,4.55462442660038));
#11190=CARTESIAN_POINT('Ctrl Pts',(13.4583450304019,8.21320277091433,4.45072747504469));
#11191=CARTESIAN_POINT('Ctrl Pts',(12.9495009931851,9.45282861416286,4.38387757266534));
#11192=CARTESIAN_POINT('Ctrl Pts',(12.944465687196,10.0018026581102,4.35407471946232));
#11193=CARTESIAN_POINT('Origin',(15.,10.,9.54592528053767));
#11194=CARTESIAN_POINT('',(12.9447203589281,9.99816149350058,5.75407471946233));
#11195=CARTESIAN_POINT('',(12.9455805553419,10.0018769103914,5.69592528053768));
#11196=CARTESIAN_POINT('',(12.94525,10.0000000000001,9.54592528053767));
#11197=CARTESIAN_POINT('Ctrl Pts',(12.9455805553419,10.0018769103914,5.69592528053768));
#11198=CARTESIAN_POINT('Ctrl Pts',(12.9440383474063,10.172357811441,5.68668302835179));
#11199=CARTESIAN_POINT('Ctrl Pts',(13.0414311459384,11.024464022361,5.64039372698956));
#11200=CARTESIAN_POINT('Ctrl Pts',(14.2260750296995,12.3020342758629,5.55705737645099));
#11201=CARTESIAN_POINT('Ctrl Pts',(16.51439031526,11.8986689139798,5.44591622892198));
#11202=CARTESIAN_POINT('Ctrl Pts',(17.4164925788533,9.75733709227475,5.33477508139295));
#11203=CARTESIAN_POINT('Ctrl Pts',(16.1066330737735,7.83812930313874,5.22363393386394));
#11204=CARTESIAN_POINT('Ctrl Pts',(13.7838054045903,7.89781247823008,5.11249278633491));
#11205=CARTESIAN_POINT('Ctrl Pts',(12.9577392125388,9.25272884593619,5.03658990189283));
#11206=CARTESIAN_POINT('Ctrl Pts',(12.9419577317687,9.96617502738866,4.99773406662709));
#11207=CARTESIAN_POINT('Ctrl Pts',(12.9420873152149,9.99939266312408,4.99592528053768));
#11208=CARTESIAN_POINT('Ctrl Pts',(12.9447203589281,9.99816149350058,5.75407471946233));
#11209=CARTESIAN_POINT('Ctrl Pts',(12.9497104259152,10.538897567902,5.72472844693841));
#11210=CARTESIAN_POINT('Ctrl Pts',(13.445663016072,11.770362488044,5.65833512523815));
#11211=CARTESIAN_POINT('Ctrl Pts',(15.5229818972268,12.3716681799822,5.55489475436157));
#11212=CARTESIAN_POINT('Ctrl Pts',(17.2762330137476,10.8468076994282,5.44375360683255));
#11213=CARTESIAN_POINT('Ctrl Pts',(16.9459104193154,8.54681293441946,5.33261245930352));
#11214=CARTESIAN_POINT('Ctrl Pts',(14.8343783616792,7.57700815405708,5.22147131177451));
#11215=CARTESIAN_POINT('Ctrl Pts',(13.1970787562676,8.61966030426231,5.12862539849411));
#11216=CARTESIAN_POINT('Ctrl Pts',(12.9487124143475,9.65288887362781,5.07282653439004));
#11217=CARTESIAN_POINT('Ctrl Pts',(12.9486078680663,10.0000693726643,5.05407471946232));
#11218=CARTESIAN_POINT('Origin',(15.,10.,9.54592528053767));
#11219=CARTESIAN_POINT('',(12.9425629288878,10.0010699703231,6.45407471946232));
#11220=CARTESIAN_POINT('',(12.9484827731942,9.99946914088102,6.39592528053768));
#11221=CARTESIAN_POINT('',(12.94525,10.0000000000001,9.54592528053767));
#11222=CARTESIAN_POINT('Ctrl Pts',(12.9484827731942,9.99946914088102,6.39592528053768));
#11223=CARTESIAN_POINT('Ctrl Pts',(12.9493514564268,10.3751323293684,6.3756319900765));
#11224=CARTESIAN_POINT('Ctrl Pts',(13.2280330016817,11.4377987966319,6.31829165043898));
#11225=CARTESIAN_POINT('Ctrl Pts',(14.9350675106875,12.4277778414421,6.22390426162511));
#11226=CARTESIAN_POINT('Ctrl Pts',(17.0045372308406,11.3711864275124,6.1127631140961));
#11227=CARTESIAN_POINT('Ctrl Pts',(17.2391328194089,9.05946509552617,6.00162196656707));
#11228=CARTESIAN_POINT('Ctrl Pts',(15.424114751786,7.608672268086,5.89048081903805));
#11229=CARTESIAN_POINT('Ctrl Pts',(13.4040950392535,8.28542469052011,5.78858192369492));
#11230=CARTESIAN_POINT('Ctrl Pts',(12.9502202013615,9.48899468762855,5.72373007752813));
#11231=CARTESIAN_POINT('Ctrl Pts',(12.9455805553419,10.0018769103914,5.69592528053768));
#11232=CARTESIAN_POINT('Ctrl Pts',(12.9425629288878,10.0010699703231,6.45407471946232));
#11233=CARTESIAN_POINT('Ctrl Pts',(12.9421730677846,10.0626339108422,6.45072445783945));
#11234=CARTESIAN_POINT('Ctrl Pts',(12.9726042727645,10.8045784977884,6.41032714704025));
#11235=CARTESIAN_POINT('Ctrl Pts',(13.8720874462699,12.1508444526632,6.33288278706471));
#11236=CARTESIAN_POINT('Ctrl Pts',(16.1953904039119,12.1140865945272,6.22174163953568));
#11237=CARTESIAN_POINT('Ctrl Pts',(17.4244805427636,10.1421770013196,6.11060049200667));
#11238=CARTESIAN_POINT('Ctrl Pts',(16.4342968937075,8.04012443367538,5.99945934447764));
#11239=CARTESIAN_POINT('Ctrl Pts',(14.1312146531314,7.73206435471271,5.88831819694863));
#11240=CARTESIAN_POINT('Ctrl Pts',(13.0215193522343,9.03317276281873,5.80652332194352));
#11241=CARTESIAN_POINT('Ctrl Pts',(12.9434109118316,9.85626654812099,5.76177549611475));
#11242=CARTESIAN_POINT('Ctrl Pts',(12.9447203589281,9.99816149350058,5.75407471946233));
#11243=CARTESIAN_POINT('Origin',(15.,10.,9.54592528053767));
#11244=CARTESIAN_POINT('',(12.9479405474349,10.0011587877502,7.15407471946232));
#11245=CARTESIAN_POINT('',(12.9436341942584,9.99839713117394,7.09592528053768));
#11246=CARTESIAN_POINT('',(12.94525,10.0000000000001,9.54592528053767));
#11247=CARTESIAN_POINT('Ctrl Pts',(12.9436341942584,9.99839713117394,7.09592528053768));
#11248=CARTESIAN_POINT('Ctrl Pts',(12.9485802607195,10.5751617788476,7.0645809518012));
#11249=CARTESIAN_POINT('Ctrl Pts',(13.5024258197495,11.8419530434235,6.99618957388839));
#11250=CARTESIAN_POINT('Ctrl Pts',(15.6497677286939,12.3401097288481,6.89075114679923));
#11251=CARTESIAN_POINT('Ctrl Pts',(17.3184787798211,10.7231732227644,6.77960999927021));
#11252=CARTESIAN_POINT('Ctrl Pts',(16.864945940343,8.44426865073882,6.66846885174118));
#11253=CARTESIAN_POINT('Ctrl Pts',(14.7043153597183,7.58942105489702,6.55732770421218));
#11254=CARTESIAN_POINT('Ctrl Pts',(13.1594333615178,8.69431383299048,6.46647984714433));
#11255=CARTESIAN_POINT('Ctrl Pts',(12.9477656046647,9.68932868188927,6.41267903925283));
#11256=CARTESIAN_POINT('Ctrl Pts',(12.9484827731942,9.99946914088102,6.39592528053768));
#11257=CARTESIAN_POINT('Ctrl Pts',(12.9479405474349,10.0011587877502,7.15407471946232));
#11258=CARTESIAN_POINT('Ctrl Pts',(12.9465638731556,10.2675785025657,7.13967341956416));
#11259=CARTESIAN_POINT('Ctrl Pts',(13.1185705249126,11.2176540004845,7.08822507048966));
#11260=CARTESIAN_POINT('Ctrl Pts',(14.552316547407,12.3870127270114,6.99972967223883));
#11261=CARTESIAN_POINT('Ctrl Pts',(16.7627159052523,11.6706763447836,6.8885885247098));
#11262=CARTESIAN_POINT('Ctrl Pts',(17.359610496679,9.42504513942049,6.77744737718079));
#11263=CARTESIAN_POINT('Ctrl Pts',(15.796602835303,7.70571713781293,6.66630622965176));
#11264=CARTESIAN_POINT('Ctrl Pts',(13.5735166221464,8.07500088427441,6.55851534374561));
#11265=CARTESIAN_POINT('Ctrl Pts',(12.9464841351245,9.38186249993724,6.48777150701579));
#11266=CARTESIAN_POINT('Ctrl Pts',(12.9425629288878,10.0010699703231,6.45407471946232));
#11267=CARTESIAN_POINT('Origin',(15.,10.,9.54592528053767));
#11268=CARTESIAN_POINT('',(12.9473113968994,9.99752941021421,7.85407471946233));
#11269=CARTESIAN_POINT('',(12.9434528818545,10.0014882284141,7.79592528053768));
#11270=CARTESIAN_POINT('',(12.94525,10.0000000000001,9.54592528053767));
#11271=CARTESIAN_POINT('',(14.4698297828114,8.01482567432828,8.));
#11272=CARTESIAN_POINT('Ctrl Pts',(14.4698297828114,8.01482567432828,8.));
#11273=CARTESIAN_POINT('Ctrl Pts',(13.8096927451188,8.1911250512252,7.96295295082366));
#11274=CARTESIAN_POINT('Ctrl Pts',(13.0749952948832,8.88701044345236,7.91431119064444));
#11275=CARTESIAN_POINT('Ctrl Pts',(12.9456877182649,9.7832841399949,7.86566943046521));
#11276=CARTESIAN_POINT('Ctrl Pts',(12.9473113968994,9.99752941021421,7.85407471946233));
#11277=CARTESIAN_POINT('',(15.5312698928193,8.01125028009066,8.));
#11278=CARTESIAN_POINT('Origin',(15.,10.,8.));
#11279=CARTESIAN_POINT('Ctrl Pts',(15.531270276981,8.01124903105919,8.));
#11280=CARTESIAN_POINT('Ctrl Pts',(14.8865857166431,7.83988501971335,7.96367382485347));
#11281=CARTESIAN_POINT('Ctrl Pts',(13.5069335921707,8.15949860066886,7.89564891836603));
#11282=CARTESIAN_POINT('Ctrl Pts',(12.9483221305924,9.41848319233778,7.82762401187859));
#11283=CARTESIAN_POINT('Ctrl Pts',(12.9434528818545,10.0014882284141,7.79592528053768));
#11284=CARTESIAN_POINT('Origin',(-15.,-10.,9.54592528053767));
#11285=CARTESIAN_POINT('',(-17.0517816873057,-9.99918029423424,0.15407471946232));
#11286=CARTESIAN_POINT('',(-17.0565583212302,-10.0015648221723,0.0959252805376758));
#11287=CARTESIAN_POINT('',(-17.05475,-9.99999999999991,9.54592528053767));
#11288=CARTESIAN_POINT('',(-16.3390017195986,-8.44145197141315,1.11022302462516E-15));
#11289=CARTESIAN_POINT('Ctrl Pts',(-17.0565583212302,-10.0015648221723,
0.0959252805376758));
#11290=CARTESIAN_POINT('Ctrl Pts',(-17.0518107016117,-9.41495008139905,
0.0639501870251164));
#11291=CARTESIAN_POINT('Ctrl Pts',(-16.7863171109465,-8.82575586659747,
0.0319750935125572));
#11292=CARTESIAN_POINT('Ctrl Pts',(-16.3390017195986,-8.44145197141311,
-2.22044604925031E-15));
#11293=CARTESIAN_POINT('',(-15.3842288288255,-7.97768903459251,4.89463757827447E-16));
#11294=CARTESIAN_POINT('Origin',(-15.,-10.,0.));
#11295=CARTESIAN_POINT('Ctrl Pts',(-17.0517816873057,-9.99918029423424,
0.15407471946232));
#11296=CARTESIAN_POINT('Ctrl Pts',(-17.0529881094183,-9.72108671039038,
0.139042654788077));
#11297=CARTESIAN_POINT('Ctrl Pts',(-16.8731950448097,-8.77236588328783,
0.0876844149673042));
#11298=CARTESIAN_POINT('Ctrl Pts',(-16.0394219710344,-8.10301220682191,
0.0363261751465313));
#11299=CARTESIAN_POINT('Ctrl Pts',(-15.3842290239278,-7.97768774796568,
8.9812597463268E-16));
#11300=CARTESIAN_POINT('Origin',(-15.,-10.,9.54592528053767));
#11301=CARTESIAN_POINT('',(-17.0535052914424,-10.0017735080204,0.854074719462321));
#11302=CARTESIAN_POINT('',(-17.0562189577482,-9.9983358962701,0.795925280537676));
#11303=CARTESIAN_POINT('',(-17.05475,-9.99999999999991,9.54592528053767));
#11304=CARTESIAN_POINT('Ctrl Pts',(-17.0562189577482,-9.9983358962701,0.795925280537676));
#11305=CARTESIAN_POINT('Ctrl Pts',(-17.0571797200526,-9.88829543020703,
0.789946197926163));
#11306=CARTESIAN_POINT('Ctrl Pts',(-16.9990976027996,-9.09745400255305,
0.74692006613831));
#11307=CARTESIAN_POINT('Ctrl Pts',(-15.9729748140483,-7.77487725906727,
0.666846885174117));
#11308=CARTESIAN_POINT('Ctrl Pts',(-13.6580450846071,-7.97554008402429,
0.555705737645098));
#11309=CARTESIAN_POINT('Ctrl Pts',(-12.5715926480149,-10.0300833696701,
0.444564590116077));
#11310=CARTESIAN_POINT('Ctrl Pts',(-13.7078055175393,-12.0555949236832,
0.333423442587058));
#11311=CARTESIAN_POINT('Ctrl Pts',(-16.0272313718098,-12.2024171088693,
0.222282295058038));
#11312=CARTESIAN_POINT('Ctrl Pts',(-17.0090838666329,-10.8667907385836,
0.143116241041577));
#11313=CARTESIAN_POINT('Ctrl Pts',(-17.0573113985028,-10.0946148692583,
0.100997236201457));
#11314=CARTESIAN_POINT('Ctrl Pts',(-17.0565583212302,-10.0015648221723,
0.0959252805376758));
#11315=CARTESIAN_POINT('Ctrl Pts',(-17.0535052914424,-10.0017735080204,
0.854074719462321));
#11316=CARTESIAN_POINT('Ctrl Pts',(-17.0495358857753,-9.52010780339371,
0.827991616512785));
#11317=CARTESIAN_POINT('Ctrl Pts',(-16.6400833000123,-8.34823531025937,
0.764861464386909));
#11318=CARTESIAN_POINT('Ctrl Pts',(-14.687180849695,-7.59155940883828,0.664684263084691));
#11319=CARTESIAN_POINT('Ctrl Pts',(-12.8068360000695,-8.95675512341312,
0.553543115555673));
#11320=CARTESIAN_POINT('Ctrl Pts',(-12.9341202906761,-11.2767116091318,
0.442401968026652));
#11321=CARTESIAN_POINT('Ctrl Pts',(-14.9522479049698,-12.4283740802081,
0.331260820497633));
#11322=CARTESIAN_POINT('Ctrl Pts',(-16.7355221426696,-11.5014784845208,
0.235151737642855));
#11323=CARTESIAN_POINT('Ctrl Pts',(-17.050014839924,-10.4064580748405,0.176089703964417));
#11324=CARTESIAN_POINT('Ctrl Pts',(-17.0517816873057,-9.99918029423424,
0.15407471946232));
#11325=CARTESIAN_POINT('Origin',(-15.,-10.,9.54592528053767));
#11326=CARTESIAN_POINT('',(-17.0581309722196,-9.99997008132667,1.55407471946232));
#11327=CARTESIAN_POINT('',(-17.0514806312403,-9.99955010506969,1.49592528053768));
#11328=CARTESIAN_POINT('',(-17.05475,-9.99999999999991,9.54592528053767));
#11329=CARTESIAN_POINT('Ctrl Pts',(-17.0514806312403,-9.99955010506969,
1.49592528053768));
#11330=CARTESIAN_POINT('Ctrl Pts',(-17.0520975200814,-9.6842796794923,1.47889515965087));
#11331=CARTESIAN_POINT('Ctrl Pts',(-16.8355232859291,-8.68397857454396,
1.42481798958773));
#11332=CARTESIAN_POINT('Ctrl Pts',(-15.2777376918069,-7.58728937837554,
1.33369377034824));
#11333=CARTESIAN_POINT('Ctrl Pts',(-13.1235278364479,-8.45818684891592,
1.22255262281922));
#11334=CARTESIAN_POINT('Ctrl Pts',(-12.686968390135,-10.7404136399833,1.1114114752902));
#11335=CARTESIAN_POINT('Ctrl Pts',(-14.367662797513,-12.344866918125,1.00027032776118));
#11336=CARTESIAN_POINT('Ctrl Pts',(-16.5056253516517,-11.8321284649118,
0.895108262843669));
#11337=CARTESIAN_POINT('Ctrl Pts',(-17.0512267318348,-10.5701181817067,
0.826993247102503));
#11338=CARTESIAN_POINT('Ctrl Pts',(-17.0562189577482,-9.9983358962701,0.795925280537676));
#11339=CARTESIAN_POINT('Ctrl Pts',(-17.0581309722196,-9.99997008132667,
1.55407471946232));
#11340=CARTESIAN_POINT('Ctrl Pts',(-17.0581313153895,-9.99837112568893,
1.55398762741383));
#11341=CARTESIAN_POINT('Ctrl Pts',(-17.0574055017633,-9.31661179721689,
1.516853486189));
#11342=CARTESIAN_POINT('Ctrl Pts',(-16.3123135839388,-7.95643629520889,
1.44267229578783));
#11343=CARTESIAN_POINT('Ctrl Pts',(-13.9947483624482,-7.78916489875036,
1.33153114825881));
#11344=CARTESIAN_POINT('Ctrl Pts',(-12.5973498364434,-9.64560634071132,
1.22039000072979));
#11345=CARTESIAN_POINT('Ctrl Pts',(-13.3992440433914,-11.826442250177,1.10924885320077));
#11346=CARTESIAN_POINT('Ctrl Pts',(-15.6664035468934,-12.3354318728424,
0.998107705671752));
#11347=CARTESIAN_POINT('Ctrl Pts',(-16.934658910805,-11.0888971028013,0.913049661092267));
#11348=CARTESIAN_POINT('Ctrl Pts',(-17.0551738180119,-10.204240097024,0.865038665689124));
#11349=CARTESIAN_POINT('Ctrl Pts',(-17.0535052914424,-10.0017735080204,
0.854074719462321));
#11350=CARTESIAN_POINT('Origin',(-15.,-10.,9.54592528053767));
#11351=CARTESIAN_POINT('',(-17.0534183899706,-9.99824587165492,2.25407471946232));
#11352=CARTESIAN_POINT('',(-17.0545721863858,-10.0018793627325,2.19592528053768));
#11353=CARTESIAN_POINT('',(-17.05475,-9.99999999999991,9.54592528053767));
#11354=CARTESIAN_POINT('Ctrl Pts',(-17.0545721863858,-10.0018793627325,
2.19592528053768));
#11355=CARTESIAN_POINT('Ctrl Pts',(-17.0498496452687,-9.48399778682363,
2.16784412137558));
#11356=CARTESIAN_POINT('Ctrl Pts',(-16.5885931819089,-8.27539049526638,
2.10271591303714));
#11357=CARTESIAN_POINT('Ctrl Pts',(-14.5581012599229,-7.61189486585896,
2.00054065552235));
#11358=CARTESIAN_POINT('Ctrl Pts',(-12.7539300664426,-9.07615430524727,
1.88939950799334));
#11359=CARTESIAN_POINT('Ctrl Pts',(-13.0057225272674,-11.3860658425327,
1.77825836046431));
#11360=CARTESIAN_POINT('Ctrl Pts',(-15.0829976689147,-12.4272269759234,
1.6671172129353));
#11361=CARTESIAN_POINT('Ctrl Pts',(-16.7776412533276,-11.4275083697971,
1.57300618629308));
#11362=CARTESIAN_POINT('Ctrl Pts',(-17.0507555500869,-10.3701138575256,
1.51594220882721));
#11363=CARTESIAN_POINT('Ctrl Pts',(-17.0514806312403,-9.99955010506969,
1.49592528053768));
#11364=CARTESIAN_POINT('Ctrl Pts',(-17.0534183899706,-9.99824587165492,
2.25407471946232));
#11365=CARTESIAN_POINT('Ctrl Pts',(-17.0550897983517,-9.79253954287702,
2.24293658913854));
#11366=CARTESIAN_POINT('Ctrl Pts',(-16.932137008376,-8.90457640973076,2.19475140963841));
#11367=CARTESIAN_POINT('Ctrl Pts',(-15.6554439913718,-7.66147180407228,
2.10951918096195));
#11368=CARTESIAN_POINT('Ctrl Pts',(-13.3906939345767,-8.18108411896286,
1.99837803343293));
#11369=CARTESIAN_POINT('Ctrl Pts',(-12.5990390076834,-10.3656601528754,
1.88723688590391));
#11370=CARTESIAN_POINT('Ctrl Pts',(-14.0051288824869,-12.2155252739355,
1.77609573837489));
#11371=CARTESIAN_POINT('Ctrl Pts',(-16.3200689326647,-12.0375258716092,
1.66504168289436));
#11372=CARTESIAN_POINT('Ctrl Pts',(-17.0579853384182,-10.6785318196738,
1.59103467659017));
#11373=CARTESIAN_POINT('Ctrl Pts',(-17.0581309722196,-9.99997008132667,
1.55407471946232));
#11374=CARTESIAN_POINT('Origin',(-15.,-10.,9.54592528053767));
#11375=CARTESIAN_POINT('',(-17.0519256455684,-10.0010517737669,2.95407471946232));
#11376=CARTESIAN_POINT('',(-17.0578444882157,-9.99930470806554,2.89592528053768));
#11377=CARTESIAN_POINT('',(-17.05475,-9.99999999999991,9.54592528053767));
#11378=CARTESIAN_POINT('Ctrl Pts',(-17.0578444882157,-9.99930470806554,
2.89592528053768));
#11379=CARTESIAN_POINT('Ctrl Pts',(-17.0580128383109,-9.96100841827086,
2.89384013227662));
#11380=CARTESIAN_POINT('Ctrl Pts',(-17.0396873848621,-9.24246223468361,
2.85470793483923));
#11381=CARTESIAN_POINT('Ctrl Pts',(-16.2005167846521,-7.88882016989784,
2.77852868822549));
#11382=CARTESIAN_POINT('Ctrl Pts',(-13.8773094527777,-7.84642465758702,
2.66738754069648));
#11383=CARTESIAN_POINT('Ctrl Pts',(-12.5817686609856,-9.7753268677064,2.55624639316746));
#11384=CARTESIAN_POINT('Ctrl Pts',(-13.4997812308935,-11.9098859856603,
2.44510524563844));
#11385=CARTESIAN_POINT('Ctrl Pts',(-15.7910347483105,-12.2962109712173,
2.33396409810941));
#11386=CARTESIAN_POINT('Ctrl Pts',(-16.962241421697,-11.0141261502186,2.2509041097425));
#11387=CARTESIAN_POINT('Ctrl Pts',(-17.0560800224405,-10.1672311284198,
2.20489117055192));
#11388=CARTESIAN_POINT('Ctrl Pts',(-17.0545721863858,-10.0018793627325,
2.19592528053768));
#11389=CARTESIAN_POINT('Ctrl Pts',(-17.0519256455684,-10.0010517737669,
2.95407471946232));
#11390=CARTESIAN_POINT('Ctrl Pts',(-17.0500218558526,-9.59049710140644,
2.93188555086324));
#11391=CARTESIAN_POINT('Ctrl Pts',(-16.7315452820547,-8.49176055139755,
2.87264933308782));
#11392=CARTESIAN_POINT('Ctrl Pts',(-14.9409585972601,-7.57207185286643,
2.77636606613607));
#11393=CARTESIAN_POINT('Ctrl Pts',(-12.9281030287572,-8.73289151373681,
2.66522491860704));
#11394=CARTESIAN_POINT('Ctrl Pts',(-12.8117800332785,-11.0535721874087,
2.55408377107803));
#11395=CARTESIAN_POINT('Ctrl Pts',(-14.6984670829124,-12.4098545333209,
2.442942623549));
#11396=CARTESIAN_POINT('Ctrl Pts',(-16.6444282867541,-11.6453952227051,
2.34293960634378));
#11397=CARTESIAN_POINT('Ctrl Pts',(-17.0495304498177,-10.4767488541872,
2.27998363831488));
#11398=CARTESIAN_POINT('Ctrl Pts',(-17.0534183899706,-9.99824587165492,
2.25407471946232));
#11399=CARTESIAN_POINT('Origin',(-15.,-10.,9.54592528053767));
#11400=CARTESIAN_POINT('',(-17.057256555318,-10.001191465967,3.65407471946232));
#11401=CARTESIAN_POINT('',(-17.0525172682208,-9.99855769014068,3.59592528053768));
#11402=CARTESIAN_POINT('',(-17.05475,-9.99999999999991,9.54592528053767));
#11403=CARTESIAN_POINT('Ctrl Pts',(-17.0525172682208,-9.99855769014068,
3.59592528053768));
#11404=CARTESIAN_POINT('Ctrl Pts',(-17.0540904425641,-9.75568132341078,
3.58278909400133));
#11405=CARTESIAN_POINT('Ctrl Pts',(-16.901884557562,-8.82974572708431,3.53260585828864));
#11406=CARTESIAN_POINT('Ctrl Pts',(-15.5287351392234,-7.62960763240948,
3.44537557339961));
#11407=CARTESIAN_POINT('Ctrl Pts',(-13.2952058270941,-8.27026081396139,
3.33423442587059));
#11408=CARTESIAN_POINT('Ctrl Pts',(-12.6221777004152,-10.4942488597207,
3.22309327834158));
#11409=CARTESIAN_POINT('Ctrl Pts',(-14.1257140976557,-12.2658210399188,
3.11195213081255));
#11410=CARTESIAN_POINT('Ctrl Pts',(-16.3863146130996,-11.9690249555389,
3.00289613154459));
#11411=CARTESIAN_POINT('Ctrl Pts',(-17.0550217444047,-10.6414226400287,
2.93088718145296));
#11412=CARTESIAN_POINT('Ctrl Pts',(-17.0578444882157,-9.99930470806554,
2.89592528053768));
#11413=CARTESIAN_POINT('Ctrl Pts',(-17.057256555318,-10.001191465967,3.65407471946232));
#11414=CARTESIAN_POINT('Ctrl Pts',(-17.0530396235064,-9.39023283914347,
3.62083451258795));
#11415=CARTESIAN_POINT('Ctrl Pts',(-16.4406464494583,-8.09100504150255,
3.55054725653724));
#11416=CARTESIAN_POINT('Ctrl Pts',(-14.2316631334124,-7.69609474266784,
3.44321295131019));
#11417=CARTESIAN_POINT('Ctrl Pts',(-12.647638657407,-9.39608188535426,3.33207180378117));
#11418=CARTESIAN_POINT('Ctrl Pts',(-13.2168727518909,-11.6488717938068,
3.22093065625215));
#11419=CARTESIAN_POINT('Ctrl Pts',(-15.4183110319232,-12.3923496516694,
3.10978950872312));
#11420=CARTESIAN_POINT('Ctrl Pts',(-16.873776480767,-11.2347337715044,3.02083752979319));
#11421=CARTESIAN_POINT('Ctrl Pts',(-17.0532004243018,-10.2759594281538,
2.96893260003959));
#11422=CARTESIAN_POINT('Ctrl Pts',(-17.0519256455684,-10.0010517737669,
2.95407471946232));
#11423=CARTESIAN_POINT('Origin',(-15.,-10.,9.54592528053767));
#11424=CARTESIAN_POINT('',(-17.0555344808246,-9.99819734174245,4.35407471946232));
#11425=CARTESIAN_POINT('',(-17.0526295118996,-10.0014953654714,4.29592528053768));
#11426=CARTESIAN_POINT('',(-17.05475,-9.99999999999991,9.54592528053767));
#11427=CARTESIAN_POINT('Ctrl Pts',(-17.0526295118996,-10.0014953654714,
4.29592528053768));
#11428=CARTESIAN_POINT('Ctrl Pts',(-17.049615748339,-9.55435663972008,4.27173805572604));
#11429=CARTESIAN_POINT('Ctrl Pts',(-16.6860607259798,-8.41788413676447,
4.21050378173805));
#11430=CARTESIAN_POINT('Ctrl Pts',(-14.8104759432562,-7.57876034732949,
4.11222245857374));
#11431=CARTESIAN_POINT('Ctrl Pts',(-12.8629591929671,-8.84614671087597,
4.00108131104471));
#11432=CARTESIAN_POINT('Ctrl Pts',(-12.8716051077936,-11.1697247567595,
3.88994016351569));
#11433=CARTESIAN_POINT('Ctrl Pts',(-14.8284995591272,-12.4225830063246,
3.77879901598667));
#11434=CARTESIAN_POINT('Ctrl Pts',(-16.6925314739129,-11.571923493464,3.680794054994));
#11435=CARTESIAN_POINT('Ctrl Pts',(-17.0496537312629,-10.4406482030388,
3.61983614317767));
#11436=CARTESIAN_POINT('Ctrl Pts',(-17.0525172682208,-9.99855769014068,
3.59592528053768));
#11437=CARTESIAN_POINT('Ctrl Pts',(-17.0555344808246,-9.99819734174245,
4.35407471946232));
#11438=CARTESIAN_POINT('Ctrl Pts',(-17.0567584155299,-9.86475790704786,
4.346830523489));
#11439=CARTESIAN_POINT('Ctrl Pts',(-16.9841133186881,-9.05023169781548,
4.30253927833933));
#11440=CARTESIAN_POINT('Ctrl Pts',(-15.8966028265696,-7.74291684984371,
4.22120098401332));
#11441=CARTESIAN_POINT('Ctrl Pts',(-13.5899069966017,-8.02263845058788,
4.11005983648432));
#11442=CARTESIAN_POINT('Ctrl Pts',(-12.5739545527748,-10.1123586370691,
3.99891868895528));
#11443=CARTESIAN_POINT('Ctrl Pts',(-13.7787081956621,-12.0992301693682,
3.88777754142627));
#11444=CARTESIAN_POINT('Ctrl Pts',(-16.1013840714784,-12.1645493993947,
3.77663639389725));
#11445=CARTESIAN_POINT('Ctrl Pts',(-17.0227508013064,-10.8215719974621,
3.6987354532426));
#11446=CARTESIAN_POINT('Ctrl Pts',(-17.0577395003991,-10.0711616425707,
3.65788156176429));
#11447=CARTESIAN_POINT('Ctrl Pts',(-17.057256555318,-10.001191465967,3.65407471946232));
#11448=CARTESIAN_POINT('Origin',(-15.,-10.,9.54592528053767));
#11449=CARTESIAN_POINT('',(-17.0513922996156,-9.99993062733026,5.05407471946232));
#11450=CARTESIAN_POINT('',(-17.0579125370942,-10.0006073368323,4.99592528053768));
#11451=CARTESIAN_POINT('',(-17.05475,-9.99999999999991,9.54592528053767));
#11452=CARTESIAN_POINT('Ctrl Pts',(-17.0579125370942,-10.0006073368323,
4.99592528053768));
#11453=CARTESIAN_POINT('Ctrl Pts',(-17.0553880289355,-9.3534707240389,4.96068701745074));
#11454=CARTESIAN_POINT('Ctrl Pts',(-16.3773572422904,-8.02142236710827,
4.88840170518746));
#11455=CARTESIAN_POINT('Ctrl Pts',(-14.1088765326179,-7.74074795791574,
4.77906934374786));
#11456=CARTESIAN_POINT('Ctrl Pts',(-12.6185654451633,-9.52346009110162,
4.66792819621883));
#11457=CARTESIAN_POINT('Ctrl Pts',(-13.3081253972587,-11.7423780164876,
4.55678704868982));
#11458=CARTESIAN_POINT('Ctrl Pts',(-15.5463604710685,-12.3663919919164,
4.44564590116079));
#11459=CARTESIAN_POINT('Ctrl Pts',(-16.9062187021531,-11.1599029697348,
4.35869197844342));
#11460=CARTESIAN_POINT('Ctrl Pts',(-17.0542318648098,-10.2392293562288,
4.30878510490238));
#11461=CARTESIAN_POINT('Ctrl Pts',(-17.0526295118996,-10.0014953654714,
4.29592528053768));
#11462=CARTESIAN_POINT('Ctrl Pts',(-17.0513922996156,-9.99993062733025,
5.05407471946232));
#11463=CARTESIAN_POINT('Ctrl Pts',(-17.0514943003483,-9.66120346411399,
5.03577948521371));
#11464=CARTESIAN_POINT('Ctrl Pts',(-16.8117677005034,-8.63670450547305,
4.98043720178875));
#11465=CARTESIAN_POINT('Ctrl Pts',(-15.1953985278237,-7.57922731532253,
4.88804786918744));
#11466=CARTESIAN_POINT('Ctrl Pts',(-13.0721026532078,-8.52299871511589,
4.77690672165843));
#11467=CARTESIAN_POINT('Ctrl Pts',(-12.7135277889139,-10.818758696566,4.6657655741294));
#11468=CARTESIAN_POINT('Ctrl Pts',(-14.4478991890863,-12.3650593375113,
4.55462442660038));
#11469=CARTESIAN_POINT('Ctrl Pts',(-16.5416550956139,-11.7867973751395,
4.45072747504469));
#11470=CARTESIAN_POINT('Ctrl Pts',(-17.0504991744238,-10.5471714305632,
4.38387757266534));
#11471=CARTESIAN_POINT('Ctrl Pts',(-17.0555344808246,-9.99819734174245,
4.35407471946232));
#11472=CARTESIAN_POINT('Origin',(-15.,-10.,9.54592528053767));
#11473=CARTESIAN_POINT('',(-17.0552798090643,-10.0018385066652,5.75407471946232));
#11474=CARTESIAN_POINT('',(-17.0544192972179,-9.99812308974333,5.69592528053768));
#11475=CARTESIAN_POINT('',(-17.05475,-9.99999999999991,9.54592528053767));
#11476=CARTESIAN_POINT('Ctrl Pts',(-17.0544192972179,-9.99812308974333,
5.69592528053768));
#11477=CARTESIAN_POINT('Ctrl Pts',(-17.0559615050427,-9.82764220092783,
5.68668302835179));
#11478=CARTESIAN_POINT('Ctrl Pts',(-16.9585687134996,-8.9755360511576,5.64039372698956));
#11479=CARTESIAN_POINT('Ctrl Pts',(-15.7739249147585,-7.69796588935184,
5.55705737645099));
#11480=CARTESIAN_POINT('Ctrl Pts',(-13.4856097934235,-8.10133122228054,
5.44591622892198));
#11481=CARTESIAN_POINT('Ctrl Pts',(-12.583507594572,-10.2426628903111,5.33477508139295));
#11482=CARTESIAN_POINT('Ctrl Pts',(-13.8933670056466,-12.161870541709,5.22363393386393));
#11483=CARTESIAN_POINT('Ctrl Pts',(-16.2161945081267,-12.1021873709018,
5.11249278633491));
#11484=CARTESIAN_POINT('Ctrl Pts',(-17.0422606408936,-10.7472711004341,
5.03658990189283));
#11485=CARTESIAN_POINT('Ctrl Pts',(-17.0580421205311,-10.0338249701837,
4.99773406662709));
#11486=CARTESIAN_POINT('Ctrl Pts',(-17.0579125370942,-10.0006073368323,
4.99592528053768));
#11487=CARTESIAN_POINT('Ctrl Pts',(-17.0552798090643,-10.0018385066652,
5.75407471946232));
#11488=CARTESIAN_POINT('Ctrl Pts',(-17.05028974167,-9.46110238806226,5.72472844693841));
#11489=CARTESIAN_POINT('Ctrl Pts',(-16.5543371109916,-8.2296373672222,5.65833512523816));
#11490=CARTESIAN_POINT('Ctrl Pts',(-14.4770180600175,-7.62833162617035,
5.55489475436157));
#11491=CARTESIAN_POINT('Ctrl Pts',(-12.7237668001956,-9.15319223134576,
5.44375360683254));
#11492=CARTESIAN_POINT('Ctrl Pts',(-13.0540894216228,-11.4531871843689,
5.33261245930352));
#11493=CARTESIAN_POINT('Ctrl Pts',(-15.1656216518599,-12.4229920439975,
5.22147131177451));
#11494=CARTESIAN_POINT('Ctrl Pts',(-16.8029213911039,-11.380339808568,5.1286253984941));
#11495=CARTESIAN_POINT('Ctrl Pts',(-17.0512877533257,-10.3471111547456,
5.07282653439004));
#11496=CARTESIAN_POINT('Ctrl Pts',(-17.0513922996156,-9.99993062733025,
5.05407471946232));
#11497=CARTESIAN_POINT('Origin',(-15.,-10.,9.54592528053767));
#11498=CARTESIAN_POINT('',(-17.0574372391259,-9.99893002996487,6.45407471946233));
#11499=CARTESIAN_POINT('',(-17.0515170795977,-10.0005308591959,6.39592528053768));
#11500=CARTESIAN_POINT('',(-17.05475,-9.99999999999991,9.54592528053767));
#11501=CARTESIAN_POINT('Ctrl Pts',(-17.0515170795977,-10.0005308591959,
6.39592528053768));
#11502=CARTESIAN_POINT('Ctrl Pts',(-17.0506483964156,-9.62486769760656,
6.3756319900765));
#11503=CARTESIAN_POINT('Ctrl Pts',(-16.771966871107,-8.56220130633378,6.31829165043898));
#11504=CARTESIAN_POINT('Ctrl Pts',(-15.0649324846807,-7.5722223329502,6.22390426162511));
#11505=CARTESIAN_POINT('Ctrl Pts',(-12.995462913005,-8.62881367080874,6.11276311409609));
#11506=CARTESIAN_POINT('Ctrl Pts',(-12.7608673412954,-10.9405348370204,
6.00162196656707));
#11507=CARTESIAN_POINT('Ctrl Pts',(-14.5758852786477,-12.3913275602698,
5.89048081903805));
#11508=CARTESIAN_POINT('Ctrl Pts',(-16.5959048462141,-11.7145751864396,
5.78858192369492));
#11509=CARTESIAN_POINT('Ctrl Pts',(-17.0497796515317,-10.5110052757004,
5.72373007752813));
#11510=CARTESIAN_POINT('Ctrl Pts',(-17.0544192972179,-9.99812308974333,
5.69592528053768));
#11511=CARTESIAN_POINT('Ctrl Pts',(-17.0574372391259,-9.99893002996487,
6.45407471946233));
#11512=CARTESIAN_POINT('Ctrl Pts',(-17.0578271002392,-9.93736608446989,
6.45072445783946));
#11513=CARTESIAN_POINT('Ctrl Pts',(-17.0273958925505,-9.19542143745478,
6.41032714704025));
#11514=CARTESIAN_POINT('Ctrl Pts',(-16.1279126463626,-7.84915537048691,
6.3328827870647));
#11515=CARTESIAN_POINT('Ctrl Pts',(-13.8046094981315,-7.88591323323186,
6.22174163953568));
#11516=CARTESIAN_POINT('Ctrl Pts',(-12.5755192591945,-9.85782298675155,
6.11060049200667));
#11517=CARTESIAN_POINT('Ctrl Pts',(-13.5657029889766,-11.9598757266924,
5.99945934447763));
#11518=CARTESIAN_POINT('Ctrl Pts',(-15.8687854179254,-12.2679358305796,
5.88831819694863));
#11519=CARTESIAN_POINT('Ctrl Pts',(-16.9784808094819,-10.9668273162222,
5.80652332194351));
#11520=CARTESIAN_POINT('Ctrl Pts',(-17.0565892562676,-10.1437334636437,
5.76177549611475));
#11521=CARTESIAN_POINT('Ctrl Pts',(-17.0552798090643,-10.0018385066652,
5.75407471946232));
#11522=CARTESIAN_POINT('Origin',(-15.,-10.,9.54592528053767));
#11523=CARTESIAN_POINT('',(-17.0520596215353,-9.99884120146076,7.15407471946233));
#11524=CARTESIAN_POINT('',(-17.0563656598722,-10.0016028745823,7.09592528053768));
#11525=CARTESIAN_POINT('',(-17.05475,-9.99999999999991,9.54592528053767));
#11526=CARTESIAN_POINT('Ctrl Pts',(-17.0563656598722,-10.0016028745823,
7.09592528053768));
#11527=CARTESIAN_POINT('Ctrl Pts',(-17.0514195939162,-9.42483826837157,
7.0645809518012));
#11528=CARTESIAN_POINT('Ctrl Pts',(-16.4975740702056,-8.15804707939392,
6.99618957388839));
#11529=CARTESIAN_POINT('Ctrl Pts',(-14.350232319384,-7.65989044479182,6.89075114679923));
#11530=CARTESIAN_POINT('Ctrl Pts',(-12.6815213858194,-9.27682682597027,
6.77960999927021));
#11531=CARTESIAN_POINT('Ctrl Pts',(-13.1350541938888,-11.5557312393606,
6.66846885174119));
#11532=CARTESIAN_POINT('Ctrl Pts',(-15.295684618859,-12.4105787711389,6.55732770421217));
#11533=CARTESIAN_POINT('Ctrl Pts',(-16.8405665064385,-11.3056860735596,
6.46647984714433));
#11534=CARTESIAN_POINT('Ctrl Pts',(-17.0522342480855,-10.3106712959811,
6.41267903925284));
#11535=CARTESIAN_POINT('Ctrl Pts',(-17.0515170795977,-10.0005308591959,
6.39592528053768));
#11536=CARTESIAN_POINT('Ctrl Pts',(-17.0520596215353,-9.99884120146076,
7.15407471946233));
#11537=CARTESIAN_POINT('Ctrl Pts',(-17.053436293058,-9.73242147652985,7.13967341956416));
#11538=CARTESIAN_POINT('Ctrl Pts',(-16.8814296172514,-8.78234594443343,
7.08822507048967));
#11539=CARTESIAN_POINT('Ctrl Pts',(-15.4476835001917,-7.61298704116733,
6.99972967223882));
#11540=CARTESIAN_POINT('Ctrl Pts',(-13.2372839439424,-8.32932353917012,
6.88858852470981));
#11541=CARTESIAN_POINT('Ctrl Pts',(-12.64038931445,-10.5749548961775,6.77744737718078));
#11542=CARTESIAN_POINT('Ctrl Pts',(-14.2033970972384,-12.2942830560246,
6.66630622965177));
#11543=CARTESIAN_POINT('Ctrl Pts',(-16.4264834956963,-11.9249992699025,
6.55851534374561));
#11544=CARTESIAN_POINT('Ctrl Pts',(-17.0535160327875,-10.618137550398,6.4877715070158));
#11545=CARTESIAN_POINT('Ctrl Pts',(-17.0574372391259,-9.99893002996487,
6.45407471946233));
#11546=CARTESIAN_POINT('Origin',(-15.,-10.,9.54592528053767));
#11547=CARTESIAN_POINT('',(-17.0526884867324,-10.0024695060038,7.85407471946233));
#11548=CARTESIAN_POINT('',(-17.0565470023424,-9.99851185632501,7.79592528053768));
#11549=CARTESIAN_POINT('',(-17.05475,-9.99999999999991,9.54592528053767));
#11550=CARTESIAN_POINT('',(-15.5301702171886,-11.9851743256717,8.));
#11551=CARTESIAN_POINT('Ctrl Pts',(-15.5301702171886,-11.9851743256717,
8.));
#11552=CARTESIAN_POINT('Ctrl Pts',(-16.1903072548812,-11.8088749487748,
7.96295295082366));
#11553=CARTESIAN_POINT('Ctrl Pts',(-16.9250043904129,-11.1129876322537,
7.91431119064444));
#11554=CARTESIAN_POINT('Ctrl Pts',(-17.0543121182783,-10.216714563805,7.86566943046521));
#11555=CARTESIAN_POINT('Ctrl Pts',(-17.0526884867324,-10.0024695060038,
7.85407471946233));
#11556=CARTESIAN_POINT('',(-14.4687304269164,-11.988749893056,8.));
#11557=CARTESIAN_POINT('Origin',(-15.,-10.,8.));
#11558=CARTESIAN_POINT('Ctrl Pts',(-14.4687300448211,-11.9887511357905,
8.));
#11559=CARTESIAN_POINT('Ctrl Pts',(-15.1134147663027,-12.1601152915704,
7.96367382485347));
#11560=CARTESIAN_POINT('Ctrl Pts',(-16.4930658496611,-11.8405006708346,
7.89564891836603));
#11561=CARTESIAN_POINT('Ctrl Pts',(-17.0516776590012,-10.5815167296829,
7.82762401187859));
#11562=CARTESIAN_POINT('Ctrl Pts',(-17.0565470023424,-9.99851185632501,
7.79592528053768));
#11563=CARTESIAN_POINT('Origin',(12.9142135623731,11.9142135623731,26.));
#11564=CARTESIAN_POINT('',(18.,6.82842712474619,28.));
#11565=CARTESIAN_POINT('',(12.8284271247462,12.,28.));
#11566=CARTESIAN_POINT('',(12.9142135623731,11.9142135623731,28.));
#11567=CARTESIAN_POINT('',(12.,10.,26.));
#11568=CARTESIAN_POINT('Origin',(12.8284271247462,12.,26.));
#11569=CARTESIAN_POINT('',(16.,6.,26.));
#11570=CARTESIAN_POINT('',(11.5,10.5,26.));
#11571=CARTESIAN_POINT('Origin',(18.,6.82842712474619,26.));
#11572=CARTESIAN_POINT('Origin',(-6.,12.,26.));
#11573=CARTESIAN_POINT('',(-12.8284271247462,12.,28.));
#11574=CARTESIAN_POINT('',(-6.,12.,28.));
#11575=CARTESIAN_POINT('',(-12.,10.,26.));
#11576=CARTESIAN_POINT('Origin',(-12.8284271247462,12.,26.));
#11577=CARTESIAN_POINT('',(-6.,10.,26.));
#11578=CARTESIAN_POINT('Origin',(-14.9142135623731,9.9142135623731,26.));
#11579=CARTESIAN_POINT('',(-18.,6.82842712474619,28.));
#11580=CARTESIAN_POINT('',(-14.9142135623731,9.9142135623731,28.));
#11581=CARTESIAN_POINT('',(-16.,6.,26.));
#11582=CARTESIAN_POINT('Origin',(-18.,6.82842712474619,26.));
#11583=CARTESIAN_POINT('',(-13.5,8.5,26.));
#11584=CARTESIAN_POINT('Origin',(-18.,-5.,26.));
#11585=CARTESIAN_POINT('',(-18.,-12.,28.));
#11586=CARTESIAN_POINT('',(-18.,-5.,28.));
#11587=CARTESIAN_POINT('',(-16.,-10.,26.));
#11588=CARTESIAN_POINT('Origin',(-18.,-12.,26.));
#11589=CARTESIAN_POINT('',(-16.,-5.,26.));
#11590=CARTESIAN_POINT('Origin',(8.,-12.,26.));
#11591=CARTESIAN_POINT('',(16.,-10.,26.));
#11592=CARTESIAN_POINT('',(8.,-10.,26.));
#11593=CARTESIAN_POINT('',(18.,-12.,28.));
#11594=CARTESIAN_POINT('',(8.,-12.,28.));
#11595=CARTESIAN_POINT('Origin',(18.,-12.,26.));
#11596=CARTESIAN_POINT('Origin',(18.,3.,26.));
#11597=CARTESIAN_POINT('',(16.,3.,26.));
#11598=CARTESIAN_POINT('',(18.,3.,28.));
#11599=CARTESIAN_POINT('Origin',(16.,-10.,0.));
#11600=CARTESIAN_POINT('',(16.,-10.,8.));
#11601=CARTESIAN_POINT('',(16.,-10.,0.));
#11602=CARTESIAN_POINT('',(13.1979999955782,-10.0000000206464,8.));
#11603=CARTESIAN_POINT('',(8.,-10.,8.));
#11604=CARTESIAN_POINT('',(-13.198,-10.,8.));
#11605=CARTESIAN_POINT('',(8.,-10.,8.));
#11606=CARTESIAN_POINT('',(-16.,-10.,8.));
#11607=CARTESIAN_POINT('',(8.,-10.,8.));
#11608=CARTESIAN_POINT('',(-16.,-10.,0.));
#11609=CARTESIAN_POINT('Origin',(16.,6.,0.));
#11610=CARTESIAN_POINT('',(16.,6.,8.));
#11611=CARTESIAN_POINT('',(16.,6.,0.));
#11612=CARTESIAN_POINT('',(16.,3.,8.));
#11613=CARTESIAN_POINT('',(16.,3.,8.));
#11614=CARTESIAN_POINT('Origin',(12.,10.,0.));
#11615=CARTESIAN_POINT('',(12.,10.,8.));
#11616=CARTESIAN_POINT('',(12.,10.,0.));
#11617=CARTESIAN_POINT('',(11.5,10.5,8.));
#11618=CARTESIAN_POINT('Origin',(0.,0.,28.));
#11619=CARTESIAN_POINT('',(32.,-3.77491721763538,28.));
#11620=CARTESIAN_POINT('',(32.,-18.,28.));
#11621=CARTESIAN_POINT('',(32.,-10.,28.));
#11622=CARTESIAN_POINT('',(32.,3.77491721763538,28.));
#11623=CARTESIAN_POINT('Origin',(28.,0.,28.));
#11624=CARTESIAN_POINT('',(32.,18.,28.));
#11625=CARTESIAN_POINT('',(32.,-10.,28.));
#11626=CARTESIAN_POINT('',(-32.,18.,28.));
#11627=CARTESIAN_POINT('',(17.,18.,28.));
#11628=CARTESIAN_POINT('',(-32.,3.77491721763538,28.));
#11629=CARTESIAN_POINT('',(-32.,10.,28.));
#11630=CARTESIAN_POINT('',(-22.5,-6.73555739531045E-16,28.));
#11631=CARTESIAN_POINT('Origin',(-28.,0.,28.));
#11632=CARTESIAN_POINT('',(-32.,-3.77491721763538,28.));
#11633=CARTESIAN_POINT('Origin',(-28.,0.,28.));
#11634=CARTESIAN_POINT('',(-32.,-18.,28.));
#11635=CARTESIAN_POINT('',(-32.,10.,28.));
#11636=CARTESIAN_POINT('',(-17.,-18.,28.));
#11637=CARTESIAN_POINT('Origin',(32.,-10.,26.));
#11638=CARTESIAN_POINT('',(32.75,-6.37798309992857E-16,27.8540496217739));
#11639=CARTESIAN_POINT('Ctrl Pts',(32.,3.77491721763538,28.));
#11640=CARTESIAN_POINT('Ctrl Pts',(32.0019525144519,3.77000349735399,28.));
#11641=CARTESIAN_POINT('Ctrl Pts',(32.0039017377963,3.76508846538185,27.9999971407691));
#11642=CARTESIAN_POINT('Ctrl Pts',(32.2437689219487,3.15906880248546,27.9992958069976));
#11643=CARTESIAN_POINT('Ctrl Pts',(32.4320766813924,2.53932916982673,27.9572986150603));
#11644=CARTESIAN_POINT('Ctrl Pts',(32.6335924011263,1.53220364744403,27.8985426691076));
#11645=CARTESIAN_POINT('Ctrl Pts',(32.6866197302491,1.16003166445502,27.8787386406688));
#11646=CARTESIAN_POINT('Ctrl Pts',(32.7391880669654,0.522990467484402,27.8585298486776));
#11647=CARTESIAN_POINT('Ctrl Pts',(32.75,0.262060967255928,27.8540496217739));
#11648=CARTESIAN_POINT('Ctrl Pts',(32.75,-6.93889390390723E-16,27.8540496217739));
#11649=CARTESIAN_POINT('Ctrl Pts',(32.75,-6.93889390390723E-16,27.8540496217739));
#11650=CARTESIAN_POINT('Ctrl Pts',(32.75,-0.262060967255973,27.8540496217739));
#11651=CARTESIAN_POINT('Ctrl Pts',(32.7391880669654,-0.522990467484491,
27.8585298486776));
#11652=CARTESIAN_POINT('Ctrl Pts',(32.6866197302491,-1.16003166445499,27.8787386406688));
#11653=CARTESIAN_POINT('Ctrl Pts',(32.6335924011263,-1.53220364744395,27.8985426691076));
#11654=CARTESIAN_POINT('Ctrl Pts',(32.4320766813953,-2.53932916981226,27.9572986150594));
#11655=CARTESIAN_POINT('Ctrl Pts',(32.2437689219548,-3.15906880247018,27.9992958069976));
#11656=CARTESIAN_POINT('Ctrl Pts',(32.0039017377962,-3.76508846538219,27.9999971407691));
#11657=CARTESIAN_POINT('Ctrl Pts',(32.001952514452,-3.77000349735365,28.));
#11658=CARTESIAN_POINT('Ctrl Pts',(32.,-3.77491721763538,28.));
#11659=CARTESIAN_POINT('',(34.,-20.,26.));
#11660=CARTESIAN_POINT('Origin',(32.,-18.,26.));
#11661=CARTESIAN_POINT('',(34.,20.,26.));
#11662=CARTESIAN_POINT('',(34.,-10.,26.));
#11663=CARTESIAN_POINT('Origin',(32.,18.,26.));
#11664=CARTESIAN_POINT('Origin',(-17.,-18.,26.));
#11665=CARTESIAN_POINT('',(-34.,-20.,26.));
#11666=CARTESIAN_POINT('Origin',(-32.,-18.,26.));
#11667=CARTESIAN_POINT('',(-17.,-20.,26.));
#11668=CARTESIAN_POINT('Origin',(-32.,10.,26.));
#11669=CARTESIAN_POINT('Ctrl Pts',(-32.,-3.77491721763538,28.));
#11670=CARTESIAN_POINT('Ctrl Pts',(-32.0019525144519,-3.77000349735395,
28.));
#11671=CARTESIAN_POINT('Ctrl Pts',(-32.0039017377963,-3.7650884653819,27.9999971407691));
#11672=CARTESIAN_POINT('Ctrl Pts',(-32.2437689219487,-3.15906880248546,
27.9992958069976));
#11673=CARTESIAN_POINT('Ctrl Pts',(-32.4320766813924,-2.53932916982673,
27.9572986150603));
#11674=CARTESIAN_POINT('Ctrl Pts',(-32.6335924011263,-1.53220364744392,
27.8985426691076));
#11675=CARTESIAN_POINT('Ctrl Pts',(-32.6866197302491,-1.16003166445497,
27.8787386406688));
#11676=CARTESIAN_POINT('Ctrl Pts',(-32.7391880669654,-0.522990467484492,
27.8585298486776));
#11677=CARTESIAN_POINT('Ctrl Pts',(-32.75,-0.262060967255973,27.8540496217739));
#11678=CARTESIAN_POINT('Ctrl Pts',(-32.75,0.262060967255972,27.8540496217739));
#11679=CARTESIAN_POINT('Ctrl Pts',(-32.7391880669654,0.52299046748449,27.8585298486776));
#11680=CARTESIAN_POINT('Ctrl Pts',(-32.6866197302491,1.16003166445499,27.8787386406688));
#11681=CARTESIAN_POINT('Ctrl Pts',(-32.6335924011263,1.53220364744395,27.8985426691076));
#11682=CARTESIAN_POINT('Ctrl Pts',(-32.4320766813924,2.53932916982672,27.9572986150603));
#11683=CARTESIAN_POINT('Ctrl Pts',(-32.2437689219487,3.15906880248545,27.9992958069976));
#11684=CARTESIAN_POINT('Ctrl Pts',(-32.0039017377963,3.7650884653819,27.9999971407691));
#11685=CARTESIAN_POINT('Ctrl Pts',(-32.0019525144519,3.77000349735395,28.));
#11686=CARTESIAN_POINT('Ctrl Pts',(-32.,3.77491721763538,28.));
#11687=CARTESIAN_POINT('',(-34.,20.,26.));
#11688=CARTESIAN_POINT('Origin',(-32.,18.,26.));
#11689=CARTESIAN_POINT('',(-34.,10.,26.));
#11690=CARTESIAN_POINT('Origin',(17.,18.,26.));
#11691=CARTESIAN_POINT('',(17.,20.,26.));
#11692=CARTESIAN_POINT('Origin',(34.,20.,24.));
#11693=CARTESIAN_POINT('',(34.,20.,24.));
#11694=CARTESIAN_POINT('',(34.,20.,24.));
#11695=CARTESIAN_POINT('',(-34.,20.,24.));
#11696=CARTESIAN_POINT('',(34.,20.,24.));
#11697=CARTESIAN_POINT('',(-34.,20.,24.));
#11698=CARTESIAN_POINT('Origin',(34.,-20.,24.));
#11699=CARTESIAN_POINT('',(34.,-20.,24.));
#11700=CARTESIAN_POINT('',(34.,-20.,24.));
#11701=CARTESIAN_POINT('',(34.,-20.,24.));
#11702=CARTESIAN_POINT('Origin',(28.,0.,26.));
#11703=CARTESIAN_POINT('',(31.5,-6.16297582203915E-32,26.));
#11704=CARTESIAN_POINT('Origin',(33.5,-6.73555739531044E-16,26.));
#11705=CARTESIAN_POINT('',(24.5,4.28626379701574E-16,26.));
#11706=CARTESIAN_POINT('Origin',(28.,0.,26.));
#11707=CARTESIAN_POINT('Origin',(28.,0.,26.));
#11708=CARTESIAN_POINT('Origin',(-28.,0.,26.));
#11709=CARTESIAN_POINT('',(-24.5,-6.16297582203915E-32,26.));
#11710=CARTESIAN_POINT('Origin',(-22.5,-6.73555739531044E-16,26.));
#11711=CARTESIAN_POINT('',(-31.5,4.28626379701574E-16,26.));
#11712=CARTESIAN_POINT('Origin',(-28.,0.,26.));
#11713=CARTESIAN_POINT('Origin',(-28.,0.,26.));
#11714=CARTESIAN_POINT('Origin',(28.,0.,26.));
#11715=CARTESIAN_POINT('',(24.5,4.28626379701574E-16,24.));
#11716=CARTESIAN_POINT('',(24.5,4.28626379701574E-16,26.));
#11717=CARTESIAN_POINT('Origin',(28.,0.,24.));
#11718=CARTESIAN_POINT('Origin',(-28.,0.,26.));
#11719=CARTESIAN_POINT('',(-31.5,4.28626379701574E-16,24.));
#11720=CARTESIAN_POINT('',(-31.5,4.28626379701574E-16,26.));
#11721=CARTESIAN_POINT('Origin',(-28.,0.,24.));
#11722=CARTESIAN_POINT('Origin',(-15.,-10.,9.54592528053767));
#11723=CARTESIAN_POINT('Ctrl Pts',(-17.0565470023424,-9.99851185632501,
7.79592528053768));
#11724=CARTESIAN_POINT('Ctrl Pts',(-17.0573685745232,-9.90014528989089,
7.79057696270225));
#11725=CARTESIAN_POINT('Ctrl Pts',(-17.0062396084505,-9.12123442332477,
7.74818159569048));
#11726=CARTESIAN_POINT('Ctrl Pts',(-16.0106088364074,-7.79139167661744,
7.66873917950237));
#11727=CARTESIAN_POINT('Ctrl Pts',(-13.6926511338527,-7.95337102943111,
7.55759803197335));
#11728=CARTESIAN_POINT('Ctrl Pts',(-12.5713805503198,-9.98835294159719,
7.44645688444433));
#11729=CARTESIAN_POINT('Ctrl Pts',(-13.6731764957754,-12.0342028340593,
7.3353157369153));
#11730=CARTESIAN_POINT('Ctrl Pts',(-15.989492000612,-12.2179172171411,7.22417458938629));
#11731=CARTESIAN_POINT('Ctrl Pts',(-17.0022526535647,-10.8922265068485,
7.14437777059375));
#11732=CARTESIAN_POINT('Ctrl Pts',(-17.0572655365823,-10.1065381991343,
7.10162800097754));
#11733=CARTESIAN_POINT('Ctrl Pts',(-17.0563656598722,-10.0016028745823,
7.09592528053768));
#11734=CARTESIAN_POINT('Ctrl Pts',(-17.0526884867324,-10.0024695060038,
7.85407471946233));
#11735=CARTESIAN_POINT('Ctrl Pts',(-17.0491243427736,-9.53216561815421,
7.82862238128887));
#11736=CARTESIAN_POINT('Ctrl Pts',(-16.6564412157395,-8.37020235436293,
7.76612299393908));
#11737=CARTESIAN_POINT('Ctrl Pts',(-14.727662200004,-7.58731060863186,7.66657655741293));
#11738=CARTESIAN_POINT('Ctrl Pts',(-12.8251332301876,-8.91924943693317,
7.55543540988393));
#11739=CARTESIAN_POINT('Ctrl Pts',(-12.9125601407559,-11.2417229038903,
7.4442942623549));
#11740=CARTESIAN_POINT('Ctrl Pts',(-14.9111754350777,-12.4269243298781,
7.33315311482589));
#11741=CARTESIAN_POINT('Ctrl Pts',(-16.721395498903,-11.5251875586803,7.23641326719502));
#11742=CARTESIAN_POINT('Ctrl Pts',(-17.0498948337479,-10.417780764987,7.1767204687405));
#11743=CARTESIAN_POINT('Ctrl Pts',(-17.0520596215353,-9.99884120146076,
7.15407471946233));
#11744=CARTESIAN_POINT('Ctrl Pts',(-13.7309291201476,-8.92064134695149,
8.));
#11745=CARTESIAN_POINT('Ctrl Pts',(-13.3720061708544,-9.34264997380806,
7.96295295082366));
#11746=CARTESIAN_POINT('Ctrl Pts',(-13.1145386540675,-10.5656659613133,
7.88885885247098));
#11747=CARTESIAN_POINT('Ctrl Pts',(-14.4551162761764,-11.893574716725,7.77771770494197));
#11748=CARTESIAN_POINT('Ctrl Pts',(-16.2942887603119,-11.4833631126878,
7.66657655741294));
#11749=CARTESIAN_POINT('Ctrl Pts',(-16.9487772336236,-9.71772814539447,
7.55543540988392));
#11750=CARTESIAN_POINT('Ctrl Pts',(-15.8194059235697,-8.20925101995117,
7.4442942623549));
#11751=CARTESIAN_POINT('Ctrl Pts',(-13.9399960038928,-8.34058456504792,
7.33315311482588));
#11752=CARTESIAN_POINT('Ctrl Pts',(-13.0308650672018,-9.9905565157323,7.22201196729686));
#11753=CARTESIAN_POINT('Ctrl Pts',(-13.9242058848823,-11.6493402708567,
7.11087081976784));
#11754=CARTESIAN_POINT('Ctrl Pts',(-15.8022843036961,-11.798296670523,6.99972967223882));
#11755=CARTESIAN_POINT('Ctrl Pts',(-16.9459843182726,-10.3012080146147,
6.88858852470981));
#11756=CARTESIAN_POINT('Ctrl Pts',(-16.3084067449585,-8.52838242895221,
6.77744737718078));
#11757=CARTESIAN_POINT('Ctrl Pts',(-14.4731656133806,-8.10262926439867,
6.66630622965177));
#11758=CARTESIAN_POINT('Ctrl Pts',(-13.1201677229713,-9.41364812851512,
6.55516508212274));
#11759=CARTESIAN_POINT('Ctrl Pts',(-13.4878940440534,-11.2613934759824,
6.44402393459372));
#11760=CARTESIAN_POINT('Ctrl Pts',(-15.2397423409267,-11.9545074742511,
6.33288278706471));
#11761=CARTESIAN_POINT('Ctrl Pts',(-16.7721399948386,-10.8585434454103,
6.22174163953568));
#11762=CARTESIAN_POINT('Ctrl Pts',(-16.6823907514308,-8.97670225553072,
6.11060049200667));
#11763=CARTESIAN_POINT('Ctrl Pts',(-15.0526475335092,-8.03154758812267,
5.99945934447764));
#11764=CARTESIAN_POINT('Ctrl Pts',(-13.3747128424705,-8.888236318563,5.88831819694863));
#11765=CARTESIAN_POINT('Ctrl Pts',(-13.1845017596292,-10.7625896281669,
5.7771770494196));
#11766=CARTESIAN_POINT('Ctrl Pts',(-14.6561259881869,-11.938898510967,5.66603590189058));
#11767=CARTESIAN_POINT('Ctrl Pts',(-16.4425188921508,-11.3404163686345,
5.55489475436156));
#11768=CARTESIAN_POINT('Ctrl Pts',(-16.908487033224,-9.51497006870877,5.44375360683254));
#11769=CARTESIAN_POINT('Ctrl Pts',(-15.6275015977553,-8.13350099606285,
5.33261245930353));
#11770=CARTESIAN_POINT('Ctrl Pts',(-13.7721260084407,-8.46055131588728,
5.22147131177451));
#11771=CARTESIAN_POINT('Ctrl Pts',(-13.0406977260285,-10.1967520989212,
5.11033016424549));
#11772=CARTESIAN_POINT('Ctrl Pts',(-14.1027372825927,-11.7528537887758,
4.99918901671646));
#11773=CARTESIAN_POINT('Ctrl Pts',(-15.9860956566683,-11.7044624211814,
4.88804786918745));
#11774=CARTESIAN_POINT('Ctrl Pts',(-16.9668210527183,-10.0958735403876,
4.77690672165842));
#11775=CARTESIAN_POINT('Ctrl Pts',(-16.1471962169778,-8.39952581124097,
4.6657655741294));
#11776=CARTESIAN_POINT('Ctrl Pts',(-14.2774733195481,-8.16818887839767,
4.55462442660039));
#11777=CARTESIAN_POINT('Ctrl Pts',(-13.069122779726,-9.61361942415149,4.44348327907136));
#11778=CARTESIAN_POINT('Ctrl Pts',(-13.628220908545,-11.4127274731565,4.33234213154235));
#11779=CARTESIAN_POINT('Ctrl Pts',(-15.4429913832827,-11.9186806465666,
4.22120098401332));
#11780=CARTESIAN_POINT('Ctrl Pts',(-16.8522650597871,-10.6683494127027,
4.11005983648431));
#11781=CARTESIAN_POINT('Ctrl Pts',(-16.5660485313643,-8.80623755018859,
3.99891868895528));
#11782=CARTESIAN_POINT('Ctrl Pts',(-14.8463330923299,-8.03684863786395,
3.88777754142627));
#11783=CARTESIAN_POINT('Ctrl Pts',(-13.2672782652309,-9.06445086765756,
3.77663639389725));
#11784=CARTESIAN_POINT('Ctrl Pts',(-13.2742884095798,-10.9484177855025,
3.66549524636822));
#11785=CARTESIAN_POINT('Ctrl Pts',(-14.8609467163918,-11.9642405589667,
3.55435409883921));
#11786=CARTESIAN_POINT('Ctrl Pts',(-16.5748889014339,-11.182075182594,3.44321295131019));
#11787=CARTESIAN_POINT('Ctrl Pts',(-16.8472400506147,-9.31788491838175,
3.33207180378117));
#11788=CARTESIAN_POINT('Ctrl Pts',(-15.4287006895954,-8.07807583189886,
3.22093065625215));
#11789=CARTESIAN_POINT('Ctrl Pts',(-13.6177456663529,-8.59752014408551,
3.10978950872313));
#11790=CARTESIAN_POINT('Ctrl Pts',(-13.0720516115789,-10.4007390681565,
2.99864836119411));
#11791=CARTESIAN_POINT('Ctrl Pts',(-14.2911252885726,-11.8371372928603,
2.88750721366509));
#11792=CARTESIAN_POINT('Ctrl Pts',(-16.1590748504492,-11.5918926722399,
2.77636606613607));
#11793=CARTESIAN_POINT('Ctrl Pts',(-16.9660531192297,-9.88949243651641,
2.66522491860705));
#11794=CARTESIAN_POINT('Ctrl Pts',(-15.9733840920941,-8.28824645482409,
2.55408377107803));
#11795=CARTESIAN_POINT('Ctrl Pts',(-14.0897177507374,-8.25387199393599,
2.44294262354901));
#11796=CARTESIAN_POINT('Ctrl Pts',(-13.0392877913138,-9.8178340730497,2.33180147601999));
#11797=CARTESIAN_POINT('Ctrl Pts',(-13.7836162699446,-11.5485436438058,
2.22066032849097));
#11798=CARTESIAN_POINT('Ctrl Pts',(-15.6413743232439,-11.8617775778309,
2.10951918096195));
#11799=CARTESIAN_POINT('Ctrl Pts',(-16.9120436804446,-10.4708139397355,
1.99837803343293));
#11800=CARTESIAN_POINT('Ctrl Pts',(-16.4325038426079,-8.64888580471299,
1.88723688590391));
#11801=CARTESIAN_POINT('Ctrl Pts',(-14.6417066305057,-8.06371424578222,
1.77609573837489));
#11802=CARTESIAN_POINT('Ctrl Pts',(-13.1788769878056,-9.25094199904707,
1.66495459084587));
#11803=CARTESIAN_POINT('Ctrl Pts',(-13.3830313811546,-11.1238280538555,
1.55381344331685));
#11804=CARTESIAN_POINT('Ctrl Pts',(-15.0672948613758,-11.9680059091803,
1.44267229578783));
#11805=CARTESIAN_POINT('Ctrl Pts',(-16.6899593997283,-11.0107497962058,
1.33153114825881));
#11806=CARTESIAN_POINT('Ctrl Pts',(-16.7657016971608,-9.12829166368782,
1.22039000072979));
#11807=CARTESIAN_POINT('Ctrl Pts',(-15.2251908964839,-8.04376401234878,
1.10924885320077));
#11808=CARTESIAN_POINT('Ctrl Pts',(-13.4785484246367,-8.74989136892269,
0.998107705671749));
#11809=CARTESIAN_POINT('Ctrl Pts',(-13.1245841771335,-10.6003305142777,
0.88696655814273));
#11810=CARTESIAN_POINT('Ctrl Pts',(-14.4872983188498,-11.9012280255974,
0.775825410613709));
#11811=CARTESIAN_POINT('Ctrl Pts',(-16.3193253350176,-11.4618607893957,
0.66468426308469));
#11812=CARTESIAN_POINT('Ctrl Pts',(-16.9436824216117,-9.68427827620017,
0.55354311555567));
#11813=CARTESIAN_POINT('Ctrl Pts',(-15.788892098895,-8.19586106027792,0.44240196802665));
#11814=CARTESIAN_POINT('Ctrl Pts',(-13.9119372726392,-8.3585593283779,0.331260820497631));
#11815=CARTESIAN_POINT('Ctrl Pts',(-13.031037036911,-10.0243917235043,0.22011967296861));
#11816=CARTESIAN_POINT('Ctrl Pts',(-13.9522832423509,-11.6666850676998,
0.10897852543959));
#11817=CARTESIAN_POINT('Ctrl Pts',(-15.8328835456553,-11.7857291171073,
-0.00216262208942913));
#11818=CARTESIAN_POINT('Ctrl Pts',(-16.9505137600752,-10.2654025971077,
-0.113303769618449));
#11819=CARTESIAN_POINT('Ctrl Pts',(-16.5058833578897,-9.0973437658213,-0.187397867971129));
#11820=CARTESIAN_POINT('Ctrl Pts',(-16.0856682637066,-8.73632265938642,
-0.224444917147469));
#11821=CARTESIAN_POINT('Ctrl Pts',(-13.6322193753412,-8.83668763019027,
8.07481497238249));
#11822=CARTESIAN_POINT('Ctrl Pts',(-13.2453789997699,-9.29152055750512,
8.03776792320615));
#11823=CARTESIAN_POINT('Ctrl Pts',(-12.9678853731089,-10.6096640890565,
7.96367382485346));
#11824=CARTESIAN_POINT('Ctrl Pts',(-14.4127346139843,-12.0408590646896,
7.85253267732446));
#11825=CARTESIAN_POINT('Ctrl Pts',(-16.394959979914,-11.5987407457524,7.74139152979542));
#11826=CARTESIAN_POINT('Ctrl Pts',(-17.1003552947622,-9.69577272653137,
7.63025038226641));
#11827=CARTESIAN_POINT('Ctrl Pts',(-15.8831402278489,-8.06996457217325,
7.51910923473739));
#11828=CARTESIAN_POINT('Ctrl Pts',(-13.8575477138794,-8.21151338650899,
7.40796808720837));
#11829=CARTESIAN_POINT('Ctrl Pts',(-12.8777035615744,-9.98982199102059,
7.29682693967935));
#11830=CARTESIAN_POINT('Ctrl Pts',(-13.8405294218466,-11.7776277919242,
7.18568579215033));
#11831=CARTESIAN_POINT('Ctrl Pts',(-15.8646868693347,-11.9381701860624,
7.0745446446213));
#11832=CARTESIAN_POINT('Ctrl Pts',(-17.0973451433484,-10.3246363090688,
6.96340349709229));
#11833=CARTESIAN_POINT('Ctrl Pts',(-16.4101760771119,-8.41391837718253,
6.85226234956327));
#11834=CARTESIAN_POINT('Ctrl Pts',(-14.4321878487151,-7.95504965786306,
6.74112120203425));
#11835=CARTESIAN_POINT('Ctrl Pts',(-12.973952277254,-9.36804102766683,6.62998005450523));
#11836=CARTESIAN_POINT('Ctrl Pts',(-13.3702807606652,-11.3595060637751,
6.51883890697621));
#11837=CARTESIAN_POINT('Ctrl Pts',(-15.2583897669041,-12.1065312398804,
6.40769775944719));
#11838=CARTESIAN_POINT('Ctrl Pts',(-16.9099790150454,-10.9253219096766,
6.29655661191817));
#11839=CARTESIAN_POINT('Ctrl Pts',(-16.8132489756442,-8.89710901860346,
6.18541546438915));
#11840=CARTESIAN_POINT('Ctrl Pts',(-15.0567425172331,-7.87843916973185,
6.07427431686013));
#11841=CARTESIAN_POINT('Ctrl Pts',(-13.2482961993154,-8.80176210264491,
5.96313316933111));
#11842=CARTESIAN_POINT('Ctrl Pts',(-13.0432902868512,-10.8219046977847,
5.8519920218021));
#11843=CARTESIAN_POINT('Ctrl Pts',(-14.6293790850072,-12.0897081940679,
5.74085087427307));
#11844=CARTESIAN_POINT('Ctrl Pts',(-16.5547196163051,-11.4446754449263,
5.62970972674406));
#11845=CARTESIAN_POINT('Ctrl Pts',(-17.056931277755,-9.47724390108383,5.51856857921503));
#11846=CARTESIAN_POINT('Ctrl Pts',(-15.6763093700897,-7.98832262715918,
5.40742743168601));
#11847=CARTESIAN_POINT('Ctrl Pts',(-13.676620603435,-8.34081128468504,5.296286284157));
#11848=CARTESIAN_POINT('Ctrl Pts',(-12.888301015543,-10.2120556960512,5.18514513662797));
#11849=CARTESIAN_POINT('Ctrl Pts',(-14.0329471902773,-11.8891927064202,
5.07400398909895));
#11850=CARTESIAN_POINT('Ctrl Pts',(-16.0627952738211,-11.8370374044215,
4.96286284156994));
#11851=CARTESIAN_POINT('Ctrl Pts',(-17.119802582179,-10.1033306910129,4.85172169404091));
#11852=CARTESIAN_POINT('Ctrl Pts',(-16.236426414927,-8.27503914839981,4.7405805465119));
#11853=CARTESIAN_POINT('Ctrl Pts',(-14.2212743905714,-8.02570857157036,
4.62943939898287));
#11854=CARTESIAN_POINT('Ctrl Pts',(-12.9189370015384,-9.58356631313487,
4.51829825145385));
#11855=CARTESIAN_POINT('Ctrl Pts',(-13.5215224047829,-11.5226109876002,
4.40715710392484));
#11856=CARTESIAN_POINT('Ctrl Pts',(-15.477447745878,-12.0679177616832,4.29601595639581));
#11857=CARTESIAN_POINT('Ctrl Pts',(-16.9963362966803,-10.7203343735246,
4.18487480886679));
#11858=CARTESIAN_POINT('Ctrl Pts',(-16.6878575282767,-8.71338537884723,
4.07373366133777));
#11859=CARTESIAN_POINT('Ctrl Pts',(-14.8343807093053,-7.88415254101912,
3.96259251380876));
#11860=CARTESIAN_POINT('Ctrl Pts',(-13.1325052411429,-8.99168281539703,
3.85145136627973));
#11861=CARTESIAN_POINT('Ctrl Pts',(-13.1400606423177,-11.0221867759215,
3.74031021875072));
#11862=CARTESIAN_POINT('Ctrl Pts',(-14.8501309973036,-12.1170213747526,
3.62916907122169));
#11863=CARTESIAN_POINT('Ctrl Pts',(-16.6973855121647,-11.2740183052897,
3.51802792369268));
#11864=CARTESIAN_POINT('Ctrl Pts',(-16.9909204367044,-9.26482924851799,
3.40688677616366));
#11865=CARTESIAN_POINT('Ctrl Pts',(-15.4620455061381,-7.92858643206906,
3.29574562863463));
#11866=CARTESIAN_POINT('Ctrl Pts',(-13.5102323866,-8.48843370071082,3.18460448110562));
#11867=CARTESIAN_POINT('Ctrl Pts',(-12.922093641191,-10.4319089986779,3.07346333357659));
#11868=CARTESIAN_POINT('Ctrl Pts',(-14.2359882249336,-11.9800318752131,
2.96232218604758));
#11869=CARTESIAN_POINT('Ctrl Pts',(-16.2492289817241,-11.7157118551798,
2.85118103851855));
#11870=CARTESIAN_POINT('Ctrl Pts',(-17.1189749179693,-9.88089703529509,
2.74003989098954));
#11871=CARTESIAN_POINT('Ctrl Pts',(-16.0490949896134,-8.15510435984867,
2.62889874346051));
#11872=CARTESIAN_POINT('Ctrl Pts',(-14.0189149847508,-8.11805621515299,
2.5177575959315));
#11873=CARTESIAN_POINT('Ctrl Pts',(-12.8867814145378,-9.80366500460193,
2.40661644840247));
#11874=CARTESIAN_POINT('Ctrl Pts',(-13.6890045902609,-11.6689910910907,
2.29547530087346));
#11875=CARTESIAN_POINT('Ctrl Pts',(-15.6912611315994,-12.0065887089597,
2.18433415334443));
#11876=CARTESIAN_POINT('Ctrl Pts',(-17.060764564953,-10.5074343717227,2.07319300581542));
#11877=CARTESIAN_POINT('Ctrl Pts',(-16.5439255850677,-8.54379463956336,
1.9620518582864));
#11878=CARTESIAN_POINT('Ctrl Pts',(-14.6138381736448,-7.91310778580779,
1.85091071075738));
#11879=CARTESIAN_POINT('Ctrl Pts',(-13.0372280140179,-9.19267943444714,
1.73976956322836));
#11880=CARTESIAN_POINT('Ctrl Pts',(-13.2572617631922,-11.2112406500812,
1.62862841569934));
#11881=CARTESIAN_POINT('Ctrl Pts',(-15.0725291305554,-12.1210795980947,
1.51748726817032));
#11882=CARTESIAN_POINT('Ctrl Pts',(-16.821406321826,-11.0893670397582,1.4063461206413));
#11883=CARTESIAN_POINT('Ctrl Pts',(-16.903039939412,-9.06048921956191,1.29520497311228));
#11884=CARTESIAN_POINT('Ctrl Pts',(-15.2427064949249,-7.89160580102436,
1.18406382558326));
#11885=CARTESIAN_POINT('Ctrl Pts',(-13.3602082285737,-8.65265652892044,
1.07292267805424));
#11886=CARTESIAN_POINT('Ctrl Pts',(-12.978712248134,-10.6470248895129,0.961781530525217));
#11887=CARTESIAN_POINT('Ctrl Pts',(-14.4474198117375,-12.04910765644,0.850640382996199));
#11888=CARTESIAN_POINT('Ctrl Pts',(-16.4219439272521,-11.5755659478345,
0.739499235467178));
#11889=CARTESIAN_POINT('Ctrl Pts',(-17.0948642026044,-9.65972108929999,
0.62835808793816));
#11890=CARTESIAN_POINT('Ctrl Pts',(-15.8502530039462,-8.05553312654103,
0.517216940409138));
#11891=CARTESIAN_POINT('Ctrl Pts',(-13.8273065432951,-8.2308862469267,0.40607579288012));
#11892=CARTESIAN_POINT('Ctrl Pts',(-12.8778889072789,-10.0262889388929,
0.294934645351099));
#11893=CARTESIAN_POINT('Ctrl Pts',(-13.8707906674137,-11.796321686361,0.183793497822079));
#11894=CARTESIAN_POINT('Ctrl Pts',(-15.8976661543735,-11.9246251143613,
0.07265235029306));
#11895=CARTESIAN_POINT('Ctrl Pts',(-17.102226890173,-10.2860459063565,-0.0384887972359602));
#11896=CARTESIAN_POINT('Ctrl Pts',(-16.6230126406787,-9.02713415977149,
-0.11258289558864));
#11897=CARTESIAN_POINT('Ctrl Pts',(-16.170112749004,-8.63803243006198,-0.14962994476498));
#11898=CARTESIAN_POINT('Ctrl Pts',(-13.5335096305347,-8.75273391342904,
8.14962994476498));
#11899=CARTESIAN_POINT('Ctrl Pts',(-13.1187518286854,-9.24039114120217,
8.11258289558864));
#11900=CARTESIAN_POINT('Ctrl Pts',(-12.8212320921502,-10.6536622167997,
8.03848879723595));
#11901=CARTESIAN_POINT('Ctrl Pts',(-14.3703529517921,-12.1881434126541,
7.92734764970695));
#11902=CARTESIAN_POINT('Ctrl Pts',(-16.4956311995161,-11.7141183788172,
7.81620650217792));
#11903=CARTESIAN_POINT('Ctrl Pts',(-17.2519333559009,-9.67381730766822,
7.7050653546489));
#11904=CARTESIAN_POINT('Ctrl Pts',(-15.9468745321282,-7.93067812439536,
7.59392420711988));
#11905=CARTESIAN_POINT('Ctrl Pts',(-13.7750994238661,-8.08244220797005,
7.48278305959086));
#11906=CARTESIAN_POINT('Ctrl Pts',(-12.7245420559471,-9.9890874663089,7.37164191206184));
#11907=CARTESIAN_POINT('Ctrl Pts',(-13.756852958811,-11.9059153129918,7.26050076453282));
#11908=CARTESIAN_POINT('Ctrl Pts',(-15.9270894349734,-12.0780437016018,
7.1493596170038));
#11909=CARTESIAN_POINT('Ctrl Pts',(-17.2487059684241,-10.3480646035229,
7.03821846947478));
#11910=CARTESIAN_POINT('Ctrl Pts',(-16.5119454092653,-8.29945432541285,
6.92707732194576));
#11911=CARTESIAN_POINT('Ctrl Pts',(-14.3912100840495,-7.80747005132744,
6.81593617441674));
#11912=CARTESIAN_POINT('Ctrl Pts',(-12.8277368315367,-9.32243392681855,
6.70479502688772));
#11913=CARTESIAN_POINT('Ctrl Pts',(-13.252667477277,-11.4576186515678,6.59365387935869));
#11914=CARTESIAN_POINT('Ctrl Pts',(-15.2770371928816,-12.2585550055097,
6.48251273182969));
#11915=CARTESIAN_POINT('Ctrl Pts',(-17.0478180352521,-10.9921003739429,
6.37137158430066));
#11916=CARTESIAN_POINT('Ctrl Pts',(-16.9441071998576,-8.81751578167622,
6.26023043677165));
#11917=CARTESIAN_POINT('Ctrl Pts',(-15.0608375009569,-7.72533075134102,
6.14908928924262));
#11918=CARTESIAN_POINT('Ctrl Pts',(-13.1218795561602,-8.71528788672682,
6.03794814171361));
#11919=CARTESIAN_POINT('Ctrl Pts',(-12.9020788140733,-10.8812197674026,
5.92680699418457));
#11920=CARTESIAN_POINT('Ctrl Pts',(-14.6026321818275,-12.2405178771688,
5.81566584665556));
#11921=CARTESIAN_POINT('Ctrl Pts',(-16.6669203404595,-11.5489345212182,
5.70452469912655));
#11922=CARTESIAN_POINT('Ctrl Pts',(-17.205375522286,-9.43951773345887,5.59338355159752));
#11923=CARTESIAN_POINT('Ctrl Pts',(-15.7251171424241,-7.84314425825552,
5.4822424040685));
#11924=CARTESIAN_POINT('Ctrl Pts',(-13.5811151984292,-8.22107125348279,
5.37110125653949));
#11925=CARTESIAN_POINT('Ctrl Pts',(-12.7359043050575,-10.2273592931811,
5.25996010901046));
#11926=CARTESIAN_POINT('Ctrl Pts',(-13.9631570979619,-12.0255316240646,
5.14881896148144));
#11927=CARTESIAN_POINT('Ctrl Pts',(-16.1394948909739,-11.9696123876616,
5.03767781395243));
#11928=CARTESIAN_POINT('Ctrl Pts',(-17.2727841116396,-10.1107878416383,
4.92653666642339));
#11929=CARTESIAN_POINT('Ctrl Pts',(-16.3256566128762,-8.15055248555867,
4.81539551889439));
#11930=CARTESIAN_POINT('Ctrl Pts',(-14.1650754615946,-7.88322826474304,
4.70425437136536));
#11931=CARTESIAN_POINT('Ctrl Pts',(-12.7687512233509,-9.55351320211825,
4.59311322383635));
#11932=CARTESIAN_POINT('Ctrl Pts',(-13.4148239010208,-11.6324945020439,
4.48197207630732));
#11933=CARTESIAN_POINT('Ctrl Pts',(-15.5119041084733,-12.2171548767998,
4.37083092877831));
#11934=CARTESIAN_POINT('Ctrl Pts',(-17.1404075335735,-10.7723193343466,
4.25968978124929));
#11935=CARTESIAN_POINT('Ctrl Pts',(-16.809666525189,-8.62053320750586,4.14854863372026));
#11936=CARTESIAN_POINT('Ctrl Pts',(-14.8224283262808,-7.73145644417431,
4.03740748619125));
#11937=CARTESIAN_POINT('Ctrl Pts',(-12.997732217055,-8.9189147631365,3.92626633866222));
#11938=CARTESIAN_POINT('Ctrl Pts',(-13.0058328750556,-11.0959557663405,
3.81512519113321));
#11939=CARTESIAN_POINT('Ctrl Pts',(-14.8393152782154,-12.2698021905386,
3.70398404360418));
#11940=CARTESIAN_POINT('Ctrl Pts',(-16.8198821228955,-11.3659614279855,
3.59284289607517));
#11941=CARTESIAN_POINT('Ctrl Pts',(-17.1346008227942,-9.21177357865423,
3.48170174854615));
#11942=CARTESIAN_POINT('Ctrl Pts',(-15.4953903226807,-7.77909703223927,
3.37056060101712));
#11943=CARTESIAN_POINT('Ctrl Pts',(-13.402719106847,-8.3793472573361,3.25941945348811));
#11944=CARTESIAN_POINT('Ctrl Pts',(-12.7721356708031,-10.4630789291993,
3.14827830595908));
#11945=CARTESIAN_POINT('Ctrl Pts',(-14.1808511612947,-12.1229264575659,
3.03713715843007));
#11946=CARTESIAN_POINT('Ctrl Pts',(-16.339383112999,-11.8395310381196,2.92599601090104));
#11947=CARTESIAN_POINT('Ctrl Pts',(-17.2718967167089,-9.87230163407375,
2.81485486337203));
#11948=CARTESIAN_POINT('Ctrl Pts',(-16.1248058871327,-8.02196226487325,
2.703713715843));
#11949=CARTESIAN_POINT('Ctrl Pts',(-13.9481122187642,-7.98224043637001,
2.59257256831399));
#11950=CARTESIAN_POINT('Ctrl Pts',(-12.7342750377617,-9.78949593615416,
2.48143142078496));
#11951=CARTESIAN_POINT('Ctrl Pts',(-13.5943929105772,-11.7894385383755,
2.37029027325595));
#11952=CARTESIAN_POINT('Ctrl Pts',(-15.741147939955,-12.1513998400885,2.25914912572692));
#11953=CARTESIAN_POINT('Ctrl Pts',(-17.2094854494613,-10.5440548037099,
2.14800797819791));
#11954=CARTESIAN_POINT('Ctrl Pts',(-16.6553473275274,-8.43870347441375,
2.03686683066889));
#11955=CARTESIAN_POINT('Ctrl Pts',(-14.5859697167838,-7.76250132583336,
1.92572568313987));
#11956=CARTESIAN_POINT('Ctrl Pts',(-12.8955790402303,-9.13441686984722,
1.81458453561085));
#11957=CARTESIAN_POINT('Ctrl Pts',(-13.1314921452297,-11.298653246307,1.70344338808183));
#11958=CARTESIAN_POINT('Ctrl Pts',(-15.0777633997351,-12.274153287009,1.59230224055281));
#11959=CARTESIAN_POINT('Ctrl Pts',(-16.9528532439237,-11.1679842833106,
1.48116109302379));
#11960=CARTESIAN_POINT('Ctrl Pts',(-17.0403781816632,-8.99268677543598,
1.37001994549477));
#11961=CARTESIAN_POINT('Ctrl Pts',(-15.2602220933659,-7.73944758969995,
1.25887879796575));
#11962=CARTESIAN_POINT('Ctrl Pts',(-13.2418680325108,-8.55542168891818,
1.14773765043673));
#11963=CARTESIAN_POINT('Ctrl Pts',(-12.8328403191345,-10.6937192647481,
1.03659650290771));
#11964=CARTESIAN_POINT('Ctrl Pts',(-14.4075413046253,-12.1969872872825,
0.925455355378688));
#11965=CARTESIAN_POINT('Ctrl Pts',(-16.5245625194866,-11.6892711062734,
0.814314207849668));
#11966=CARTESIAN_POINT('Ctrl Pts',(-17.2460459835971,-9.63516390239978,
0.703173060320648));
#11967=CARTESIAN_POINT('Ctrl Pts',(-15.9116139089972,-7.91520519280415,
0.592031912791628));
#11968=CARTESIAN_POINT('Ctrl Pts',(-13.7426758139511,-8.10321316547549,
0.480890765262609));
#11969=CARTESIAN_POINT('Ctrl Pts',(-12.7247407776469,-10.0281861542815,
0.369749617733589));
#11970=CARTESIAN_POINT('Ctrl Pts',(-13.7892980924765,-11.9259583050221,
0.258608470204568));
#11971=CARTESIAN_POINT('Ctrl Pts',(-15.9624487630916,-12.0635211116153,
0.147467322675549));
#11972=CARTESIAN_POINT('Ctrl Pts',(-17.2539400202709,-10.3066892156053,
0.0363261751465287));
#11973=CARTESIAN_POINT('Ctrl Pts',(-16.7401419234677,-8.95692455372168,
-0.0377679232061509));
#11974=CARTESIAN_POINT('Ctrl Pts',(-16.2545572343013,-8.53974220073755,
-0.0748149723824913));
#11975=CARTESIAN_POINT('Ctrl Pts',(-13.4347998857283,-8.66878019666781,
8.22444491714747));
#11976=CARTESIAN_POINT('Ctrl Pts',(-12.9921246576009,-9.18926172489923,
8.18739786797113));
#11977=CARTESIAN_POINT('Ctrl Pts',(-12.6745788111916,-10.6976603445429,
8.11330376961844));
#11978=CARTESIAN_POINT('Ctrl Pts',(-14.3279712896,-12.3354277606187,8.00216262208943));
#11979=CARTESIAN_POINT('Ctrl Pts',(-16.5963024191182,-11.8294960118818,
7.89102147456041));
#11980=CARTESIAN_POINT('Ctrl Pts',(-17.4035114170396,-9.65186188880512,
7.77988032703139));
#11981=CARTESIAN_POINT('Ctrl Pts',(-16.0106088364074,-7.79139167661744,
7.66873917950237));
#11982=CARTESIAN_POINT('Ctrl Pts',(-13.6926511338527,-7.95337102943111,
7.55759803197335));
#11983=CARTESIAN_POINT('Ctrl Pts',(-12.5713805503198,-9.98835294159719,
7.44645688444433));
#11984=CARTESIAN_POINT('Ctrl Pts',(-13.6731764957754,-12.0342028340593,
7.3353157369153));
#11985=CARTESIAN_POINT('Ctrl Pts',(-15.989492000612,-12.2179172171411,7.22417458938629));
#11986=CARTESIAN_POINT('Ctrl Pts',(-17.4000667934998,-10.371492897977,7.11303344185727));
#11987=CARTESIAN_POINT('Ctrl Pts',(-16.6137147414187,-8.18499027364317,
7.00189229432825));
#11988=CARTESIAN_POINT('Ctrl Pts',(-14.350232319384,-7.65989044479182,6.89075114679923));
#11989=CARTESIAN_POINT('Ctrl Pts',(-12.6815213858194,-9.27682682597027,
6.77960999927021));
#11990=CARTESIAN_POINT('Ctrl Pts',(-13.1350541938888,-11.5557312393606,
6.66846885174119));
#11991=CARTESIAN_POINT('Ctrl Pts',(-15.295684618859,-12.4105787711389,6.55732770421217));
#11992=CARTESIAN_POINT('Ctrl Pts',(-17.185657055459,-11.0588788382093,6.44618655668315));
#11993=CARTESIAN_POINT('Ctrl Pts',(-17.0749654240711,-8.73792254474896,
6.33504540915413));
#11994=CARTESIAN_POINT('Ctrl Pts',(-15.0649324846807,-7.5722223329502,6.22390426162511));
#11995=CARTESIAN_POINT('Ctrl Pts',(-12.995462913005,-8.62881367080874,6.11276311409609));
#11996=CARTESIAN_POINT('Ctrl Pts',(-12.7608673412954,-10.9405348370204,
6.00162196656707));
#11997=CARTESIAN_POINT('Ctrl Pts',(-14.5758852786477,-12.3913275602698,
5.89048081903805));
#11998=CARTESIAN_POINT('Ctrl Pts',(-16.7791210646139,-11.65319359751,5.77933967150903));
#11999=CARTESIAN_POINT('Ctrl Pts',(-17.353819766817,-9.40179156583393,5.66819852398001));
#12000=CARTESIAN_POINT('Ctrl Pts',(-15.7739249147585,-7.69796588935184,
5.55705737645099));
#12001=CARTESIAN_POINT('Ctrl Pts',(-13.4856097934235,-8.10133122228054,
5.44591622892198));
#12002=CARTESIAN_POINT('Ctrl Pts',(-12.583507594572,-10.2426628903111,5.33477508139295));
#12003=CARTESIAN_POINT('Ctrl Pts',(-13.8933670056466,-12.161870541709,5.22363393386393));
#12004=CARTESIAN_POINT('Ctrl Pts',(-16.2161945081267,-12.1021873709018,
5.11249278633491));
#12005=CARTESIAN_POINT('Ctrl Pts',(-17.4257656411002,-10.1182449922637,
5.00135163880589));
#12006=CARTESIAN_POINT('Ctrl Pts',(-16.4148868108254,-8.02606582271751,
4.89021049127687));
#12007=CARTESIAN_POINT('Ctrl Pts',(-14.1088765326179,-7.74074795791574,
4.77906934374786));
#12008=CARTESIAN_POINT('Ctrl Pts',(-12.6185654451633,-9.52346009110162,
4.66792819621883));
#12009=CARTESIAN_POINT('Ctrl Pts',(-13.3081253972587,-11.7423780164876,
4.55678704868982));
#12010=CARTESIAN_POINT('Ctrl Pts',(-15.5463604710685,-12.3663919919164,
4.44564590116079));
#12011=CARTESIAN_POINT('Ctrl Pts',(-17.2844787704667,-10.8243042951685,
4.33450475363178));
#12012=CARTESIAN_POINT('Ctrl Pts',(-16.9314755221013,-8.52768103616449,
4.22336360610275));
#12013=CARTESIAN_POINT('Ctrl Pts',(-14.8104759432562,-7.57876034732949,
4.11222245857374));
#12014=CARTESIAN_POINT('Ctrl Pts',(-12.8629591929671,-8.84614671087597,
4.00108131104471));
#12015=CARTESIAN_POINT('Ctrl Pts',(-12.8716051077936,-11.1697247567595,
3.88994016351569));
#12016=CARTESIAN_POINT('Ctrl Pts',(-14.8284995591272,-12.4225830063246,
3.77879901598667));
#12017=CARTESIAN_POINT('Ctrl Pts',(-16.9423787336263,-11.4579045506812,
3.66765786845765));
#12018=CARTESIAN_POINT('Ctrl Pts',(-17.2782812088839,-9.15871790879045,
3.55651672092864));
#12019=CARTESIAN_POINT('Ctrl Pts',(-15.5287351392234,-7.62960763240948,
3.44537557339961));
#12020=CARTESIAN_POINT('Ctrl Pts',(-13.2952058270941,-8.27026081396139,
3.33423442587059));
#12021=CARTESIAN_POINT('Ctrl Pts',(-12.6221777004152,-10.4942488597207,
3.22309327834158));
#12022=CARTESIAN_POINT('Ctrl Pts',(-14.1257140976557,-12.2658210399188,
3.11195213081255));
#12023=CARTESIAN_POINT('Ctrl Pts',(-16.429537244274,-11.9633502210594,3.00081098328354));
#12024=CARTESIAN_POINT('Ctrl Pts',(-17.4248185154485,-9.8637062328524,2.88966983575451));
#12025=CARTESIAN_POINT('Ctrl Pts',(-16.2005167846521,-7.88882016989784,
2.77852868822549));
#12026=CARTESIAN_POINT('Ctrl Pts',(-13.8773094527777,-7.84642465758702,
2.66738754069648));
#12027=CARTESIAN_POINT('Ctrl Pts',(-12.5817686609856,-9.7753268677064,2.55624639316746));
#12028=CARTESIAN_POINT('Ctrl Pts',(-13.4997812308935,-11.9098859856603,
2.44510524563844));
#12029=CARTESIAN_POINT('Ctrl Pts',(-15.7910347483105,-12.2962109712173,
2.33396409810941));
#12030=CARTESIAN_POINT('Ctrl Pts',(-17.3582063339697,-10.5806752356971,
2.2228229505804));
#12031=CARTESIAN_POINT('Ctrl Pts',(-16.7667690699872,-8.33361230926411,
2.11168180305138));
#12032=CARTESIAN_POINT('Ctrl Pts',(-14.5581012599229,-7.61189486585896,
2.00054065552235));
#12033=CARTESIAN_POINT('Ctrl Pts',(-12.7539300664426,-9.07615430524727,
1.88939950799334));
#12034=CARTESIAN_POINT('Ctrl Pts',(-13.0057225272674,-11.3860658425327,
1.77825836046431));
#12035=CARTESIAN_POINT('Ctrl Pts',(-15.0829976689147,-12.4272269759234,
1.6671172129353));
#12036=CARTESIAN_POINT('Ctrl Pts',(-17.0843001660214,-11.2466015268631,
1.55597606540628));
#12037=CARTESIAN_POINT('Ctrl Pts',(-17.1777164239143,-8.92488433131005,
1.44483491787726));
#12038=CARTESIAN_POINT('Ctrl Pts',(-15.2777376918069,-7.58728937837554,
1.33369377034824));
#12039=CARTESIAN_POINT('Ctrl Pts',(-13.1235278364479,-8.45818684891592,
1.22255262281922));
#12040=CARTESIAN_POINT('Ctrl Pts',(-12.686968390135,-10.7404136399833,1.1114114752902));
#12041=CARTESIAN_POINT('Ctrl Pts',(-14.367662797513,-12.344866918125,1.00027032776118));
#12042=CARTESIAN_POINT('Ctrl Pts',(-16.6271811117211,-11.8029762647123,
0.889129180232156));
#12043=CARTESIAN_POINT('Ctrl Pts',(-17.3972277645898,-9.61060671549959,
0.777988032703138));
#12044=CARTESIAN_POINT('Ctrl Pts',(-15.9729748140483,-7.77487725906727,
0.666846885174117));
#12045=CARTESIAN_POINT('Ctrl Pts',(-13.6580450846071,-7.97554008402429,
0.555705737645098));
#12046=CARTESIAN_POINT('Ctrl Pts',(-12.5715926480149,-10.0300833696701,
0.444564590116077));
#12047=CARTESIAN_POINT('Ctrl Pts',(-13.7078055175393,-12.0555949236832,
0.333423442587058));
#12048=CARTESIAN_POINT('Ctrl Pts',(-16.0272313718098,-12.2024171088693,
0.222282295058038));
#12049=CARTESIAN_POINT('Ctrl Pts',(-17.4056531503688,-10.3273325248541,
0.111141147529018));
#12050=CARTESIAN_POINT('Ctrl Pts',(-16.8572712062568,-8.88671494767186,
0.0370470491763382));
#12051=CARTESIAN_POINT('Ctrl Pts',(-16.3390017195986,-8.44145197141311,
-2.22044604925031E-15));
#12052=CARTESIAN_POINT('Ctrl Pts',(-16.3390017195986,-8.44145197141311,
-2.22044604925031E-15));
#12053=CARTESIAN_POINT('Ctrl Pts',(-16.3898412550158,-8.49415674362063,
-2.22613706717393E-15));
#12054=CARTESIAN_POINT('Ctrl Pts',(-16.4374589296418,-8.54962581051277,
-1.71409610791473E-15));
#12055=CARTESIAN_POINT('Ctrl Pts',(-16.4818118062285,-8.60751256073212,
-1.85962356624714E-15));
#12056=CARTESIAN_POINT('Ctrl Pts',(-16.5273944148942,-8.66700428449924,
-2.00918593274442E-15));
#12057=CARTESIAN_POINT('Ctrl Pts',(-16.5695290717974,-8.7290505709106,-1.66395111688824E-15));
#12058=CARTESIAN_POINT('Ctrl Pts',(-16.6081216798471,-8.79330183658361,
-1.58206781009085E-15));
#12059=CARTESIAN_POINT('Ctrl Pts',(-16.640731850897,-8.84759318587709,-1.51287765229278E-15));
#12060=CARTESIAN_POINT('Ctrl Pts',(-16.6708122443294,-8.90345969057086,
-3.85227514727774E-17));
#12061=CARTESIAN_POINT('Ctrl Pts',(-16.6982777801774,-8.96069680171699,
-1.38777878078145E-16));
#12062=CARTESIAN_POINT('Ctrl Pts',(-16.7104763391781,-8.98611812541558,
-1.83305248080649E-16));
#12063=CARTESIAN_POINT('Ctrl Pts',(-16.7221587384426,-9.01180984573392,
-1.61721416497441E-15));
#12064=CARTESIAN_POINT('Ctrl Pts',(-16.7333158123914,-9.0377540202666,-1.74860126378462E-15));
#12065=CARTESIAN_POINT('Ctrl Pts',(-16.7394484186841,-9.05201451622892,
-1.82081960280802E-15));
#12066=CARTESIAN_POINT('Ctrl Pts',(-16.7454222912401,-9.06635128371498,
-1.59328855671869E-15));
#12067=CARTESIAN_POINT('Ctrl Pts',(-16.7512357689513,-9.08076132240649,
-1.66533453693773E-15));
#12068=CARTESIAN_POINT('Ctrl Pts',(-16.7565954716119,-9.09404657549439,
-1.73175691800603E-15));
#12069=CARTESIAN_POINT('Ctrl Pts',(-16.761819475366,-9.10739609302559,-3.43152104970979E-15));
#12070=CARTESIAN_POINT('Ctrl Pts',(-16.7668988698636,-9.12078671142655,
-3.3584246494911E-15));
#12071=CARTESIAN_POINT('Ctrl Pts',(-16.792860351532,-9.18922799794368,-2.98481892636936E-15));
#12072=CARTESIAN_POINT('Ctrl Pts',(-16.8150968550578,-9.2588588983408,3.9807706675476E-16));
#12073=CARTESIAN_POINT('Ctrl Pts',(-16.833523678901,-9.32935115717727,4.9960036108132E-16));
#12074=CARTESIAN_POINT('Ctrl Pts',(-16.851806919093,-9.39929413329465,6.00332575761995E-16));
#12075=CARTESIAN_POINT('Ctrl Pts',(-16.8663396941486,-9.47008611206394,
-1.23947449676468E-16));
#12076=CARTESIAN_POINT('Ctrl Pts',(-16.8769883967272,-9.54140886116961,
3.88578058618805E-16));
#12077=CARTESIAN_POINT('Ctrl Pts',(-16.8858394571407,-9.60069138470125,
8.14582466568122E-16));
#12078=CARTESIAN_POINT('Ctrl Pts',(-16.8920062609022,-9.66034091039286,
-3.79887144988971E-15));
#12079=CARTESIAN_POINT('Ctrl Pts',(-16.8953843819236,-9.72016855746037,
-4.21884749357559E-15));
#12080=CARTESIAN_POINT('Ctrl Pts',(-16.8967942299417,-9.74513743486574,
-4.39412315394293E-15));
#12081=CARTESIAN_POINT('Ctrl Pts',(-16.897718042808,-9.77013723287953,-1.04049734037864E-15));
#12082=CARTESIAN_POINT('Ctrl Pts',(-16.8981468950099,-9.79515367142193,
-1.16573417585641E-15));
#12083=CARTESIAN_POINT('Ctrl Pts',(-16.8983454979286,-9.80673886950697,
-1.22373178187433E-15));
#12084=CARTESIAN_POINT('Ctrl Pts',(-16.8984379380574,-9.81832763098025,
-2.19002109012887E-15));
#12085=CARTESIAN_POINT('Ctrl Pts',(-16.8984232708294,-9.82991850741629,
-2.35922392732846E-15));
#12086=CARTESIAN_POINT('Ctrl Pts',(-16.898407987489,-9.8419962708459,-2.53553430822076E-15));
#12087=CARTESIAN_POINT('Ctrl Pts',(-16.898276391407,-9.85406801930843,2.2754508191584E-15));
#12088=CARTESIAN_POINT('Ctrl Pts',(-16.8980280297643,-9.86612772948922,
2.24820162486594E-15));
#12089=CARTESIAN_POINT('Ctrl Pts',(-16.896612869921,-9.93484372517432,2.09293624208695E-15));
#12090=CARTESIAN_POINT('Ctrl Pts',(-16.8914106127702,-10.0032167380162,
-1.36002320516582E-15));
#12091=CARTESIAN_POINT('Ctrl Pts',(-16.8823084122723,-10.0709659878617,
-1.36002320516582E-15));
#12092=CARTESIAN_POINT('Ctrl Pts',(-16.874055619439,-10.1323929498053,-1.36002320516582E-15));
#12093=CARTESIAN_POINT('Ctrl Pts',(-16.862596252108,-10.1933075358049,-1.26372848136827E-15));
#12094=CARTESIAN_POINT('Ctrl Pts',(-16.8478109454459,-10.2534888721422,
-1.38777878078145E-15));
#12095=CARTESIAN_POINT('Ctrl Pts',(-16.8303241431413,-10.3246662345746,
-1.52144137683588E-15));
#12096=CARTESIAN_POINT('Ctrl Pts',(-16.8081848462467,-10.3948195464577,
1.0568803955417E-15));
#12097=CARTESIAN_POINT('Ctrl Pts',(-16.7816446910013,-10.4635997456855,
9.15933995315754E-16));
#12098=CARTESIAN_POINT('Ctrl Pts',(-16.7758002954335,-10.47874580221,8.84896252350212E-16));
#12099=CARTESIAN_POINT('Ctrl Pts',(-16.7697423260011,-10.4938251023906,
3.43889358474875E-15));
#12100=CARTESIAN_POINT('Ctrl Pts',(-16.76347320795,-10.5088336097722,3.58046925441613E-15));
#12101=CARTESIAN_POINT('Ctrl Pts',(-16.757017516591,-10.5242887807586,3.72625831435445E-15));
#12102=CARTESIAN_POINT('Ctrl Pts',(-16.7503352761988,-10.5396743969356,
1.17227682962454E-15));
#12103=CARTESIAN_POINT('Ctrl Pts',(-16.7434433794614,-10.5549551926611,
1.11022302462516E-15));
#12104=CARTESIAN_POINT('Ctrl Pts',(-16.7152442624164,-10.6174786116301,
8.56321583999907E-16));
#12105=CARTESIAN_POINT('Ctrl Pts',(-16.6835079213234,-10.678330876987,-5.09021181669685E-16));
#12106=CARTESIAN_POINT('Ctrl Pts',(-16.6484901027957,-10.7372591681392,
-6.24500451351651E-16));
#12107=CARTESIAN_POINT('Ctrl Pts',(-16.6134795778401,-10.7961751856045,
-7.39955668810536E-16));
#12108=CARTESIAN_POINT('Ctrl Pts',(-16.5751880678017,-10.8531687996888,
-5.44190642062304E-16));
#12109=CARTESIAN_POINT('Ctrl Pts',(-16.5338329814792,-10.9079522899894,
-1.36002320516582E-15));
#12110=CARTESIAN_POINT('Ctrl Pts',(-16.5038966901276,-10.9476091900891,
-1.95059146351222E-15));
#12111=CARTESIAN_POINT('Ctrl Pts',(-16.4723542281424,-10.9861072729443,
3.54640415640727E-16));
#12112=CARTESIAN_POINT('Ctrl Pts',(-16.4392794411118,-11.023322519061,4.23272528138341E-16));
#12113=CARTESIAN_POINT('Ctrl Pts',(-16.4144728570297,-11.0512345092751,
4.74747637194398E-16));
#12114=CARTESIAN_POINT('Ctrl Pts',(-16.3888041482335,-11.078424626853,-2.43914533858063E-18));
#12115=CARTESIAN_POINT('Ctrl Pts',(-16.3623027552176,-11.1048350815606,
-1.2490009027033E-16));
#12116=CARTESIAN_POINT('Ctrl Pts',(-16.3534958039143,-11.1136118122165,
-1.65596350195737E-16));
#12117=CARTESIAN_POINT('Ctrl Pts',(-16.344603778745,-11.1222955249443,1.47368254087686E-15));
#12118=CARTESIAN_POINT('Ctrl Pts',(-16.3356283270931,-11.1308842376674,
1.38083988687754E-15));
#12119=CARTESIAN_POINT('Ctrl Pts',(-16.288023609681,-11.1764377382574,8.88413602512318E-16));
#12120=CARTESIAN_POINT('Ctrl Pts',(-16.2380710211992,-11.2193250402242,
1.04010533930317E-15));
#12121=CARTESIAN_POINT('Ctrl Pts',(-16.1859608069979,-11.2592665759842,
1.45716771982052E-15));
#12122=CARTESIAN_POINT('Ctrl Pts',(-16.1492839781811,-11.2873787012596,
1.75070950947919E-15));
#12123=CARTESIAN_POINT('Ctrl Pts',(-16.1115377653254,-11.3140307077825,
1.50961177331903E-15));
#12124=CARTESIAN_POINT('Ctrl Pts',(-16.0727840466388,-11.3391103479433,
1.30104260698261E-15));
#12125=CARTESIAN_POINT('Ctrl Pts',(-16.0603479160929,-11.3471584447364,
1.23411242664593E-15));
#12126=CARTESIAN_POINT('Ctrl Pts',(-16.0478062717038,-11.3550455819844,
3.29476744426013E-15));
#12127=CARTESIAN_POINT('Ctrl Pts',(-16.035166679802,-11.3627643666854,3.46944695195361E-15));
#12128=CARTESIAN_POINT('Ctrl Pts',(-15.9813223879855,-11.3956461637514,
4.21357654567057E-15));
#12129=CARTESIAN_POINT('Ctrl Pts',(-15.9258102639214,-11.4254113967777,
2.49285835226939E-15));
#12130=CARTESIAN_POINT('Ctrl Pts',(-15.8687981257942,-11.4517907020109,
7.73686670285656E-16));
#12131=CARTESIAN_POINT('Ctrl Pts',(-15.8162031923817,-11.4761261829765,
-8.1228647698802E-16));
#12132=CARTESIAN_POINT('Ctrl Pts',(-15.7623311074045,-11.4975799204738,
-1.81768923500598E-15));
#12133=CARTESIAN_POINT('Ctrl Pts',(-15.7073085825,-11.5159013381686,-2.16320017454308E-15));
#12134=CARTESIAN_POINT('Ctrl Pts',(-15.6970482491915,-11.5193178271894,
-2.23227875911951E-15));
#12135=CARTESIAN_POINT('Ctrl Pts',(-15.6867479087967,-11.522625281403,-1.49184837699714E-15));
#12136=CARTESIAN_POINT('Ctrl Pts',(-15.6764092460937,-11.5258237909713,
-1.51267887105178E-15));
#12137=CARTESIAN_POINT('Ctrl Pts',(-13.1992962903993,-10.0024064022658,
8.));
#12138=CARTESIAN_POINT('Ctrl Pts',(-13.1914749172297,-10.0697907508692,
8.));
#12139=CARTESIAN_POINT('Ctrl Pts',(-13.187400594648,-10.13757275596,8.));
#12140=CARTESIAN_POINT('Ctrl Pts',(-13.1871885483144,-10.2054359876388,
8.));
#12141=CARTESIAN_POINT('Ctrl Pts',(-13.1871289997272,-10.2244938958915,
8.));
#12142=CARTESIAN_POINT('Ctrl Pts',(-13.1873743545316,-10.243558269923,8.));
#12143=CARTESIAN_POINT('Ctrl Pts',(-13.1879279070141,-10.2626221926416,
8.));
#12144=CARTESIAN_POINT('Ctrl Pts',(-13.1882788291768,-10.2747076826339,
8.));
#12145=CARTESIAN_POINT('Ctrl Pts',(-13.188753786007,-10.2867946010088,8.));
#12146=CARTESIAN_POINT('Ctrl Pts',(-13.1893525572532,-10.2988636614694,
8.));
#12147=CARTESIAN_POINT('Ctrl Pts',(-13.1928456546243,-10.3692718576439,
8.));
#12148=CARTESIAN_POINT('Ctrl Pts',(-13.200551400234,-10.4392065520031,8.));
#12149=CARTESIAN_POINT('Ctrl Pts',(-13.2125313402152,-10.5083097512027,
8.));
#12150=CARTESIAN_POINT('Ctrl Pts',(-13.2141825349725,-10.5178342430122,
8.));
#12151=CARTESIAN_POINT('Ctrl Pts',(-13.2159150020402,-10.527342969275,8.));
#12152=CARTESIAN_POINT('Ctrl Pts',(-13.2177289760061,-10.5368350182323,
8.));
#12153=CARTESIAN_POINT('Ctrl Pts',(-13.2303840186811,-10.6030555301501,
8.));
#12154=CARTESIAN_POINT('Ctrl Pts',(-13.2470016652037,-10.6684641941904,
8.));
#12155=CARTESIAN_POINT('Ctrl Pts',(-13.2673108671637,-10.732853414775,8.));
#12156=CARTESIAN_POINT('Ctrl Pts',(-13.2891629308514,-10.8021341945802,
8.));
#12157=CARTESIAN_POINT('Ctrl Pts',(-13.3152885233548,-10.8702357394381,
8.));
#12158=CARTESIAN_POINT('Ctrl Pts',(-13.3454140237584,-10.9368936728771,
8.));
#12159=CARTESIAN_POINT('Ctrl Pts',(-13.3509664607591,-10.9491794099123,
8.));
#12160=CARTESIAN_POINT('Ctrl Pts',(-13.3566549432153,-10.9614160670129,
8.));
#12161=CARTESIAN_POINT('Ctrl Pts',(-13.3624779793227,-10.9736019244815,
8.));
#12162=CARTESIAN_POINT('Ctrl Pts',(-13.3674124355839,-10.9839282524614,
8.));
#12163=CARTESIAN_POINT('Ctrl Pts',(-13.3724393907479,-10.9942094580485,
8.));
#12164=CARTESIAN_POINT('Ctrl Pts',(-13.3775570341231,-11.004443789421,8.));
#12165=CARTESIAN_POINT('Ctrl Pts',(-13.4093429320592,-11.0680096514008,
8.));
#12166=CARTESIAN_POINT('Ctrl Pts',(-13.4446277894419,-11.1297776805203,
8.));
#12167=CARTESIAN_POINT('Ctrl Pts',(-13.4831035148986,-11.1895235034675,
8.));
#12168=CARTESIAN_POINT('Ctrl Pts',(-13.5223919592831,-11.2505313314996,
8.));
#12169=CARTESIAN_POINT('Ctrl Pts',(-13.5650078538732,-11.3094314878199,
8.));
#12170=CARTESIAN_POINT('Ctrl Pts',(-13.6106776763614,-11.365976797792,8.));
#12171=CARTESIAN_POINT('Ctrl Pts',(-13.6566254157242,-11.4228662057914,
8.));
#12172=CARTESIAN_POINT('Ctrl Pts',(-13.7056649005089,-11.4773729508705,
8.));
#12173=CARTESIAN_POINT('Ctrl Pts',(-13.7575651962072,-11.5292234094565,
8.));
#12174=CARTESIAN_POINT('Ctrl Pts',(-13.770395915342,-11.5420418079294,8.));
#12175=CARTESIAN_POINT('Ctrl Pts',(-13.7834016831258,-11.5546977194546,
8.));
#12176=CARTESIAN_POINT('Ctrl Pts',(-13.7965793954044,-11.5671867011474,
8.));
#12177=CARTESIAN_POINT('Ctrl Pts',(-13.8068738937706,-11.5769431595457,
8.));
#12178=CARTESIAN_POINT('Ctrl Pts',(-13.8172745884826,-11.5865987303042,
8.));
#12179=CARTESIAN_POINT('Ctrl Pts',(-13.8277639078832,-11.5961370139814,
8.));
#12180=CARTESIAN_POINT('Ctrl Pts',(-13.8835125900578,-11.6468311271936,
8.));
#12181=CARTESIAN_POINT('Ctrl Pts',(-13.941858687196,-11.6943084473716,8.));
#12182=CARTESIAN_POINT('Ctrl Pts',(-14.0025044412164,-11.7383154250973,
8.));
#12183=CARTESIAN_POINT('Ctrl Pts',(-14.0632169827124,-11.7823708664787,
8.));
#12184=CARTESIAN_POINT('Ctrl Pts',(-14.1262348879421,-11.8229492486321,
8.));
#12185=CARTESIAN_POINT('Ctrl Pts',(-14.1913041337018,-11.8597697342368,
8.));
#12186=CARTESIAN_POINT('Ctrl Pts',(-14.2548907820865,-11.8957512681268,
8.));
#12187=CARTESIAN_POINT('Ctrl Pts',(-14.320437088868,-11.9281449399806,8.));
#12188=CARTESIAN_POINT('Ctrl Pts',(-14.3877383201204,-11.9566513247419,
8.));
#12189=CARTESIAN_POINT('Ctrl Pts',(-14.4022443265699,-11.9627955481611,
8.));
#12190=CARTESIAN_POINT('Ctrl Pts',(-14.4168319601953,-11.9687590163805,
8.));
#12191=CARTESIAN_POINT('Ctrl Pts',(-14.4314993237549,-11.9745384454386,
8.));
#12192=CARTESIAN_POINT('Ctrl Pts',(-14.4438535969467,-11.9794064399618,
8.));
#12193=CARTESIAN_POINT('Ctrl Pts',(-14.4562644367296,-11.9841438631167,
8.));
#12194=CARTESIAN_POINT('Ctrl Pts',(-14.4687300448211,-11.9887511357905,
8.));
#12195=CARTESIAN_POINT('Ctrl Pts',(-13.7309291201476,-8.92064134695149,
8.));
#12196=CARTESIAN_POINT('Ctrl Pts',(-13.6852992237889,-8.96320919740821,
8.));
#12197=CARTESIAN_POINT('Ctrl Pts',(-13.6424343385012,-9.00837891446438,
8.));
#12198=CARTESIAN_POINT('Ctrl Pts',(-13.6023333218234,-9.05579903672846,
8.));
#12199=CARTESIAN_POINT('Ctrl Pts',(-13.5611744803124,-9.10447005453275,
8.));
#12200=CARTESIAN_POINT('Ctrl Pts',(-13.5229267493543,-9.15551228037441,
8.));
#12201=CARTESIAN_POINT('Ctrl Pts',(-13.4876147577988,-9.20859491497877,
8.));
#12202=CARTESIAN_POINT('Ctrl Pts',(-13.4504234878807,-9.26450256857094,
8.));
#12203=CARTESIAN_POINT('Ctrl Pts',(-13.4164879292609,-9.32267412786545,
8.));
#12204=CARTESIAN_POINT('Ctrl Pts',(-13.3858756344612,-9.38276912102125,
8.));
#12205=CARTESIAN_POINT('Ctrl Pts',(-13.3760567911501,-9.40204449143826,
8.));
#12206=CARTESIAN_POINT('Ctrl Pts',(-13.3665801818845,-9.42151804589282,
8.));
#12207=CARTESIAN_POINT('Ctrl Pts',(-13.3574490403934,-9.44117931849771,
8.));
#12208=CARTESIAN_POINT('Ctrl Pts',(-13.3522109746218,-9.45245797836281,
8.));
#12209=CARTESIAN_POINT('Ctrl Pts',(-13.3470863249925,-9.46379928849863,
8.));
#12210=CARTESIAN_POINT('Ctrl Pts',(-13.3420822593818,-9.47518585358561,
8.));
#12211=CARTESIAN_POINT('Ctrl Pts',(-13.315074917903,-9.53664005412922,8.));
#12212=CARTESIAN_POINT('Ctrl Pts',(-13.2915286665307,-9.59951131295569,
8.));
#12213=CARTESIAN_POINT('Ctrl Pts',(-13.2714786288552,-9.66344604206431,
8.));
#12214=CARTESIAN_POINT('Ctrl Pts',(-13.251118980486,-9.72836804492028,8.));
#12215=CARTESIAN_POINT('Ctrl Pts',(-13.2343637932416,-9.79438749311294,
8.));
#12216=CARTESIAN_POINT('Ctrl Pts',(-13.2212910825401,-9.86116786571081,
8.));
#12217=CARTESIAN_POINT('Ctrl Pts',(-13.2148890447258,-9.89387190700605,
8.));
#12218=CARTESIAN_POINT('Ctrl Pts',(-13.2093708532485,-9.92675886633403,
8.));
#12219=CARTESIAN_POINT('Ctrl Pts',(-13.2047498322757,-9.95979108763484,
8.));
#12220=CARTESIAN_POINT('Ctrl Pts',(-13.2027644288902,-9.97398325087913,
8.));
#12221=CARTESIAN_POINT('Ctrl Pts',(-13.2009464686606,-9.98818943744355,
8.));
#12222=CARTESIAN_POINT('Ctrl Pts',(-13.1992962903989,-10.0024064022693,
8.));
#12223=CARTESIAN_POINT('Ctrl Pts',(-16.6673099838652,-10.001299617498,6.87148036339021));
#12224=CARTESIAN_POINT('Ctrl Pts',(-16.6680396077119,-10.0863816229506,
6.87718308383008));
#12225=CARTESIAN_POINT('Ctrl Pts',(-16.6620894467177,-10.1713612071089,
6.88288580426994));
#12226=CARTESIAN_POINT('Ctrl Pts',(-16.6491047202909,-10.2552518596557,
6.8885885247098));
#12227=CARTESIAN_POINT('Ctrl Pts',(-16.5647509800805,-10.8002375665841,
6.92563557388614));
#12228=CARTESIAN_POINT('Ctrl Pts',(-16.1835176418883,-11.2992671185536,
6.96268262306248));
#12229=CARTESIAN_POINT('Ctrl Pts',(-15.6798879029899,-11.5239558279272,
6.99972967223882));
#12230=CARTESIAN_POINT('Ctrl Pts',(-15.1762581640915,-11.7486445373009,
7.03677672141516));
#12231=CARTESIAN_POINT('Ctrl Pts',(-14.5502320244869,-11.6989924040788,
7.0738237705915));
#12232=CARTESIAN_POINT('Ctrl Pts',(-14.0883288184045,-11.3977023782804,
7.11087081976784));
#12233=CARTESIAN_POINT('Ctrl Pts',(-13.6264256123221,-11.0964123524819,
7.14791786894418));
#12234=CARTESIAN_POINT('Ctrl Pts',(-13.3286453397619,-10.5434844341071,
7.18496491812052));
#12235=CARTESIAN_POINT('Ctrl Pts',(-13.3312770262637,-9.99202514980564,
7.22201196729686));
#12236=CARTESIAN_POINT('Ctrl Pts',(-13.3339087127654,-9.44056586550417,
7.2590590164732));
#12237=CARTESIAN_POINT('Ctrl Pts',(-13.6369523583291,-8.89057521527605,
7.29610606564954));
#12238=CARTESIAN_POINT('Ctrl Pts',(-14.1017091677237,-8.59369096597919,
7.33315311482588));
#12239=CARTESIAN_POINT('Ctrl Pts',(-14.5664659771184,-8.29680671668234,
7.37020016400222));
#12240=CARTESIAN_POINT('Ctrl Pts',(-15.192935950344,-8.25302886831675,7.40724721317856));
#12241=CARTESIAN_POINT('Ctrl Pts',(-15.6943994886325,-8.48255279837451,
7.4442942623549));
#12242=CARTESIAN_POINT('Ctrl Pts',(-16.195863026921,-8.71207672843227,7.48134131153124));
#12243=CARTESIAN_POINT('Ctrl Pts',(-16.5723201302723,-9.21490243691337,
7.51838836070758));
#12244=CARTESIAN_POINT('Ctrl Pts',(-16.6514672697293,-9.76058778570281,
7.55543540988392));
#12245=CARTESIAN_POINT('Ctrl Pts',(-16.6628933904863,-9.83936595423039,
7.56078372771935));
#12246=CARTESIAN_POINT('Ctrl Pts',(-16.6681231513107,-9.9190373782495,7.56613204555478));
#12247=CARTESIAN_POINT('Ctrl Pts',(-16.6674570171079,-9.99879340680734,
7.57148036339021));
#12248=CARTESIAN_POINT('Ctrl Pts',(-15.5301702171886,-11.9851743256717,
8.));
#12249=CARTESIAN_POINT('Ctrl Pts',(-16.1903072548812,-11.8088749487748,
7.96295295082366));
#12250=CARTESIAN_POINT('Ctrl Pts',(-17.3094427799721,-10.7488569090756,
7.88885885247098));
#12251=CARTESIAN_POINT('Ctrl Pts',(-16.8810965229137,-8.46138998352444,
7.77771770494196));
#12252=CARTESIAN_POINT('Ctrl Pts',(-14.727662200004,-7.58731060863186,7.66657655741293));
#12253=CARTESIAN_POINT('Ctrl Pts',(-12.8251332301876,-8.91924943693317,
7.55543540988393));
#12254=CARTESIAN_POINT('Ctrl Pts',(-12.9125601407559,-11.2417229038903,
7.4442942623549));
#12255=CARTESIAN_POINT('Ctrl Pts',(-14.9111754350777,-12.4269243298781,
7.33315311482589));
#12256=CARTESIAN_POINT('Ctrl Pts',(-16.9908762005917,-11.3909493725631,
7.22201196729686));
#12257=CARTESIAN_POINT('Ctrl Pts',(-17.2483216335285,-9.08158193933239,
7.11087081976785));
#12258=CARTESIAN_POINT('Ctrl Pts',(-15.4476835001917,-7.61298704116733,
6.99972967223882));
#12259=CARTESIAN_POINT('Ctrl Pts',(-13.2372839439424,-8.32932353917012,
6.88858852470981));
#12260=CARTESIAN_POINT('Ctrl Pts',(-12.64038931445,-10.5749548961775,6.77744737718078));
#12261=CARTESIAN_POINT('Ctrl Pts',(-14.2033970972384,-12.2942830560246,
6.66630622965177));
#12262=CARTESIAN_POINT('Ctrl Pts',(-16.4955795141811,-11.9135215156732,
6.55516508212274));
#12263=CARTESIAN_POINT('Ctrl Pts',(-17.4187697235728,-9.78119478057994,
6.44402393459372));
#12264=CARTESIAN_POINT('Ctrl Pts',(-16.1279126463626,-7.84915537048691,
6.3328827870647));
#12265=CARTESIAN_POINT('Ctrl Pts',(-13.8046094981315,-7.88591323323186,
6.22174163953568));
#12266=CARTESIAN_POINT('Ctrl Pts',(-12.5755192591945,-9.85782298675155,
6.11060049200667));
#12267=CARTESIAN_POINT('Ctrl Pts',(-13.5657029889766,-11.9598757266924,
5.99945934447763));
#12268=CARTESIAN_POINT('Ctrl Pts',(-15.8687854179254,-12.2679358305796,
5.88831819694863));
#12269=CARTESIAN_POINT('Ctrl Pts',(-17.3766160640088,-10.5000170785009,
5.7771770494196));
#12270=CARTESIAN_POINT('Ctrl Pts',(-16.7089863056128,-8.27440249298907,
5.66603590189059));
#12271=CARTESIAN_POINT('Ctrl Pts',(-14.4770180600175,-7.62833162617035,
5.55489475436157));
#12272=CARTESIAN_POINT('Ctrl Pts',(-12.7237668001956,-9.15319223134576,
5.44375360683254));
#12273=CARTESIAN_POINT('Ctrl Pts',(-13.0540894216228,-11.4531871843689,
5.33261245930352));
#12274=CARTESIAN_POINT('Ctrl Pts',(-15.1656216518599,-12.4229920439975,
5.22147131177451));
#12275=CARTESIAN_POINT('Ctrl Pts',(-17.1255503707361,-11.1748857803501,
5.11033016424548));
#12276=CARTESIAN_POINT('Ctrl Pts',(-17.1398343152041,-8.85133552402972,
4.99918901671647));
#12277=CARTESIAN_POINT('Ctrl Pts',(-15.1953985278237,-7.57922731532253,
4.88804786918744));
#12278=CARTESIAN_POINT('Ctrl Pts',(-13.0721026532078,-8.52299871511589,
4.77690672165843));
#12279=CARTESIAN_POINT('Ctrl Pts',(-12.7135277889139,-10.818758696566,4.6657655741294));
#12280=CARTESIAN_POINT('Ctrl Pts',(-14.4478991890863,-12.3650593375113,
4.55462442660038));
#12281=CARTESIAN_POINT('Ctrl Pts',(-16.6876418438301,-11.7464781654166,
4.44348327907137));
#12282=CARTESIAN_POINT('Ctrl Pts',(-17.3825838770138,-9.52923992914208,
4.33234213154235));
#12283=CARTESIAN_POINT('Ctrl Pts',(-15.8966028265696,-7.74291684984371,
4.22120098401332));
#12284=CARTESIAN_POINT('Ctrl Pts',(-13.5899069966017,-8.02263845058788,
4.11005983648432));
#12285=CARTESIAN_POINT('Ctrl Pts',(-12.5739545527748,-10.1123586370691,
3.99891868895528));
#12286=CARTESIAN_POINT('Ctrl Pts',(-13.7787081956621,-12.0992301693682,
3.88777754142627));
#12287=CARTESIAN_POINT('Ctrl Pts',(-16.1013840714784,-12.1645493993947,
3.77663639389725));
#12288=CARTESIAN_POINT('Ctrl Pts',(-17.4158965123757,-10.248525686433,3.66549524636823));
#12289=CARTESIAN_POINT('Ctrl Pts',(-16.5189928002739,-8.10501138577344,
3.55435409883921));
#12290=CARTESIAN_POINT('Ctrl Pts',(-14.2316631334124,-7.69609474266784,
3.44321295131019));
#12291=CARTESIAN_POINT('Ctrl Pts',(-12.647638657407,-9.39608188535426,3.33207180378117));
#12292=CARTESIAN_POINT('Ctrl Pts',(-13.2168727518909,-11.6488717938068,
3.22093065625215));
#12293=CARTESIAN_POINT('Ctrl Pts',(-15.4183110319232,-12.3923496516694,
3.10978950872312));
#12294=CARTESIAN_POINT('Ctrl Pts',(-17.2368439315762,-10.9459652219235,
2.99864836119411));
#12295=CARTESIAN_POINT('Ctrl Pts',(-17.0078583317483,-8.63368162744371,
2.88750721366509));
#12296=CARTESIAN_POINT('Ctrl Pts',(-14.9409585972601,-7.57207185286643,
2.77636606613607));
#12297=CARTESIAN_POINT('Ctrl Pts',(-12.9281030287572,-8.73289151373681,
2.66522491860704));
#12298=CARTESIAN_POINT('Ctrl Pts',(-12.8117800332785,-11.0535721874087,
2.55408377107803));
#12299=CARTESIAN_POINT('Ctrl Pts',(-14.6984670829124,-12.4098545333209,
2.442942623549));
#12300=CARTESIAN_POINT('Ctrl Pts',(-16.8611654422835,-11.5602513173828,
2.33180147601999));
#12301=CARTESIAN_POINT('Ctrl Pts',(-17.3202265408315,-9.28245572666732,
2.22066032849097));
#12302=CARTESIAN_POINT('Ctrl Pts',(-15.6554439913718,-7.66147180407228,
2.10951918096195));
#12303=CARTESIAN_POINT('Ctrl Pts',(-13.3906939345767,-8.18108411896286,
1.99837803343293));
#12304=CARTESIAN_POINT('Ctrl Pts',(-12.5990390076834,-10.3656601528754,
1.88723688590391));
#12305=CARTESIAN_POINT('Ctrl Pts',(-14.0051288824869,-12.2155252739355,
1.77609573837489));
#12306=CARTESIAN_POINT('Ctrl Pts',(-16.3218843807385,-12.0373862789351,
1.66495459084587));
#12307=CARTESIAN_POINT('Ctrl Pts',(-17.428639303623,-9.99430418754786,1.55381344331685));
#12308=CARTESIAN_POINT('Ctrl Pts',(-16.3123135839388,-7.95643629520889,
1.44267229578783));
#12309=CARTESIAN_POINT('Ctrl Pts',(-13.9947483624482,-7.78916489875036,
1.33153114825881));
#12310=CARTESIAN_POINT('Ctrl Pts',(-12.5973498364434,-9.64560634071132,
1.22039000072979));
#12311=CARTESIAN_POINT('Ctrl Pts',(-13.3992440433914,-11.826442250177,1.10924885320077));
#12312=CARTESIAN_POINT('Ctrl Pts',(-15.6664035468934,-12.3354318728424,
0.998107705671752));
#12313=CARTESIAN_POINT('Ctrl Pts',(-17.32357021704,-10.7066464303587,0.88696655814273));
#12314=CARTESIAN_POINT('Ctrl Pts',(-16.8538197307884,-8.43105010031595,
0.775825410613713));
#12315=CARTESIAN_POINT('Ctrl Pts',(-14.687180849695,-7.59155940883828,0.664684263084691));
#12316=CARTESIAN_POINT('Ctrl Pts',(-12.8068360000695,-8.95675512341312,
0.553543115555673));
#12317=CARTESIAN_POINT('Ctrl Pts',(-12.9341202906761,-11.2767116091318,
0.442401968026652));
#12318=CARTESIAN_POINT('Ctrl Pts',(-14.9522479049698,-12.4283740802081,
0.331260820497633));
#12319=CARTESIAN_POINT('Ctrl Pts',(-17.0144374426264,-11.3565061871398,
0.220119672968612));
#12320=CARTESIAN_POINT('Ctrl Pts',(-17.2320075214997,-9.04429062969129,
0.108978525439591));
#12321=CARTESIAN_POINT('Ctrl Pts',(-15.407826937649,-7.60427002768573,-0.00216262208942734));
#12322=CARTESIAN_POINT('Ctrl Pts',(-13.2075718205704,-8.36246714664345,
-0.113303769618448));
#12323=CARTESIAN_POINT('Ctrl Pts',(-12.839200671623,-9.85926548464067,-0.187397867971127));
#12324=CARTESIAN_POINT('Ctrl Pts',(-13.0122087991468,-10.5202727210901,
-0.224444917147467));
#12325=CARTESIAN_POINT('Ctrl Pts',(-15.4967348970877,-11.8599788000028,
8.07481497238249));
#12326=CARTESIAN_POINT('Ctrl Pts',(-16.1152402239634,-11.6947977883195,
8.03776792320615));
#12327=CARTESIAN_POINT('Ctrl Pts',(-17.163797181446,-10.7016300569196,7.96367382485347));
#12328=CARTESIAN_POINT('Ctrl Pts',(-16.7624646904471,-8.55842281702485,
7.85253267732444));
#12329=CARTESIAN_POINT('Ctrl Pts',(-14.7448372528894,-7.73946748106473,
7.74139152979544));
#12330=CARTESIAN_POINT('Ctrl Pts',(-12.9622917582753,-8.98740724711157,
7.6302503822664));
#12331=CARTESIAN_POINT('Ctrl Pts',(-13.0442050684083,-11.1634133319412,
7.51910923473739));
#12332=CARTESIAN_POINT('Ctrl Pts',(-14.9167771789417,-12.2738697274138,
7.40796808720837));
#12333=CARTESIAN_POINT('Ctrl Pts',(-16.8653210847252,-11.3032287952692,
7.29682693967936));
#12334=CARTESIAN_POINT('Ctrl Pts',(-17.1065306557073,-9.13950220880304,
7.18568579215032));
#12335=CARTESIAN_POINT('Ctrl Pts',(-15.4194502259573,-7.7635246228271,7.07454464462132));
#12336=CARTESIAN_POINT('Ctrl Pts',(-13.348450082044,-8.43468517670065,6.96340349709229));
#12337=CARTESIAN_POINT('Ctrl Pts',(-12.7891987647493,-10.5386952188625,
6.85226234956327));
#12338=CARTESIAN_POINT('Ctrl Pts',(-14.253635062676,-12.1495935093596,6.74112120203425));
#12339=CARTESIAN_POINT('Ctrl Pts',(-16.4012604102937,-11.79284479276,6.62998005450523));
#12340=CARTESIAN_POINT('Ctrl Pts',(-17.2662293934371,-9.79499378760424,
6.51883890697621));
#12341=CARTESIAN_POINT('Ctrl Pts',(-16.0567805473605,-7.98479893616371,
6.4076977594472));
#12342=CARTESIAN_POINT('Ctrl Pts',(-13.8799971053183,-8.01923865491027,
6.29655661191817));
#12343=CARTESIAN_POINT('Ctrl Pts',(-12.72841975609,-9.86678941639023,6.18541546438916));
#12344=CARTESIAN_POINT('Ctrl Pts',(-13.6561572961568,-11.8362756636269,
6.07427431686014));
#12345=CARTESIAN_POINT('Ctrl Pts',(-15.8139952437406,-12.1249078784139,
5.9631331693311));
#12346=CARTESIAN_POINT('Ctrl Pts',(-17.2267341651754,-10.4684833737895,
5.85199202180211));
#12347=CARTESIAN_POINT('Ctrl Pts',(-16.6012086479404,-8.3832277403185,5.74085087427306));
#12348=CARTESIAN_POINT('Ctrl Pts',(-14.5100000495813,-7.77790149765939,
5.62970972674407));
#12349=CARTESIAN_POINT('Ctrl Pts',(-12.8673180280698,-9.20659637946829,
5.51856857921502));
#12350=CARTESIAN_POINT('Ctrl Pts',(-13.1768087690445,-11.361541563584,5.40742743168602));
#12351=CARTESIAN_POINT('Ctrl Pts',(-15.1551766801017,-12.2701854321462,
5.29628628415699));
#12352=CARTESIAN_POINT('Ctrl Pts',(-16.9915019939467,-11.1007913086607,
5.18514513662797));
#12353=CARTESIAN_POINT('Ctrl Pts',(-17.0048851178101,-8.923776342464,5.07400398909896));
#12354=CARTESIAN_POINT('Ctrl Pts',(-15.1830756697807,-7.73189396271163,
4.96286284156994));
#12355=CARTESIAN_POINT('Ctrl Pts',(-13.1936859915807,-8.61614617822962,
4.85172169404091));
#12356=CARTESIAN_POINT('Ctrl Pts',(-12.8577247426487,-10.7671234703357,
4.7405805465119));
#12357=CARTESIAN_POINT('Ctrl Pts',(-14.4827175676795,-12.215906266585,4.62943939898287));
#12358=CARTESIAN_POINT('Ctrl Pts',(-16.5812102800893,-11.6363360740339,
4.51829825145386));
#12359=CARTESIAN_POINT('Ctrl Pts',(-17.2323256165297,-9.55892853319708,
4.40715710392483));
#12360=CARTESIAN_POINT('Ctrl Pts',(-15.8400583404068,-7.88526037494785,
4.29601595639582));
#12361=CARTESIAN_POINT('Ctrl Pts',(-13.6788348718617,-8.1473412615274,4.1848748088668));
#12362=CARTESIAN_POINT('Ctrl Pts',(-12.7269537282801,-10.1052727109369,
4.07373366133778));
#12363=CARTESIAN_POINT('Ctrl Pts',(-13.8557292751018,-11.9668416827977,
3.96259251380875));
#12364=CARTESIAN_POINT('Ctrl Pts',(-16.0319250038243,-12.0280415389064,
3.85145136627974));
#12365=CARTESIAN_POINT('Ctrl Pts',(-17.2635373820377,-10.2328523505688,
3.74031021875071));
#12366=CARTESIAN_POINT('Ctrl Pts',(-16.4231971315216,-8.22451932652546,
3.6291690712217));
#12367=CARTESIAN_POINT('Ctrl Pts',(-14.2801184940623,-7.84139111591484,
3.51802792369268));
#12368=CARTESIAN_POINT('Ctrl Pts',(-12.795990926042,-9.43416813543636,3.40688677616365));
#12369=CARTESIAN_POINT('Ctrl Pts',(-13.3293261270302,-11.5448852731689,
3.29574562863464));
#12370=CARTESIAN_POINT('Ctrl Pts',(-15.391930139899,-12.2414755101134,3.18460448110562));
#12371=CARTESIAN_POINT('Ctrl Pts',(-17.0957767979589,-10.8863076836954,
3.0734633335766));
#12372=CARTESIAN_POINT('Ctrl Pts',(-16.8812322334449,-8.71984884443381,
2.96232218604758));
#12373=CARTESIAN_POINT('Ctrl Pts',(-14.9446820583973,-7.72518976132214,
2.85118103851856));
#12374=CARTESIAN_POINT('Ctrl Pts',(-13.0587677402097,-8.81280203391929,
2.74003989098954));
#12375=CARTESIAN_POINT('Ctrl Pts',(-12.9497806841384,-10.9871283884299,
2.62889874346052));
#12376=CARTESIAN_POINT('Ctrl Pts',(-14.7174833333107,-12.2578764419345,
2.5177575959315));
#12377=CARTESIAN_POINT('Ctrl Pts',(-16.7437905685052,-11.4618536697156,
2.40661644840248));
#12378=CARTESIAN_POINT('Ctrl Pts',(-17.1739008616738,-9.32770783945607,
2.29547530087346));
#12379=CARTESIAN_POINT('Ctrl Pts',(-15.6141082487193,-7.80895168178116,
2.18433415334444));
#12380=CARTESIAN_POINT('Ctrl Pts',(-13.4921852324529,-8.2957945133747,2.07319300581542));
#12381=CARTESIAN_POINT('Ctrl Pts',(-12.7504562256358,-10.3425997019803,
1.9620518582864));
#12382=CARTESIAN_POINT('Ctrl Pts',(-14.0678706835062,-12.0758026069051,
1.85091071075738));
#12383=CARTESIAN_POINT('Ctrl Pts',(-16.2385194047865,-11.9088979931037,
1.73976956322836));
#12384=CARTESIAN_POINT('Ctrl Pts',(-17.2754765459017,-9.99466339541431,
1.62862841569934));
#12385=CARTESIAN_POINT('Ctrl Pts',(-16.2295521927304,-8.08531416197898,
1.51748726817032));
#12386=CARTESIAN_POINT('Ctrl Pts',(-14.0581448136139,-7.92859177884296,
1.4063461206413));
#12387=CARTESIAN_POINT('Ctrl Pts',(-12.7488735824113,-9.66795626731204,
1.29520497311228));
#12388=CARTESIAN_POINT('Ctrl Pts',(-13.5001961264723,-11.7112572033738,
1.18406382558326));
#12389=CARTESIAN_POINT('Ctrl Pts',(-15.6243766370739,-12.1881472655394,
1.07292267805424));
#12390=CARTESIAN_POINT('Ctrl Pts',(-17.1770336680885,-10.6620815928193,
0.961781530525219));
#12391=CARTESIAN_POINT('Ctrl Pts',(-16.7369081161809,-8.52999632629676,
0.850640382996202));
#12392=CARTESIAN_POINT('Ctrl Pts',(-14.7069088692726,-7.74344832960141,
0.73949923546718));
#12393=CARTESIAN_POINT('Ctrl Pts',(-12.9451484476459,-9.02254762789837,
0.628358087938162));
#12394=CARTESIAN_POINT('Ctrl Pts',(-13.0644055219694,-11.1961954655539,
0.517216940409141));
#12395=CARTESIAN_POINT('Ctrl Pts',(-14.9552594030341,-12.2752280488692,
0.406075792880122));
#12396=CARTESIAN_POINT('Ctrl Pts',(-16.8873964310158,-11.270957778128,0.294934645351101));
#12397=CARTESIAN_POINT('Ctrl Pts',(-17.0912453973186,-9.10456268512506,
0.183793497822081));
#12398=CARTESIAN_POINT('Ctrl Pts',(-15.3821072277069,-7.75535735002619,
0.0726523502930616));
#12399=CARTESIAN_POINT('Ctrl Pts',(-13.3206117613179,-8.46573857410703,
-0.038488797235959));
#12400=CARTESIAN_POINT('Ctrl Pts',(-12.9754720329252,-9.86814094278172,
-0.112582895588638));
#12401=CARTESIAN_POINT('Ctrl Pts',(-13.1375693587171,-10.4874615891075,
-0.149629944764978));
#12402=CARTESIAN_POINT('Ctrl Pts',(-15.4632995769868,-11.7347832743338,
8.14962994476498));
#12403=CARTESIAN_POINT('Ctrl Pts',(-16.0401731930456,-11.5807206278643,
8.11258289558864));
#12404=CARTESIAN_POINT('Ctrl Pts',(-17.01815158292,-10.6544032047635,8.03848879723596));
#12405=CARTESIAN_POINT('Ctrl Pts',(-16.6438328579804,-8.65545565052525,
7.92734764970694));
#12406=CARTESIAN_POINT('Ctrl Pts',(-14.7620123057747,-7.89162435349761,
7.81620650217792));
#12407=CARTESIAN_POINT('Ctrl Pts',(-13.099450286363,-9.05556505728998,7.7050653546489));
#12408=CARTESIAN_POINT('Ctrl Pts',(-13.1758499960607,-11.085103759992,7.59392420711988));
#12409=CARTESIAN_POINT('Ctrl Pts',(-14.9223789228056,-12.1208151249496,
7.48278305959086));
#12410=CARTESIAN_POINT('Ctrl Pts',(-16.7397659688587,-11.2155082179753,
7.37164191206185));
#12411=CARTESIAN_POINT('Ctrl Pts',(-16.9647396778862,-9.19742247827372,
7.26050076453281));
#12412=CARTESIAN_POINT('Ctrl Pts',(-15.3912169517229,-7.91406220448686,
7.1493596170038));
#12413=CARTESIAN_POINT('Ctrl Pts',(-13.4596162201455,-8.54004681423119,
7.03821846947478));
#12414=CARTESIAN_POINT('Ctrl Pts',(-12.9380082150486,-10.5024355415475,
6.92707732194577));
#12415=CARTESIAN_POINT('Ctrl Pts',(-14.3038730281136,-12.0049039626946,
6.81593617441673));
#12416=CARTESIAN_POINT('Ctrl Pts',(-16.3069413064063,-11.6721680698467,
6.70479502688773));
#12417=CARTESIAN_POINT('Ctrl Pts',(-17.1136890633015,-9.80879279462856,
6.59365387935869));
#12418=CARTESIAN_POINT('Ctrl Pts',(-15.9856484483585,-8.1204425018405,6.48251273182969));
#12419=CARTESIAN_POINT('Ctrl Pts',(-13.9553847125051,-8.15256407658869,
6.37137158430066));
#12420=CARTESIAN_POINT('Ctrl Pts',(-12.8813202529855,-9.87575584602892,
6.26023043677165));
#12421=CARTESIAN_POINT('Ctrl Pts',(-13.746611603337,-11.7126756005614,6.14908928924262));
#12422=CARTESIAN_POINT('Ctrl Pts',(-15.7592050695559,-11.9818799262481,
6.0379481417136));
#12423=CARTESIAN_POINT('Ctrl Pts',(-17.0768522663421,-10.4369496690781,
5.92680699418459));
#12424=CARTESIAN_POINT('Ctrl Pts',(-16.493430990268,-8.49205298764794,5.81566584665555));
#12425=CARTESIAN_POINT('Ctrl Pts',(-14.542982039145,-7.92747136914842,5.70452469912656));
#12426=CARTESIAN_POINT('Ctrl Pts',(-13.0108692559441,-9.26000052759082,
5.59338355159751));
#12427=CARTESIAN_POINT('Ctrl Pts',(-13.2995281164661,-11.2698959427991,
5.48224240406851));
#12428=CARTESIAN_POINT('Ctrl Pts',(-15.1447317083435,-12.117378820295,5.37110125653948));
#12429=CARTESIAN_POINT('Ctrl Pts',(-16.8574536171574,-11.0266968369714,
5.25996010901046));
#12430=CARTESIAN_POINT('Ctrl Pts',(-16.8699359204162,-8.99621716089825,
5.14881896148145));
#12431=CARTESIAN_POINT('Ctrl Pts',(-15.1707528117377,-7.88456061010077,
5.03767781395242));
#12432=CARTESIAN_POINT('Ctrl Pts',(-13.3152693299537,-8.7092936413433,4.9265366664234));
#12433=CARTESIAN_POINT('Ctrl Pts',(-13.0019216963835,-10.7154882441055,
4.81539551889438));
#12434=CARTESIAN_POINT('Ctrl Pts',(-14.5175359462726,-12.0667531956587,
4.70425437136536));
#12435=CARTESIAN_POINT('Ctrl Pts',(-16.4747787163486,-11.5261939826513,
4.59311322383635));
#12436=CARTESIAN_POINT('Ctrl Pts',(-17.0820673560456,-9.58861713725206,
4.48197207630732));
#12437=CARTESIAN_POINT('Ctrl Pts',(-15.7835138542441,-8.02760390005202,
4.37083092877831));
#12438=CARTESIAN_POINT('Ctrl Pts',(-13.7677627471216,-8.27204407246692,
4.25968978124928));
#12439=CARTESIAN_POINT('Ctrl Pts',(-12.8799529037855,-10.0981867848047,
4.14854863372027));
#12440=CARTESIAN_POINT('Ctrl Pts',(-13.9327503545415,-11.8344531962273,
4.03740748619124));
#12441=CARTESIAN_POINT('Ctrl Pts',(-15.9624659361701,-11.8915336784182,
3.92626633866223));
#12442=CARTESIAN_POINT('Ctrl Pts',(-17.1111782516997,-10.2171790147046,
3.81512519113321));
#12443=CARTESIAN_POINT('Ctrl Pts',(-16.3274014627693,-8.34402726727746,
3.70398404360418));
#12444=CARTESIAN_POINT('Ctrl Pts',(-14.3285738547121,-7.98668748916186,
3.59284289607517));
#12445=CARTESIAN_POINT('Ctrl Pts',(-12.9443431946769,-9.47225438551843,
3.48170174854614));
#12446=CARTESIAN_POINT('Ctrl Pts',(-13.4417795021695,-11.440898752531,3.37056060101713));
#12447=CARTESIAN_POINT('Ctrl Pts',(-15.3655492478748,-12.0906013685574,
3.2594194534881));
#12448=CARTESIAN_POINT('Ctrl Pts',(-16.9547096643416,-10.8266501454673,
3.14827830595909));
#12449=CARTESIAN_POINT('Ctrl Pts',(-16.7546061351414,-8.80601606142392,
3.03713715843006));
#12450=CARTESIAN_POINT('Ctrl Pts',(-14.9484055195346,-7.87830766977787,
2.92599601090105));
#12451=CARTESIAN_POINT('Ctrl Pts',(-13.1894324516621,-8.89271255410176,
2.81485486337202));
#12452=CARTESIAN_POINT('Ctrl Pts',(-13.0877813349982,-10.9206845894511,
2.70371371584301));
#12453=CARTESIAN_POINT('Ctrl Pts',(-14.736499583709,-12.1058983505481,2.59257256831398));
#12454=CARTESIAN_POINT('Ctrl Pts',(-16.6264156947269,-11.3634560220484,
2.48143142078497));
#12455=CARTESIAN_POINT('Ctrl Pts',(-17.027575182516,-9.37295995224483,2.37029027325595));
#12456=CARTESIAN_POINT('Ctrl Pts',(-15.5727725060668,-7.95643155949003,
2.25914912572693));
#12457=CARTESIAN_POINT('Ctrl Pts',(-13.5936765303291,-8.41050490778654,
2.14800797819791));
#12458=CARTESIAN_POINT('Ctrl Pts',(-12.9018734435882,-10.3195392510852,
2.03686683066889));
#12459=CARTESIAN_POINT('Ctrl Pts',(-14.1306124845255,-11.9360799398746,
1.92572568313987));
#12460=CARTESIAN_POINT('Ctrl Pts',(-16.1551544288345,-11.7804097072723,
1.81458453561085));
#12461=CARTESIAN_POINT('Ctrl Pts',(-17.1223137881804,-9.99502260328078,
1.70344338808183));
#12462=CARTESIAN_POINT('Ctrl Pts',(-16.1467908015221,-8.21419202874906,
1.59230224055281));
#12463=CARTESIAN_POINT('Ctrl Pts',(-14.1215412647796,-8.06801865893557,
1.48116109302379));
#12464=CARTESIAN_POINT('Ctrl Pts',(-12.9003973283792,-9.69030619391275,
1.37001994549477));
#12465=CARTESIAN_POINT('Ctrl Pts',(-13.6011482095532,-11.5960721565707,
1.25887879796575));
#12466=CARTESIAN_POINT('Ctrl Pts',(-15.5823497272544,-12.0408626582364,
1.14773765043673));
#12467=CARTESIAN_POINT('Ctrl Pts',(-17.030497119137,-10.61751675528,1.03659650290771));
#12468=CARTESIAN_POINT('Ctrl Pts',(-16.6199965015735,-8.62894255227754,
0.92545535537869));
#12469=CARTESIAN_POINT('Ctrl Pts',(-14.7266368888501,-7.89533725036455,
0.814314207849669));
#12470=CARTESIAN_POINT('Ctrl Pts',(-13.0834608952223,-9.0883401323836,0.703173060320652));
#12471=CARTESIAN_POINT('Ctrl Pts',(-13.1946907532627,-11.115679321976,0.59203191279163));
#12472=CARTESIAN_POINT('Ctrl Pts',(-14.9582709010984,-12.1220820175303,
0.480890765262611));
#12473=CARTESIAN_POINT('Ctrl Pts',(-16.7603554194051,-11.1854093691163,
0.369749617733591));
#12474=CARTESIAN_POINT('Ctrl Pts',(-16.9504832731376,-9.1648347405588,0.258608470204569));
#12475=CARTESIAN_POINT('Ctrl Pts',(-15.3563875177647,-7.90644467236664,
0.147467322675551));
#12476=CARTESIAN_POINT('Ctrl Pts',(-13.4336517020655,-8.56901000157061,
0.0363261751465299));
#12477=CARTESIAN_POINT('Ctrl Pts',(-13.1117433942273,-9.87701640092276,
-0.0377679232061492));
#12478=CARTESIAN_POINT('Ctrl Pts',(-13.2629299182875,-10.4546504571249,
-0.0748149723824891));
#12479=CARTESIAN_POINT('Ctrl Pts',(-15.4298642568859,-11.6095877486648,
8.22444491714747));
#12480=CARTESIAN_POINT('Ctrl Pts',(-15.9651061621278,-11.4666434674091,
8.18739786797113));
#12481=CARTESIAN_POINT('Ctrl Pts',(-16.872505984394,-10.6071763526074,8.11330376961845));
#12482=CARTESIAN_POINT('Ctrl Pts',(-16.5252010255137,-8.75248848402567,
8.00216262208943));
#12483=CARTESIAN_POINT('Ctrl Pts',(-14.7791873586601,-8.04378122593049,
7.89102147456041));
#12484=CARTESIAN_POINT('Ctrl Pts',(-13.2366088144507,-9.12372286746838,
7.7798803270314));
#12485=CARTESIAN_POINT('Ctrl Pts',(-13.3074949237131,-11.0067941880429,
7.66873917950236));
#12486=CARTESIAN_POINT('Ctrl Pts',(-14.9279806666696,-11.9677605224854,
7.55759803197335));
#12487=CARTESIAN_POINT('Ctrl Pts',(-16.6142108529922,-11.1277876406814,
7.44645688444433));
#12488=CARTESIAN_POINT('Ctrl Pts',(-16.822948700065,-9.25534274774437,7.3353157369153));
#12489=CARTESIAN_POINT('Ctrl Pts',(-15.3629836774885,-8.06459978614663,
7.22417458938629));
#12490=CARTESIAN_POINT('Ctrl Pts',(-13.570782358247,-8.64540845176172,7.11303344185727));
#12491=CARTESIAN_POINT('Ctrl Pts',(-13.0868176653479,-10.4661758642325,
7.00189229432825));
#12492=CARTESIAN_POINT('Ctrl Pts',(-14.3541109935512,-11.8602144160296,
6.89075114679923));
#12493=CARTESIAN_POINT('Ctrl Pts',(-16.2126222025189,-11.5514913469335,
6.77960999927021));
#12494=CARTESIAN_POINT('Ctrl Pts',(-16.9611487331658,-9.82259180165284,
6.66846885174119));
#12495=CARTESIAN_POINT('Ctrl Pts',(-15.9145163493564,-8.25608606751732,
6.55732770421217));
#12496=CARTESIAN_POINT('Ctrl Pts',(-14.0307723196919,-8.28588949826707,
6.44618655668315));
#12497=CARTESIAN_POINT('Ctrl Pts',(-13.034220749881,-9.88472227566764,6.33504540915413));
#12498=CARTESIAN_POINT('Ctrl Pts',(-13.8370659105171,-11.5890755374958,
6.22390426162511));
#12499=CARTESIAN_POINT('Ctrl Pts',(-15.7044148953711,-11.8388519740824,
6.11276311409609));
#12500=CARTESIAN_POINT('Ctrl Pts',(-16.9269703675087,-10.4054159643667,
6.00162196656707));
#12501=CARTESIAN_POINT('Ctrl Pts',(-16.3856533325956,-8.60087823497738,
5.89048081903805));
#12502=CARTESIAN_POINT('Ctrl Pts',(-14.5759640287087,-8.07704124063746,
5.77933967150903));
#12503=CARTESIAN_POINT('Ctrl Pts',(-13.1544204838184,-9.31340467571335,
5.66819852398002));
#12504=CARTESIAN_POINT('Ctrl Pts',(-13.4222474638878,-11.1782503220142,
5.55705737645098));
#12505=CARTESIAN_POINT('Ctrl Pts',(-15.1342867365853,-11.9645722084437,
5.44591622892198));
#12506=CARTESIAN_POINT('Ctrl Pts',(-16.723405240368,-10.952602365282,5.33477508139295));
#12507=CARTESIAN_POINT('Ctrl Pts',(-16.7349867230223,-9.06865797933251,
5.22363393386394));
#12508=CARTESIAN_POINT('Ctrl Pts',(-15.1584299536947,-8.0372272574899,5.11249278633491));
#12509=CARTESIAN_POINT('Ctrl Pts',(-13.4368526683266,-8.80244110445702,
5.00135163880589));
#12510=CARTESIAN_POINT('Ctrl Pts',(-13.1461186501183,-10.6638530178752,
4.89021049127687));
#12511=CARTESIAN_POINT('Ctrl Pts',(-14.5523543248657,-11.9176001247324,
4.77906934374785));
#12512=CARTESIAN_POINT('Ctrl Pts',(-16.3683471526078,-11.4160518912686,
4.66792819621883));
#12513=CARTESIAN_POINT('Ctrl Pts',(-16.9318090955615,-9.61830574130706,
4.55678704868981));
#12514=CARTESIAN_POINT('Ctrl Pts',(-15.7269693680813,-8.16994742515617,
4.44564590116079));
#12515=CARTESIAN_POINT('Ctrl Pts',(-13.8566906223815,-8.39674688340643,
4.33450475363178));
#12516=CARTESIAN_POINT('Ctrl Pts',(-13.0329520792908,-10.0911008586724,
4.22336360610275));
#12517=CARTESIAN_POINT('Ctrl Pts',(-14.0097714339813,-11.7020647096568,
4.11222245857374));
#12518=CARTESIAN_POINT('Ctrl Pts',(-15.8930068685159,-11.7550258179299,
4.00108131104471));
#12519=CARTESIAN_POINT('Ctrl Pts',(-16.9588191213617,-10.2015056788404,
3.88994016351569));
#12520=CARTESIAN_POINT('Ctrl Pts',(-16.2316057940169,-8.46353520802948,
3.77879901598668));
#12521=CARTESIAN_POINT('Ctrl Pts',(-14.377029215362,-8.13198386240885,3.66765786845765));
#12522=CARTESIAN_POINT('Ctrl Pts',(-13.0926954633119,-9.51034063560054,
3.55651672092863));
#12523=CARTESIAN_POINT('Ctrl Pts',(-13.5542328773088,-11.336912231893,3.44537557339961));
#12524=CARTESIAN_POINT('Ctrl Pts',(-15.3391683558506,-11.9397272270015,
3.3342344258706));
#12525=CARTESIAN_POINT('Ctrl Pts',(-16.8136425307244,-10.7669926072391,
3.22309327834158));
#12526=CARTESIAN_POINT('Ctrl Pts',(-16.627980036838,-8.89218327841403,3.11195213081255));
#12527=CARTESIAN_POINT('Ctrl Pts',(-14.9521289806718,-8.03142557823359,
3.00081098328354));
#12528=CARTESIAN_POINT('Ctrl Pts',(-13.3200971631145,-8.97262307428424,
2.88966983575451));
#12529=CARTESIAN_POINT('Ctrl Pts',(-13.2257819858581,-10.8542407904722,
2.7785286882255));
#12530=CARTESIAN_POINT('Ctrl Pts',(-14.7555158341074,-11.9539202591618,
2.66738754069647));
#12531=CARTESIAN_POINT('Ctrl Pts',(-16.5090408209486,-11.2650583743812,
2.55624639316746));
#12532=CARTESIAN_POINT('Ctrl Pts',(-16.8812495033582,-9.41821206503357,
2.44510524563843));
#12533=CARTESIAN_POINT('Ctrl Pts',(-15.5314367634142,-8.1039114371989,2.33396409810942));
#12534=CARTESIAN_POINT('Ctrl Pts',(-13.6951678282053,-8.52521530219838,
2.2228229505804));
#12535=CARTESIAN_POINT('Ctrl Pts',(-13.0532906615406,-10.29647880019,2.11168180305138));
#12536=CARTESIAN_POINT('Ctrl Pts',(-14.1933542855448,-11.7963572728442,
2.00054065552236));
#12537=CARTESIAN_POINT('Ctrl Pts',(-16.0717894528825,-11.651921421441,1.88939950799334));
#12538=CARTESIAN_POINT('Ctrl Pts',(-16.9691510304591,-9.99538181114722,
1.77825836046432));
#12539=CARTESIAN_POINT('Ctrl Pts',(-16.0640294103137,-8.34306989551916,
1.6671172129353));
#12540=CARTESIAN_POINT('Ctrl Pts',(-14.1849377159453,-8.20744553902816,
1.55597606540628));
#12541=CARTESIAN_POINT('Ctrl Pts',(-13.0519210743471,-9.71265612051347,
1.44483491787726));
#12542=CARTESIAN_POINT('Ctrl Pts',(-13.7021002926342,-11.4808871097675,
1.33369377034824));
#12543=CARTESIAN_POINT('Ctrl Pts',(-15.5403228174349,-11.8935780509334,
1.22255262281922));
#12544=CARTESIAN_POINT('Ctrl Pts',(-16.8839605701855,-10.5729519177407,
1.1114114752902));
#12545=CARTESIAN_POINT('Ctrl Pts',(-16.503084886966,-8.72788877825835,1.00027032776118));
#12546=CARTESIAN_POINT('Ctrl Pts',(-14.7463649084277,-8.04722617112768,
0.889129180232157));
#12547=CARTESIAN_POINT('Ctrl Pts',(-13.2217733427987,-9.15413263686884,
0.777988032703141));
#12548=CARTESIAN_POINT('Ctrl Pts',(-13.324975984556,-11.0351631783981,0.666846885174119));
#12549=CARTESIAN_POINT('Ctrl Pts',(-14.9612823991627,-11.9689359861914,
0.5557057376451));
#12550=CARTESIAN_POINT('Ctrl Pts',(-16.6333144077944,-11.0998609601046,
0.444564590116079));
#12551=CARTESIAN_POINT('Ctrl Pts',(-16.8097211489565,-9.22510679599255,
0.333423442587059));
#12552=CARTESIAN_POINT('Ctrl Pts',(-15.3306678078225,-8.0575319947071,0.22228229505804));
#12553=CARTESIAN_POINT('Ctrl Pts',(-13.5466916428131,-8.67228142903419,
0.111141147529019));
#12554=CARTESIAN_POINT('Ctrl Pts',(-13.2480147555294,-9.88589185906381,
0.0370470491763399));
#12555=CARTESIAN_POINT('Ctrl Pts',(-13.3882904778579,-10.4218393251423,
0.));
#12556=CARTESIAN_POINT('Ctrl Pts',(-13.3882904778579,-10.4218393251423,
0.));
#12557=CARTESIAN_POINT('Ctrl Pts',(-13.3657944025764,-10.364062743702,-3.7859623319602E-17));
#12558=CARTESIAN_POINT('Ctrl Pts',(-13.3468720776219,-10.3051562840246,
1.43829901930131E-15));
#12559=CARTESIAN_POINT('Ctrl Pts',(-13.3313727935116,-10.2454301582812,
1.2490009027033E-15));
#12560=CARTESIAN_POINT('Ctrl Pts',(-13.3148521018426,-10.1817680626023,
1.04722798238191E-15));
#12561=CARTESIAN_POINT('Ctrl Pts',(-13.3022199241254,-10.1171741832588,
-2.07892182731082E-15));
#12562=CARTESIAN_POINT('Ctrl Pts',(-13.2933434453493,-10.0519874094327,
-1.55431223447522E-15));
#12563=CARTESIAN_POINT('Ctrl Pts',(-13.2855765264201,-9.99494898233489,
-1.09527884074407E-15));
#12564=CARTESIAN_POINT('Ctrl Pts',(-13.2806858148038,-9.93745562189104,
1.18024020512711E-16));
#12565=CARTESIAN_POINT('Ctrl Pts',(-13.2786149095285,-9.87971946880946,
-1.38777878078145E-16));
#12566=CARTESIAN_POINT('Ctrl Pts',(-13.2775754853061,-9.85074066579963,
-2.67671322386771E-16));
#12567=CARTESIAN_POINT('Ctrl Pts',(-13.2772469104407,-9.82170053398399,
1.4948294717503E-15));
#12568=CARTESIAN_POINT('Ctrl Pts',(-13.2776249668018,-9.79262525364946,
1.63757896132211E-15));
#12569=CARTESIAN_POINT('Ctrl Pts',(-13.2777973926671,-9.77936445211961,
1.70268487355815E-15));
#12570=CARTESIAN_POINT('Ctrl Pts',(-13.2781170152694,-9.76609462368694,
-4.7430123169196E-16));
#12571=CARTESIAN_POINT('Ctrl Pts',(-13.2785824498934,-9.75283980605701,
-5.27355936696949E-16));
#12572=CARTESIAN_POINT('Ctrl Pts',(-13.280933076777,-9.68589779304374,-7.95302946759129E-16));
#12573=CARTESIAN_POINT('Ctrl Pts',(-13.2869992525162,-9.61921855261629,
1.59603393177068E-15));
#12574=CARTESIAN_POINT('Ctrl Pts',(-13.2966473181584,-9.55313456281087,
1.49880108324396E-15));
#12575=CARTESIAN_POINT('Ctrl Pts',(-13.3064659127467,-9.4858825426913,1.39984965030756E-15));
#12576=CARTESIAN_POINT('Ctrl Pts',(-13.3199939979885,-9.41924600106486,
3.7367831032364E-16));
#12577=CARTESIAN_POINT('Ctrl Pts',(-13.3371419608068,-9.35355952774662,
2.4980018054066E-16));
#12578=CARTESIAN_POINT('Ctrl Pts',(-13.3514852540965,-9.29861653761111,
1.46183187287034E-16));
#12579=CARTESIAN_POINT('Ctrl Pts',(-13.3683620550236,-9.24433764320676,
4.21405766872162E-17));
#12580=CARTESIAN_POINT('Ctrl Pts',(-13.3877476280939,-9.19091835353792,
-2.77555756156289E-16));
#12581=CARTESIAN_POINT('Ctrl Pts',(-13.39668378758,-9.16629368598843,-4.24926040595927E-16));
#12582=CARTESIAN_POINT('Ctrl Pts',(-13.4061533950394,-9.14185172195395,
7.07869180218989E-16));
#12583=CARTESIAN_POINT('Ctrl Pts',(-13.4161558307215,-9.11761203383739,
6.93889390390723E-16));
#12584=CARTESIAN_POINT('Ctrl Pts',(-13.4205143377574,-9.10704972136054,
6.87797772882415E-16));
#12585=CARTESIAN_POINT('Ctrl Pts',(-13.4249739997542,-9.09652612469906,
-3.22868594808326E-17));
#12586=CARTESIAN_POINT('Ctrl Pts',(-13.4295289897423,-9.08605561214841,
-5.55111512312578E-17));
#12587=CARTESIAN_POINT('Ctrl Pts',(-13.4575216444335,-9.02170916066706,
-1.98235851199708E-16));
#12588=CARTESIAN_POINT('Ctrl Pts',(-13.489160585127,-8.95924403457073,-2.25359481219569E-15));
#12589=CARTESIAN_POINT('Ctrl Pts',(-13.524338957658,-8.8990088207193,-1.98452365651747E-15));
#12590=CARTESIAN_POINT('Ctrl Pts',(-13.5557936925823,-8.84514951602471,
-1.74393373524742E-15));
#12591=CARTESIAN_POINT('Ctrl Pts',(-13.590078948554,-8.79307231810761,5.85737278460583E-16));
#12592=CARTESIAN_POINT('Ctrl Pts',(-13.627153472105,-8.74302986930091,1.12410081243297E-15));
#12593=CARTESIAN_POINT('Ctrl Pts',(-13.6675383362097,-8.68851918916382,
1.70977456371544E-15));
#12594=CARTESIAN_POINT('Ctrl Pts',(-13.7112321890346,-8.63642161961057,
1.4217873119626E-15));
#12595=CARTESIAN_POINT('Ctrl Pts',(-13.7579211246953,-8.58682326989449,
1.22124532708767E-15));
#12596=CARTESIAN_POINT('Ctrl Pts',(-13.7759302268488,-8.56769193322904,
1.14389121651416E-15));
#12597=CARTESIAN_POINT('Ctrl Pts',(-13.7943854276088,-8.54893272295167,
2.44014659021857E-15));
#12598=CARTESIAN_POINT('Ctrl Pts',(-13.8132703795349,-8.53055173814469,
2.44249065417534E-15));
#12599=CARTESIAN_POINT('Ctrl Pts',(-13.8215560161117,-8.52248721350985,
2.44351909534558E-15));
#12600=CARTESIAN_POINT('Ctrl Pts',(-13.8299240193705,-8.5144959821821,-9.50368270547519E-16));
#12601=CARTESIAN_POINT('Ctrl Pts',(-13.838363019459,-8.50658761589045,-9.57567358739198E-16));
#12602=CARTESIAN_POINT('Ctrl Pts',(-13.8893887557786,-8.45877031420949,
-1.00109606734903E-15));
#12603=CARTESIAN_POINT('Ctrl Pts',(-13.9430963123383,-8.4138917808739,-6.40189758604347E-17));
#12604=CARTESIAN_POINT('Ctrl Pts',(-13.9991087396997,-8.37201357687976,
3.19189119579733E-16));
#12605=CARTESIAN_POINT('Ctrl Pts',(-14.0564211033334,-8.32916346363337,
7.11290707528551E-16));
#12606=CARTESIAN_POINT('Ctrl Pts',(-14.1161471900346,-8.28945395175835,
1.00414780997289E-15));
#12607=CARTESIAN_POINT('Ctrl Pts',(-14.1779321771154,-8.25297867940102,
2.02615701994091E-15));
#12608=CARTESIAN_POINT('Ctrl Pts',(-14.2252015423102,-8.22507282312259,
2.80805775118726E-15));
#12609=CARTESIAN_POINT('Ctrl Pts',(-14.2736771332203,-8.19906053178973,
2.53848381353579E-15));
#12610=CARTESIAN_POINT('Ctrl Pts',(-14.3232149985245,-8.17499768689248,
2.74780198594726E-15));
#12611=CARTESIAN_POINT('Ctrl Pts',(-14.3540407103556,-8.16002420513092,
2.8780534940441E-15));
#12612=CARTESIAN_POINT('Ctrl Pts',(-14.3852779880121,-8.1458058278048,1.08257402890549E-15));
#12613=CARTESIAN_POINT('Ctrl Pts',(-14.4168940263936,-8.13235879193744,
1.13103970633688E-15));
#12614=CARTESIAN_POINT('Ctrl Pts',(-14.4346636982448,-8.12480093753923,
1.15827965251909E-15));
#12615=CARTESIAN_POINT('Ctrl Pts',(-14.4525590851067,-8.11748457270256,
1.14587934816188E-15));
#12616=CARTESIAN_POINT('Ctrl Pts',(-14.470541741264,-8.11042529656637,1.04777297948999E-15));
#12617=CARTESIAN_POINT('Ctrl Pts',(-14.5401796653021,-8.08308821515669,
6.67855586339259E-16));
#12618=CARTESIAN_POINT('Ctrl Pts',(-14.611192923579,-8.05957098628127,1.41062069047362E-15));
#12619=CARTESIAN_POINT('Ctrl Pts',(-14.683209836623,-8.03998786369269,1.49880108324396E-15));
#12620=CARTESIAN_POINT('Ctrl Pts',(-14.7370845758773,-8.02533803244261,
1.56476747179147E-15));
#12621=CARTESIAN_POINT('Ctrl Pts',(-14.7915219476125,-8.01289052704023,
-7.21547261836267E-16));
#12622=CARTESIAN_POINT('Ctrl Pts',(-14.8463769008119,-8.00270909147673,
-6.76542155630955E-16));
#12623=CARTESIAN_POINT('Ctrl Pts',(-14.8634609622712,-7.99953817871924,
-6.62525736774458E-16));
#12624=CARTESIAN_POINT('Ctrl Pts',(-14.8805855769004,-7.99658717289818,
-1.00648135721956E-15));
#12625=CARTESIAN_POINT('Ctrl Pts',(-14.8977464806917,-7.99385830531565,
-1.14491749414469E-15));
#12626=CARTESIAN_POINT('Ctrl Pts',(-14.9143450340983,-7.9912188607468,-1.27881717915669E-15));
#12627=CARTESIAN_POINT('Ctrl Pts',(-14.9309690935528,-7.98878863041095,
-2.06502921266531E-15));
#12628=CARTESIAN_POINT('Ctrl Pts',(-14.9476086519096,-7.98656978706703,
-2.17534323887492E-15));
#12629=CARTESIAN_POINT('Ctrl Pts',(-15.0222846677452,-7.9766119277817,-2.67041719405268E-15));
#12630=CARTESIAN_POINT('Ctrl Pts',(-15.0973087342006,-7.97090191711569,
-8.83830117641646E-17));
#12631=CARTESIAN_POINT('Ctrl Pts',(-15.1723238725507,-7.96957800273067,
4.04190569902596E-16));
#12632=CARTESIAN_POINT('Ctrl Pts',(-15.2297781588663,-7.96856401331724,
7.81453935871769E-16));
#12633=CARTESIAN_POINT('Ctrl Pts',(-15.28722791073,-7.97012372441746,1.62407242976159E-15));
#12634=CARTESIAN_POINT('Ctrl Pts',(-15.3445186506179,-7.9743391343232,1.55257751099924E-15));
#12635=CARTESIAN_POINT('Ctrl Pts',(-15.3577644165905,-7.97531374790297,
1.53951714939913E-15));
#12636=CARTESIAN_POINT('Ctrl Pts',(-15.3710016931801,-7.97643039983451,
9.09140411173112E-16));
#12637=CARTESIAN_POINT('Ctrl Pts',(-15.3842290239278,-7.97768774796568,
9.0205620750794E-16));
#12638=CARTESIAN_POINT('Ctrl Pts',(-16.6638186297495,-9.99906044123799,
7.37851963660979));
#12639=CARTESIAN_POINT('Ctrl Pts',(-16.6649348408491,-9.78304620021843,
7.36411833671163));
#12640=CARTESIAN_POINT('Ctrl Pts',(-16.6258964811017,-9.56741857858544,
7.34971703681347));
#12641=CARTESIAN_POINT('Ctrl Pts',(-16.5448315551234,-9.36895973630092,
7.33531573691531));
#12642=CARTESIAN_POINT('Ctrl Pts',(-16.3362936925395,-8.85842842721179,
7.29826868773897));
#12643=CARTESIAN_POINT('Ctrl Pts',(-15.849638685014,-8.46151410667921,7.26122163856263));
#12644=CARTESIAN_POINT('Ctrl Pts',(-15.3076109613776,-8.3598583906821,7.22417458938629));
#12645=CARTESIAN_POINT('Ctrl Pts',(-14.7655832377413,-8.25820267468499,
7.18712754020995));
#12646=CARTESIAN_POINT('Ctrl Pts',(-14.1681827979942,-8.45180556322336,
7.15008049103361));
#12647=CARTESIAN_POINT('Ctrl Pts',(-13.7888217959707,-8.85206824290433,
7.11303344185727));
#12648=CARTESIAN_POINT('Ctrl Pts',(-13.4094607939473,-9.25233092258531,
7.07598639268093));
#12649=CARTESIAN_POINT('Ctrl Pts',(-13.2481392296476,-9.8592533934089,7.03893934350459));
#12650=CARTESIAN_POINT('Ctrl Pts',(-13.3786940021983,-10.3950543874535,
7.00189229432825));
#12651=CARTESIAN_POINT('Ctrl Pts',(-13.509248774749,-10.9308553814982,6.96484524515191));
#12652=CARTESIAN_POINT('Ctrl Pts',(-13.9316798841501,-11.3955348987639,
6.92779819597557));
#12653=CARTESIAN_POINT('Ctrl Pts',(-14.4526473070119,-11.5764208125474,
6.89075114679923));
#12654=CARTESIAN_POINT('Ctrl Pts',(-14.9736147298738,-11.7573067263309,
6.85370409762289));
#12655=CARTESIAN_POINT('Ctrl Pts',(-15.5931184661963,-11.6543990366322,
6.81665704844655));
#12656=CARTESIAN_POINT('Ctrl Pts',(-16.0276247561321,-11.3147952675694,
6.77960999927021));
#12657=CARTESIAN_POINT('Ctrl Pts',(-16.422837505005,-11.0059027562118,6.74591321171674));
#12658=CARTESIAN_POINT('Ctrl Pts',(-16.6649994941594,-10.5011885431139,
6.71221642416327));
#12659=CARTESIAN_POINT('Ctrl Pts',(-16.6681788248613,-9.99913246376521,
6.6785196366098));
#12660=CARTESIAN_POINT('Ctrl Pts',(-15.5301702171886,-11.9851743256717,
8.));
#12661=CARTESIAN_POINT('Ctrl Pts',(-15.6001784614245,-11.9592528683504,
8.));
#12662=CARTESIAN_POINT('Ctrl Pts',(-15.6685003286655,-11.9292588432449,
8.));
#12663=CARTESIAN_POINT('Ctrl Pts',(-15.7349164951987,-11.895479109407,8.));
#12664=CARTESIAN_POINT('Ctrl Pts',(-15.7995895967044,-11.8625859108175,
8.));
#12665=CARTESIAN_POINT('Ctrl Pts',(-15.8624561372199,-11.8261021803305,
8.));
#12666=CARTESIAN_POINT('Ctrl Pts',(-15.9232826782083,-11.7862589889858,
8.));
#12667=CARTESIAN_POINT('Ctrl Pts',(-15.9368593447254,-11.7773658690899,
8.));
#12668=CARTESIAN_POINT('Ctrl Pts',(-15.9503360255514,-11.7683040401431,
8.));
#12669=CARTESIAN_POINT('Ctrl Pts',(-15.9637041645642,-11.7590798556399,
8.));
#12670=CARTESIAN_POINT('Ctrl Pts',(-16.0250458750272,-11.7167533018461,
8.));
#12671=CARTESIAN_POINT('Ctrl Pts',(-16.0839844344716,-11.6710958663792,
8.));
#12672=CARTESIAN_POINT('Ctrl Pts',(-16.1402812498345,-11.6223768930558,
8.));
#12673=CARTESIAN_POINT('Ctrl Pts',(-16.179806333597,-11.5881720896576,8.));
#12674=CARTESIAN_POINT('Ctrl Pts',(-16.2180285241833,-11.5524573236335,
8.));
#12675=CARTESIAN_POINT('Ctrl Pts',(-16.2548523907682,-11.5153174086833,
8.));
#12676=CARTESIAN_POINT('Ctrl Pts',(-16.2688610567185,-11.5011885104928,
8.));
#12677=CARTESIAN_POINT('Ctrl Pts',(-16.2826672344801,-11.4868533051394,
8.));
#12678=CARTESIAN_POINT('Ctrl Pts',(-16.2962652100924,-11.4723162794782,
8.));
#12679=CARTESIAN_POINT('Ctrl Pts',(-16.3091901141748,-11.4584988063725,
8.));
#12680=CARTESIAN_POINT('Ctrl Pts',(-16.3219307389119,-11.4444944578142,
8.));
#12681=CARTESIAN_POINT('Ctrl Pts',(-16.3344601775897,-11.430332285647,8.));
#12682=CARTESIAN_POINT('Ctrl Pts',(-16.3825592602788,-11.3759653257495,
8.));
#12683=CARTESIAN_POINT('Ctrl Pts',(-16.4276039061328,-11.3192201229115,
8.));
#12684=CARTESIAN_POINT('Ctrl Pts',(-16.4693715627496,-11.2603446276274,
8.));
#12685=CARTESIAN_POINT('Ctrl Pts',(-16.5102413201592,-11.2027348069065,
8.));
#12686=CARTESIAN_POINT('Ctrl Pts',(-16.5479738235429,-11.1430844349936,
8.));
#12687=CARTESIAN_POINT('Ctrl Pts',(-16.5823154377681,-11.0816066782684,
8.));
#12688=CARTESIAN_POINT('Ctrl Pts',(-16.6159042787281,-11.0214765230673,
8.));
#12689=CARTESIAN_POINT('Ctrl Pts',(-16.6462495368313,-10.9595975009557,
8.));
#12690=CARTESIAN_POINT('Ctrl Pts',(-16.6730656532177,-10.8961620666141,
8.));
#12691=CARTESIAN_POINT('Ctrl Pts',(-16.6817772278961,-10.8755542158888,
8.));
#12692=CARTESIAN_POINT('Ctrl Pts',(-16.6901159465972,-10.854782095613,8.));
#12693=CARTESIAN_POINT('Ctrl Pts',(-16.6980708146011,-10.8338523288304,
8.));
#12694=CARTESIAN_POINT('Ctrl Pts',(-16.7025652307942,-10.8220272322104,
8.));
#12695=CARTESIAN_POINT('Ctrl Pts',(-16.7069374588343,-10.810150529649,8.));
#12696=CARTESIAN_POINT('Ctrl Pts',(-16.7111796927613,-10.7982404031086,
8.));
#12697=CARTESIAN_POINT('Ctrl Pts',(-16.7340960329223,-10.7339024821311,
8.));
#12698=CARTESIAN_POINT('Ctrl Pts',(-16.7532665659449,-10.6684789076532,
8.));
#12699=CARTESIAN_POINT('Ctrl Pts',(-16.7684629972282,-10.6021691817607,
8.));
#12700=CARTESIAN_POINT('Ctrl Pts',(-16.7706603748747,-10.5925809102312,
8.));
#12701=CARTESIAN_POINT('Ctrl Pts',(-16.772774571369,-10.582974096752,8.));
#12702=CARTESIAN_POINT('Ctrl Pts',(-16.7748048055191,-10.5733493334729,
8.));
#12703=CARTESIAN_POINT('Ctrl Pts',(-16.7891234309595,-10.5054687984451,
8.));
#12704=CARTESIAN_POINT('Ctrl Pts',(-16.799269982444,-10.4366949085313,8.));
#12705=CARTESIAN_POINT('Ctrl Pts',(-16.805341122567,-10.367383506366,8.));
#12706=CARTESIAN_POINT('Ctrl Pts',(-16.8110051473463,-10.3027199520097,
8.));
#12707=CARTESIAN_POINT('Ctrl Pts',(-16.8131212227444,-10.2375878497544,
8.));
#12708=CARTESIAN_POINT('Ctrl Pts',(-16.8117296898732,-10.1722884874833,
8.));
#12709=CARTESIAN_POINT('Ctrl Pts',(-16.8114208851943,-10.1577974545929,
8.));
#12710=CARTESIAN_POINT('Ctrl Pts',(-16.8109392074865,-10.1432982578336,
8.));
#12711=CARTESIAN_POINT('Ctrl Pts',(-16.8102848748653,-10.1287943297925,
8.));
#12712=CARTESIAN_POINT('Ctrl Pts',(-16.8097776518725,-10.117551231788,8.));
#12713=CARTESIAN_POINT('Ctrl Pts',(-16.8091666413548,-10.1063061788777,
8.));
#12714=CARTESIAN_POINT('Ctrl Pts',(-16.8084530036145,-10.0950735021604,
8.));
#12715=CARTESIAN_POINT('Ctrl Pts',(-16.8041172567116,-10.0268287323881,
8.));
#12716=CARTESIAN_POINT('Ctrl Pts',(-16.7959924597437,-9.95891461918857,
8.));
#12717=CARTESIAN_POINT('Ctrl Pts',(-16.7841888730333,-9.89166697312925,
8.));
#12718=CARTESIAN_POINT('Ctrl Pts',(-16.7724402253421,-9.82473232682209,
8.));
#12719=CARTESIAN_POINT('Ctrl Pts',(-16.757046467,-9.75845693091033,8.));
#12720=CARTESIAN_POINT('Ctrl Pts',(-16.7380691925747,-9.69319173096208,
8.));
#12721=CARTESIAN_POINT('Ctrl Pts',(-16.7194993974145,-9.6293279027342,8.));
#12722=CARTESIAN_POINT('Ctrl Pts',(-16.6974977885672,-9.56643054222536,
8.));
#12723=CARTESIAN_POINT('Ctrl Pts',(-16.6720845431421,-9.50486087342584,
8.));
#12724=CARTESIAN_POINT('Ctrl Pts',(-16.6666981633995,-9.4918110794608,8.));
#12725=CARTESIAN_POINT('Ctrl Pts',(-16.6611584002427,-9.47882107274358,
8.));
#12726=CARTESIAN_POINT('Ctrl Pts',(-16.6554652571167,-9.46589453727988,
8.));
#12727=CARTESIAN_POINT('Ctrl Pts',(-16.6501414525651,-9.45380660152724,
8.));
#12728=CARTESIAN_POINT('Ctrl Pts',(-16.6446827491174,-9.44177279704584,
8.));
#12729=CARTESIAN_POINT('Ctrl Pts',(-16.6390983123084,-9.42981508426328,
8.));
#12730=CARTESIAN_POINT('Ctrl Pts',(-16.6114456124069,-9.37060355507962,
8.));
#12731=CARTESIAN_POINT('Ctrl Pts',(-16.5806669470622,-9.31314722135339,
8.));
#12732=CARTESIAN_POINT('Ctrl Pts',(-16.5468263465045,-9.25775959274632,
8.));
#12733=CARTESIAN_POINT('Ctrl Pts',(-16.513630640101,-9.20342747607804,8.));
#12734=CARTESIAN_POINT('Ctrl Pts',(-16.4774880716359,-9.15108525442289,
8.));
#12735=CARTESIAN_POINT('Ctrl Pts',(-16.4384245194448,-9.10106457909364,
8.));
#12736=CARTESIAN_POINT('Ctrl Pts',(-16.4006314655837,-9.05267077026559,
8.));
#12737=CARTESIAN_POINT('Ctrl Pts',(-16.3601038589244,-9.0064494922551,8.));
#12738=CARTESIAN_POINT('Ctrl Pts',(-16.3168397930964,-8.96274315872729,
8.));
#12739=CARTESIAN_POINT('Ctrl Pts',(-16.309631880704,-8.95546156331935,8.));
#12740=CARTESIAN_POINT('Ctrl Pts',(-16.3023479643107,-8.94824988022331,
8.));
#12741=CARTESIAN_POINT('Ctrl Pts',(-16.2949879778178,-8.9411098246742,8.));
#12742=CARTESIAN_POINT('Ctrl Pts',(-16.2872273416651,-8.93358109166894,
8.));
#12743=CARTESIAN_POINT('Ctrl Pts',(-16.2793821269318,-8.92613199722373,
8.));
#12744=CARTESIAN_POINT('Ctrl Pts',(-16.2714538290145,-8.91876328587892,
8.));
#12745=CARTESIAN_POINT('Origin',(0.,0.,0.));
#12746=CARTESIAN_POINT('',(-20.,10.,0.));
#12747=CARTESIAN_POINT('',(-20.,-14.,0.));
#12748=CARTESIAN_POINT('',(-20.,10.,0.));
#12749=CARTESIAN_POINT('',(-16.,14.,0.));
#12750=CARTESIAN_POINT('',(-16.,14.,0.));
#12751=CARTESIAN_POINT('',(16.,14.,0.));
#12752=CARTESIAN_POINT('',(16.,14.,0.));
#12753=CARTESIAN_POINT('',(20.,10.,0.));
#12754=CARTESIAN_POINT('',(20.,10.,0.));
#12755=CARTESIAN_POINT('',(20.,-14.,0.));
#12756=CARTESIAN_POINT('',(20.,-14.,0.));
#12757=CARTESIAN_POINT('',(-20.,-14.,0.));
#12758=CARTESIAN_POINT('',(-10.,-6.,0.));
#12759=CARTESIAN_POINT('',(-6.,-6.,0.));
#12760=CARTESIAN_POINT('',(-3.,-6.,0.));
#12761=CARTESIAN_POINT('',(-6.,-4.,0.));
#12762=CARTESIAN_POINT('',(-6.,-2.,0.));
#12763=CARTESIAN_POINT('',(-10.,-4.,0.));
#12764=CARTESIAN_POINT('',(-5.,-4.,0.));
#12765=CARTESIAN_POINT('',(-10.,-3.,0.));
#12766=CARTESIAN_POINT('',(6.,-6.,0.));
#12767=CARTESIAN_POINT('',(10.,-6.,0.));
#12768=CARTESIAN_POINT('',(5.,-6.,0.));
#12769=CARTESIAN_POINT('',(10.,-4.,0.));
#12770=CARTESIAN_POINT('',(10.,-2.,0.));
#12771=CARTESIAN_POINT('',(6.,-4.,0.));
#12772=CARTESIAN_POINT('',(3.,-4.,0.));
#12773=CARTESIAN_POINT('',(6.,-3.,0.));
#12774=CARTESIAN_POINT('',(-2.,4.,0.));
#12775=CARTESIAN_POINT('',(2.,4.,0.));
#12776=CARTESIAN_POINT('',(1.,4.,0.));
#12777=CARTESIAN_POINT('',(2.,6.,0.));
#12778=CARTESIAN_POINT('',(2.,3.,0.));
#12779=CARTESIAN_POINT('',(-2.,6.,0.));
#12780=CARTESIAN_POINT('',(-1.,6.,0.));
#12781=CARTESIAN_POINT('',(-2.,2.,0.));
#12782=CARTESIAN_POINT('Ctrl Pts',(13.6609982804014,-8.44145197141313,-1.11022302462516E-15));
#12783=CARTESIAN_POINT('Ctrl Pts',(13.6101587658985,-8.49415672193897,-1.06794690886987E-15));
#12784=CARTESIAN_POINT('Ctrl Pts',(13.5625411139953,-8.54962577124122,2.88974792760603E-16));
#12785=CARTESIAN_POINT('Ctrl Pts',(13.5181882608598,-8.60751250695679,-1.11022302462516E-16));
#12786=CARTESIAN_POINT('Ctrl Pts',(13.4726056590943,-8.66700423826799,-5.22109910359462E-16));
#12787=CARTESIAN_POINT('Ctrl Pts',(13.4304710124629,-8.72905053741109,-2.35827857905889E-15));
#12788=CARTESIAN_POINT('Ctrl Pts',(13.3918784169615,-8.79330181954066,-3.3584246494911E-15));
#12789=CARTESIAN_POINT('Ctrl Pts',(13.3592682533102,-8.84759318807451,-4.20353305974852E-15));
#12790=CARTESIAN_POINT('Ctrl Pts',(13.3291878694,-8.90345971497981,-1.99390072014143E-15));
#12791=CARTESIAN_POINT('Ctrl Pts',(13.3017223445621,-8.96069685037408,-2.05391259555654E-15));
#12792=CARTESIAN_POINT('Ctrl Pts',(13.2895237825855,-8.9861182012344,-2.08056632185161E-15));
#12793=CARTESIAN_POINT('Ctrl Pts',(13.2778413813041,-9.01180994946495,-6.14394228437601E-16));
#12794=CARTESIAN_POINT('Ctrl Pts',(13.2666843062596,-9.03775415254288,-6.66133814775094E-16));
#12795=CARTESIAN_POINT('Ctrl Pts',(13.2605517074626,-9.0520146453648,-6.94573000105211E-16));
#12796=CARTESIAN_POINT('Ctrl Pts',(13.2545778422614,-9.06635140970031,5.42362793670161E-16));
#12797=CARTESIAN_POINT('Ctrl Pts',(13.2487643717516,-9.08076144522329,5.82867087928207E-16));
#12798=CARTESIAN_POINT('Ctrl Pts',(13.2434046675288,-9.09404671571921,6.20209848437461E-16));
#12799=CARTESIAN_POINT('Ctrl Pts',(13.238180662491,-9.10739625085751,-2.23585955336618E-15));
#12800=CARTESIAN_POINT('Ctrl Pts',(13.2331012669984,-9.12078688698765,-2.13717932240343E-15));
#12801=CARTESIAN_POINT('Ctrl Pts',(13.2071398037565,-9.18922820213755,-1.63281158955259E-15));
#12802=CARTESIAN_POINT('Ctrl Pts',(13.1849033194385,-9.25885913230428,-1.93388574546088E-15));
#12803=CARTESIAN_POINT('Ctrl Pts',(13.166476514568,-9.32935142061032,-1.60982338570648E-15));
#12804=CARTESIAN_POINT('Ctrl Pts',(13.1481932910496,-9.39929443419718,-1.28828611438278E-15));
#12805=CARTESIAN_POINT('Ctrl Pts',(13.1336605333199,-9.47008645034364,-1.68393081631434E-15));
#12806=CARTESIAN_POINT('Ctrl Pts',(13.1230118477655,-9.54140923520067,-2.1094237467878E-15));
#12807=CARTESIAN_POINT('Ctrl Pts',(13.1141608028635,-9.6006917793311,-2.46308777545049E-15));
#12808=CARTESIAN_POINT('Ctrl Pts',(13.107994013581,-9.66034132438599,-1.11721423492157E-15));
#12809=CARTESIAN_POINT('Ctrl Pts',(13.1046159053985,-9.72016898875187,-1.13797860024079E-15));
#12810=CARTESIAN_POINT('Ctrl Pts',(13.1032060629936,-9.74513786886308,-1.14664454021581E-15));
#12811=CARTESIAN_POINT('Ctrl Pts',(13.1022822552789,-9.7701376692114,2.01322589821468E-15));
#12812=CARTESIAN_POINT('Ctrl Pts',(13.1018534077158,-9.7951541096622,2.38697950294409E-15));
#12813=CARTESIAN_POINT('Ctrl Pts',(13.1016548070149,-9.80673930457659,2.56006601256404E-15));
#12814=CARTESIAN_POINT('Ctrl Pts',(13.1015623689196,-9.8183280627853,4.77538944853251E-16));
#12815=CARTESIAN_POINT('Ctrl Pts',(13.1015770379907,-9.82991893585887,6.10622663543836E-16));
#12816=CARTESIAN_POINT('Ctrl Pts',(13.1015923232661,-9.84199670727381,7.49296836161562E-16));
#12817=CARTESIAN_POINT('Ctrl Pts',(13.1017239212966,-9.85406846363438,-1.57579408396219E-15));
#12818=CARTESIAN_POINT('Ctrl Pts',(13.1019722848962,-9.86612818157873,-1.52655665885959E-15));
#12819=CARTESIAN_POINT('Ctrl Pts',(13.1033874555188,-9.93484420350411,-1.24600283508758E-15));
#12820=CARTESIAN_POINT('Ctrl Pts',(13.1085897217447,-10.0032172387899,-5.54350890407896E-16));
#12821=CARTESIAN_POINT('Ctrl Pts',(13.1176919287551,-10.0709665059013,-3.05311331771918E-16));
#12822=CARTESIAN_POINT('Ctrl Pts',(13.1259447254805,-10.1323934685191,-7.95119348054797E-17));
#12823=CARTESIAN_POINT('Ctrl Pts',(13.1374040930353,-10.1933080511867,1.4078718797507E-15));
#12824=CARTESIAN_POINT('Ctrl Pts',(13.1521893955025,-10.2534893792597,1.73472347597681E-15));
#12825=CARTESIAN_POINT('Ctrl Pts',(13.1696761947384,-10.3246667396211,2.121295766655E-15));
#12826=CARTESIAN_POINT('Ctrl Pts',(13.1918154833854,-10.3948200423067,3.90173504212154E-16));
#12827=CARTESIAN_POINT('Ctrl Pts',(13.2183556262969,-10.463600226698,1.38777878078145E-16));
#12828=CARTESIAN_POINT('Ctrl Pts',(13.2242000202031,-10.478746282688,8.34181511049387E-17));
#12829=CARTESIAN_POINT('Ctrl Pts',(13.2302579878528,-10.4938255820364,1.17983157929043E-15));
#12830=CARTESIAN_POINT('Ctrl Pts',(13.2365271040103,-10.5088340883018,1.27675647831893E-15));
#12831=CARTESIAN_POINT('Ctrl Pts',(13.2429827911969,-10.5242892528182,1.37656589530753E-15));
#12832=CARTESIAN_POINT('Ctrl Pts',(13.249665027142,-10.5396748622705,1.08718752268941E-15));
#12833=CARTESIAN_POINT('Ctrl Pts',(13.2565569191837,-10.5549556510553,1.04083408558608E-15));
#12834=CARTESIAN_POINT('Ctrl Pts',(13.284756021213,-10.6174790509322,8.51172771336908E-16));
#12835=CARTESIAN_POINT('Ctrl Pts',(13.3164923441765,-10.6783312930776,2.50909797921603E-15));
#12836=CARTESIAN_POINT('Ctrl Pts',(13.3515101424189,-10.7372595582005,2.26207941267376E-15));
#12837=CARTESIAN_POINT('Ctrl Pts',(13.386520648505,-10.7961755520174,2.01511228563007E-15));
#12838=CARTESIAN_POINT('Ctrl Pts',(13.4248121377808,-10.8531691394787,-1.01449280433253E-15));
#12839=CARTESIAN_POINT('Ctrl Pts',(13.4661672023612,-10.9079526014265,-9.99200722162641E-16));
#12840=CARTESIAN_POINT('Ctrl Pts',(13.4961034954915,-10.9476095042072,-9.88131019840704E-16));
#12841=CARTESIAN_POINT('Ctrl Pts',(13.5276459606208,-10.9861075874816,1.68431897089301E-15));
#12842=CARTESIAN_POINT('Ctrl Pts',(13.5607207523854,-11.0233228320109,2.00534033822919E-15));
#12843=CARTESIAN_POINT('Ctrl Pts',(13.5855273390455,-11.0512348199399,2.246111147165E-15));
#12844=CARTESIAN_POINT('Ctrl Pts',(13.6111960512469,-11.07842493416,-3.45593041235091E-16));
#12845=CARTESIAN_POINT('Ctrl Pts',(13.6376974486013,-11.1048353845436,-5.48172618408671E-16));
#12846=CARTESIAN_POINT('Ctrl Pts',(13.646504369492,-11.1136120820175,-6.15493684025071E-16));
#12847=CARTESIAN_POINT('Ctrl Pts',(13.6553963636123,-11.1222957620102,-1.38096788297345E-15));
#12848=CARTESIAN_POINT('Ctrl Pts',(13.6643717837757,-11.1308844426468,-1.19348975147204E-15));
#12849=CARTESIAN_POINT('Ctrl Pts',(13.7119764880025,-11.1764379202511,-1.99125049143139E-16));
#12850=CARTESIAN_POINT('Ctrl Pts',(13.7619290644544,-11.2193251985614,1.6044485410188E-16));
#12851=CARTESIAN_POINT('Ctrl Pts',(13.8140392685458,-11.2592667110007,-3.2612801348364E-16));
#12852=CARTESIAN_POINT('Ctrl Pts',(13.8507160970753,-11.287378825096,-6.68593562078286E-16));
#12853=CARTESIAN_POINT('Ctrl Pts',(13.8884623109934,-11.3140308200616,9.18435597775855E-16));
#12854=CARTESIAN_POINT('Ctrl Pts',(13.927216032338,-11.3391104485778,-4.5102810375397E-17));
#12855=CARTESIAN_POINT('Ctrl Pts',(13.9396521575986,-11.3471585376618,-3.54303679903529E-16));
#12856=CARTESIAN_POINT('Ctrl Pts',(13.9521937968018,-11.3550456673736,-3.44690438430398E-16));
#12857=CARTESIAN_POINT('Ctrl Pts',(13.9648333834986,-11.3627644446501,-1.42247325030098E-16));
#12858=CARTESIAN_POINT('Ctrl Pts',(14.018677675764,-11.3956462239028,7.20154779289231E-16));
#12859=CARTESIAN_POINT('Ctrl Pts',(14.0741898030955,-11.4254114396644,4.93984524176593E-16));
#12860=CARTESIAN_POINT('Ctrl Pts',(14.1312019479731,-11.4517907289967,1.56125112837913E-15));
#12861=CARTESIAN_POINT('Ctrl Pts',(14.1837968166844,-11.4761261624751,2.54582638069662E-15));
#12862=CARTESIAN_POINT('Ctrl Pts',(14.23766883648,-11.4975798614081,-2.36021162522633E-16));
#12863=CARTESIAN_POINT('Ctrl Pts',(14.2926912967956,-11.5159012511454,3.64725610824124E-16));
#12864=CARTESIAN_POINT('Ctrl Pts',(14.3029516288356,-11.5193177385409,4.87279518509108E-16));
#12865=CARTESIAN_POINT('Ctrl Pts',(14.3132519680667,-11.5226251912698,1.24120044379145E-15));
#12866=CARTESIAN_POINT('Ctrl Pts',(14.3235906297078,-11.5258236994894,1.26287869051112E-15));
#12867=CARTESIAN_POINT('Ctrl Pts',(16.6117095221421,-10.4218393251423,0.));
#12868=CARTESIAN_POINT('Ctrl Pts',(16.6342056422671,-10.3640626285304,1.03253723969441E-17));
#12869=CARTESIAN_POINT('Ctrl Pts',(16.6531280196217,-10.3051560572626,9.85900667902734E-16));
#12870=CARTESIAN_POINT('Ctrl Pts',(16.668627359564,-10.2454298235342,9.71445146547012E-16));
#12871=CARTESIAN_POINT('Ctrl Pts',(16.6851480739499,-10.1817677545397,9.56037036233499E-16));
#12872=CARTESIAN_POINT('Ctrl Pts',(16.6977802955953,-10.1171739101123,-1.65277777837953E-15));
#12873=CARTESIAN_POINT('Ctrl Pts',(16.7066568337424,-10.0519871771322,-2.33146835171283E-15));
#12874=CARTESIAN_POINT('Ctrl Pts',(16.7144238046212,-9.99494878577466,-2.92532260337946E-15));
#12875=CARTESIAN_POINT('Ctrl Pts',(16.7193145800233,-9.93745546561697,6.8060116455104E-16));
#12876=CARTESIAN_POINT('Ctrl Pts',(16.7213855572738,-9.8797193559252,6.10622663543836E-16));
#12877=CARTESIAN_POINT('Ctrl Pts',(16.7224250203391,-9.85074049893983,5.75499116364019E-16));
#12878=CARTESIAN_POINT('Ctrl Pts',(16.7227536323972,-9.8217003136112,-1.02322656074148E-15));
#12879=CARTESIAN_POINT('Ctrl Pts',(16.7223756111595,-9.79262498025395,-1.52655665885959E-15));
#12880=CARTESIAN_POINT('Ctrl Pts',(16.722203203288,-9.77936430641241,-1.75611537737089E-15));
#12881=CARTESIAN_POINT('Ctrl Pts',(16.7218836016271,-9.76609460618316,6.45474011158562E-16));
#12882=CARTESIAN_POINT('Ctrl Pts',(16.7214181907915,-9.75283991662234,5.82867087928207E-16));
#12883=CARTESIAN_POINT('Ctrl Pts',(16.7190676596557,-9.68589785571542,2.66674358641745E-16));
#12884=CARTESIAN_POINT('Ctrl Pts',(16.7130015751494,-9.61921857039721,-3.30153071919369E-15));
#12885=CARTESIAN_POINT('Ctrl Pts',(16.7033535912675,-9.55313453802705,-2.60902410786912E-15));
#12886=CARTESIAN_POINT('Ctrl Pts',(16.6935350874628,-9.4858825264979,-1.90427803020938E-15));
#12887=CARTESIAN_POINT('Ctrl Pts',(16.6800070889265,-9.41924599491758,2.56425075671755E-15));
#12888=CARTESIAN_POINT('Ctrl Pts',(16.6628592032612,-9.35355953164192,2.74780198594726E-15));
#12889=CARTESIAN_POINT('Ctrl Pts',(16.6485159926896,-9.2986166195617,2.90133193027481E-15));
#12890=CARTESIAN_POINT('Ctrl Pts',(16.6316392742217,-9.24433780152903,5.69878197833297E-16));
#12891=CARTESIAN_POINT('Ctrl Pts',(16.6122537800222,-9.19091858497507,8.04911692853238E-16));
#12892=CARTESIAN_POINT('Ctrl Pts',(16.6033176258644,-9.16629386562554,9.13255360655956E-16));
#12893=CARTESIAN_POINT('Ctrl Pts',(16.5938480192675,-9.14185185036756,1.2939697659665E-15));
#12894=CARTESIAN_POINT('Ctrl Pts',(16.583845579661,-9.11761211165287,1.19348975147204E-15));
#12895=CARTESIAN_POINT('Ctrl Pts',(16.5794871167385,-9.10704988817558,1.14970659107644E-15));
#12896=CARTESIAN_POINT('Ctrl Pts',(16.5750275002003,-9.09652638012247,1.4297108069045E-15));
#12897=CARTESIAN_POINT('Ctrl Pts',(16.5704725567595,-9.08605595522034,1.4432899320127E-15));
#12898=CARTESIAN_POINT('Ctrl Pts',(16.5424799759779,-9.02170955472239,1.52674096965357E-15));
#12899=CARTESIAN_POINT('Ctrl Pts',(16.5108410959836,-8.95924447434619,8.11841053369489E-16));
#12900=CARTESIAN_POINT('Ctrl Pts',(16.4756627651242,-8.89900929869964,6.10622663543836E-16));
#12901=CARTESIAN_POINT('Ctrl Pts',(16.4442081085769,-8.84515009856861,4.30703514785051E-16));
#12902=CARTESIAN_POINT('Ctrl Pts',(16.409922923172,-8.79307299455403,-1.06964934127292E-15));
#12903=CARTESIAN_POINT('Ctrl Pts',(16.3728484580761,-8.7430306263865,-1.69309011255336E-15));
#12904=CARTESIAN_POINT('Ctrl Pts',(16.3324636346748,-8.68852000308266,-2.37371681853972E-15));
#12905=CARTESIAN_POINT('Ctrl Pts',(16.2887698044348,-8.63642247738161,1.13943955051508E-15));
#12906=CARTESIAN_POINT('Ctrl Pts',(16.2420808769759,-8.58682415987058,1.08246744900953E-15));
#12907=CARTESIAN_POINT('Ctrl Pts',(16.2240717422292,-8.56769279764222,1.06049182633702E-15));
#12908=CARTESIAN_POINT('Ctrl Pts',(16.2056165049632,-8.54893356154431,1.05886801823215E-15));
#12909=CARTESIAN_POINT('Ctrl Pts',(16.1867315129249,-8.53055255076451,9.85322934354826E-16));
#12910=CARTESIAN_POINT('Ctrl Pts',(16.1784458604514,-8.52248801639111,9.53055565382105E-16));
#12911=CARTESIAN_POINT('Ctrl Pts',(16.1700778405889,-8.51449677522097,2.6086384421045E-15));
#12912=CARTESIAN_POINT('Ctrl Pts',(16.1616388232942,-8.50658839906083,2.60902410786912E-15));
#12913=CARTESIAN_POINT('Ctrl Pts',(16.110613081093,-8.45877112969359,2.61135600045729E-15));
#12914=CARTESIAN_POINT('Ctrl Pts',(16.0569055066012,-8.41389261610438,-1.10985713633557E-15));
#12915=CARTESIAN_POINT('Ctrl Pts',(16.0008930531355,-8.37201442081571,-6.80011602582908E-16));
#12916=CARTESIAN_POINT('Ctrl Pts',(15.9435806322954,-8.32916429367614,-2.40189980740859E-16));
#12917=CARTESIAN_POINT('Ctrl Pts',(15.8838544772616,-8.28945475968816,2.49235514291959E-15));
#12918=CARTESIAN_POINT('Ctrl Pts',(15.8220694152881,-8.25297945854376,1.84574577843932E-15));
#12919=CARTESIAN_POINT('Ctrl Pts',(15.7747998187522,-8.22507347749358,1.35104750026396E-15));
#12920=CARTESIAN_POINT('Ctrl Pts',(15.7263239837791,-8.19906107141398,1.04416537528888E-15));
#12921=CARTESIAN_POINT('Ctrl Pts',(15.6767858652511,-8.17499812306594,1.18655085756814E-15));
#12922=CARTESIAN_POINT('Ctrl Pts',(15.6459600566815,-8.1600246064804,1.2751522770456E-15));
#12923=CARTESIAN_POINT('Ctrl Pts',(15.6147226803593,-8.1458061957273,7.80813838002484E-16));
#12924=CARTESIAN_POINT('Ctrl Pts',(15.5831065420217,-8.13235912807096,4.71844785465692E-16));
#12925=CARTESIAN_POINT('Ctrl Pts',(15.5653369179383,-8.12480130001724,2.9819094265975E-16));
#12926=CARTESIAN_POINT('Ctrl Pts',(15.5474415799036,-8.11748495921732,1.28072228025138E-15));
#12927=CARTESIAN_POINT('Ctrl Pts',(15.5294589734096,-8.11042570470516,1.31838984174237E-15));
#12928=CARTESIAN_POINT('Ctrl Pts',(15.4598209192961,-8.08308858047443,1.46425833340463E-15));
#12929=CARTESIAN_POINT('Ctrl Pts',(15.3888075307889,-8.05957130809681,1.44681167701246E-15));
#12930=CARTESIAN_POINT('Ctrl Pts',(15.3167904926731,-8.03998814314756,1.67921232474555E-15));
#12931=CARTESIAN_POINT('Ctrl Pts',(15.2629156508911,-8.02533827777076,1.85306768528583E-15));
#12932=CARTESIAN_POINT('Ctrl Pts',(15.2084781793224,-8.01289073961062,7.0540273618505E-16));
#12933=CARTESIAN_POINT('Ctrl Pts',(15.1536231312556,-8.00270927344064,9.29811783123569E-16));
#12934=CARTESIAN_POINT('Ctrl Pts',(15.1365390635248,-7.99953835547088,9.99701783996981E-16));
#12935=CARTESIAN_POINT('Ctrl Pts',(15.1194144432163,-7.99658734404714,-1.52249784740926E-15));
#12936=CARTESIAN_POINT('Ctrl Pts',(15.1022535343896,-7.99385847048614,-1.51961776495568E-15));
#12937=CARTESIAN_POINT('Ctrl Pts',(15.0856549353801,-7.99121901365762,-1.51683205388155E-15));
#12938=CARTESIAN_POINT('Ctrl Pts',(15.0690308306928,-7.98878877172398,2.00705548056742E-15));
#12939=CARTESIAN_POINT('Ctrl Pts',(15.0523912277109,-7.98656991749699,1.82839854367955E-15));
#12940=CARTESIAN_POINT('Ctrl Pts',(14.977715101503,-7.9766120213578,1.02661210794354E-15));
#12941=CARTESIAN_POINT('Ctrl Pts',(14.9026909367617,-7.97090197782506,7.13283686621106E-16));
#12942=CARTESIAN_POINT('Ctrl Pts',(14.8276757175273,-7.96957803638134,3.23699400617272E-15));
#12943=CARTESIAN_POINT('Ctrl Pts',(14.7702213490998,-7.96856402588774,5.16991087269235E-15));
#12944=CARTESIAN_POINT('Ctrl Pts',(14.7127715253326,-7.97012372111896,2.66678155952208E-16));
#12945=CARTESIAN_POINT('Ctrl Pts',(14.655480726337,-7.97433912128626,1.48145384848419E-15));
#12946=CARTESIAN_POINT('Ctrl Pts',(14.6422349512898,-7.97531373227666,1.75566928754182E-15));
#12947=CARTESIAN_POINT('Ctrl Pts',(14.6289976663039,-7.97643038184829,8.63526738818194E-16));
#12948=CARTESIAN_POINT('Ctrl Pts',(14.615770327818,-7.97768772784116,8.74300631892311E-16));
#12949=CARTESIAN_POINT('Ctrl Pts',(-16.3390017195986,11.5585480285869,0.));
#12950=CARTESIAN_POINT('Ctrl Pts',(-16.3898412778797,11.5058432326767,-1.21950438921618E-16));
#12951=CARTESIAN_POINT('Ctrl Pts',(-16.4374589773482,11.4503741465571,2.81930744747739E-15));
#12952=CARTESIAN_POINT('Ctrl Pts',(-16.481811879575,11.3924873804857,1.94289029309402E-15));
#12953=CARTESIAN_POINT('Ctrl Pts',(-16.5273944957859,11.3329956649711,1.04217388485006E-15));
#12954=CARTESIAN_POINT('Ctrl Pts',(-16.5695291639216,11.2709493924853,-9.44439383800379E-17));
#12955=CARTESIAN_POINT('Ctrl Pts',(-16.6081217856935,11.2066981448109,2.4980018054066E-16));
#12956=CARTESIAN_POINT('Ctrl Pts',(-16.6407319648364,11.1524068165565,5.40681231670983E-16));
#12957=CARTESIAN_POINT('Ctrl Pts',(-16.6708123686837,11.0965403361506,-4.80669364326135E-16));
#12958=CARTESIAN_POINT('Ctrl Pts',(-16.6982779165735,11.0393032515191,-2.4980018054066E-16));
#12959=CARTESIAN_POINT('Ctrl Pts',(-16.7104764723248,11.0138819575139,-1.47261879794735E-16));
#12960=CARTESIAN_POINT('Ctrl Pts',(-16.7221588693883,10.9881902677093,-1.31648042932263E-15));
#12961=CARTESIAN_POINT('Ctrl Pts',(-16.733315942143,10.9622461243824,-1.63757896132211E-15));
#12962=CARTESIAN_POINT('Ctrl Pts',(-16.7394485566319,10.9479856249873,-1.81407449496283E-15));
#12963=CARTESIAN_POINT('Ctrl Pts',(-16.7454224372302,10.9336488540573,3.90657944783047E-16));
#12964=CARTESIAN_POINT('Ctrl Pts',(-16.7512359228157,10.9192388119023,4.44089209850063E-16));
#12965=CARTESIAN_POINT('Ctrl Pts',(-16.7565956237565,10.9059535778792,4.93349777788063E-16));
#12966=CARTESIAN_POINT('Ctrl Pts',(-16.761819626096,10.8926040796307,2.41764770258606E-15));
#12967=CARTESIAN_POINT('Ctrl Pts',(-16.7668990194954,10.8792134806461,2.3037127760972E-15));
#12968=CARTESIAN_POINT('Ctrl Pts',(-16.7928605213173,10.8107722254404,1.72137516822412E-15));
#12969=CARTESIAN_POINT('Ctrl Pts',(-16.8150970458508,10.7411413575974,8.00179814752099E-16));
#12970=CARTESIAN_POINT('Ctrl Pts',(-16.8335238904444,10.6706491309863,8.32667268468867E-16));
#12971=CARTESIAN_POINT('Ctrl Pts',(-16.8518071488745,10.6007061958358,8.64901572558164E-16));
#12972=CARTESIAN_POINT('Ctrl Pts',(-16.8663399428806,10.5299142579317,1.40567801852473E-15));
#12973=CARTESIAN_POINT('Ctrl Pts',(-16.8769886640788,10.4585915479125,1.52655665885959E-15));
#12974=CARTESIAN_POINT('Ctrl Pts',(-16.8858397414576,10.3993090468971,1.6270293991195E-15));
#12975=CARTESIAN_POINT('Ctrl Pts',(-16.8920065610542,10.3396595423699,-2.49297590265314E-16));
#12976=CARTESIAN_POINT('Ctrl Pts',(-16.8953846961167,10.2798319142083,-5.82867087928207E-16));
#12977=CARTESIAN_POINT('Ctrl Pts',(-16.8967945502735,10.2548630397562,-7.22081279834834E-16));
#12978=CARTESIAN_POINT('Ctrl Pts',(-16.8977183687733,10.2298632442895,5.3650467142801E-16));
#12979=CARTESIAN_POINT('Ctrl Pts',(-16.8981472260481,10.204846807828,6.93889390390723E-16));
#12980=CARTESIAN_POINT('Ctrl Pts',(-16.8983458313901,10.1932616063874,7.66774818164271E-16));
#12981=CARTESIAN_POINT('Ctrl Pts',(-16.8984382737427,10.1816728414559,-1.02272625117412E-16));
#12982=CARTESIAN_POINT('Ctrl Pts',(-16.8984236085324,10.1700819614545,0.));
#12983=CARTESIAN_POINT('Ctrl Pts',(-16.8984083273101,10.1580042066539,1.06568585718969E-16));
#12984=CARTESIAN_POINT('Ctrl Pts',(-16.8982767333587,10.1459324667248,-2.21252032439505E-15));
#12985=CARTESIAN_POINT('Ctrl Pts',(-16.8980283738539,10.1338727649305,-2.19269047363468E-15));
#12986=CARTESIAN_POINT('Ctrl Pts',(-16.896613225799,10.0651567979331,-2.07970033559832E-15));
#12987=CARTESIAN_POINT('Ctrl Pts',(-16.8914109785722,9.9967838096264,-4.70442234551077E-16));
#12988=CARTESIAN_POINT('Ctrl Pts',(-16.8823087851953,9.92903457865317,-2.63677968348475E-16));
#12989=CARTESIAN_POINT('Ctrl Pts',(-16.8740559966144,9.86760761741545,-7.62086733775636E-17));
#12990=CARTESIAN_POINT('Ctrl Pts',(-16.8625966295214,9.80669302774072,1.74687322657192E-15));
#12991=CARTESIAN_POINT('Ctrl Pts',(-16.847811318262,9.74651168233438,1.66533453693773E-15));
#12992=CARTESIAN_POINT('Ctrl Pts',(-16.8303245125967,9.67533431762835,1.57054602216588E-15));
#12993=CARTESIAN_POINT('Ctrl Pts',(-16.8081852066777,9.60518099567779,-6.91253892319818E-16));
#12994=CARTESIAN_POINT('Ctrl Pts',(-16.7816450379385,9.53640078021501,-1.22124532708767E-15));
#12995=CARTESIAN_POINT('Ctrl Pts',(-16.7758006405534,9.52125472310633,-1.33795447788192E-15));
#12996=CARTESIAN_POINT('Ctrl Pts',(-16.7697426691712,9.50617542201614,2.209254994723E-16));
#12997=CARTESIAN_POINT('Ctrl Pts',(-16.7634735490492,9.49116691341438,2.77555756156289E-16));
#12998=CARTESIAN_POINT('Ctrl Pts',(-16.7570178531025,9.47571173529349,3.35871390794366E-16));
#12999=CARTESIAN_POINT('Ctrl Pts',(-16.7503356078206,9.46032611170409,-3.0677869516106E-15));
#13000=CARTESIAN_POINT('Ctrl Pts',(-16.74344370592,9.44504530833083,-2.96984659087229E-15));
#13001=CARTESIAN_POINT('Ctrl Pts',(-16.715244572443,9.38252186847721,-2.56911057560626E-15));
#13002=CARTESIAN_POINT('Ctrl Pts',(-16.6835082115129,9.32166957773068,-2.6303592251713E-15));
#13003=CARTESIAN_POINT('Ctrl Pts',(-16.6484903707908,9.26274125810786,-2.22044604925031E-15));
#13004=CARTESIAN_POINT('Ctrl Pts',(-16.61347982519,9.20382521477699,-1.810618268838E-15));
#13005=CARTESIAN_POINT('Ctrl Pts',(-16.5751882924367,9.14683157157451,-1.33283324348233E-15));
#13006=CARTESIAN_POINT('Ctrl Pts',(-16.5338331823285,9.09204805026436,-8.46545056276682E-16));
#13007=CARTESIAN_POINT('Ctrl Pts',(-16.503896892843,9.05239115299845,-4.94528971504313E-16));
#13008=CARTESIAN_POINT('Ctrl Pts',(-16.4723544342098,9.01389307050919,-5.66796375334866E-16));
#13009=CARTESIAN_POINT('Ctrl Pts',(-16.4392796522632,8.97667782257107,-1.04083408558608E-16));
#13010=CARTESIAN_POINT('Ctrl Pts',(-16.4144730709346,8.94876582979876,2.42958239687017E-16));
#13011=CARTESIAN_POINT('Ctrl Pts',(-16.388804365793,8.92157570849334,-2.11364162782013E-15));
#13012=CARTESIAN_POINT('Ctrl Pts',(-16.362302977449,8.89516524900551,-2.22738494315422E-15));
#13013=CARTESIAN_POINT('Ctrl Pts',(-16.3534959930271,8.88638848220873,-2.26518430646481E-15));
#13014=CARTESIAN_POINT('Ctrl Pts',(-16.3446039340464,8.87770473382657,-1.94670993893357E-15));
#13015=CARTESIAN_POINT('Ctrl Pts',(-16.3356284481052,8.8691159861548,-2.00534033822919E-15));
#13016=CARTESIAN_POINT('Ctrl Pts',(-16.2880237162768,8.82356246043644,-2.31630783946E-15));
#13017=CARTESIAN_POINT('Ctrl Pts',(-16.2380711146439,8.78067513260799,-9.30438712188027E-16));
#13018=CARTESIAN_POINT('Ctrl Pts',(-16.1859608893929,8.7407335713535,-1.61676227961038E-15));
#13019=CARTESIAN_POINT('Ctrl Pts',(-16.1492840602602,8.71262143385326,-2.09981857212978E-15));
#13020=CARTESIAN_POINT('Ctrl Pts',(-16.1115378485653,8.6859694146933,-7.92101159662489E-16));
#13021=CARTESIAN_POINT('Ctrl Pts',(-16.0727841327849,8.66088976180095,2.77555756156289E-17));
#13022=CARTESIAN_POINT('Ctrl Pts',(-16.0603479962521,8.6528416564443,2.90849064636273E-16));
#13023=CARTESIAN_POINT('Ctrl Pts',(-16.0478063459813,8.64495451082727,-3.48235544776103E-16));
#13024=CARTESIAN_POINT('Ctrl Pts',(-16.0351667481742,8.63723571788537,-4.54497550705923E-16));
#13025=CARTESIAN_POINT('Ctrl Pts',(-15.9813224568397,8.60435390137038,-9.07170372454036E-16));
#13026=CARTESIAN_POINT('Ctrl Pts',(-15.9258103363421,8.57458864949673,-5.08306115800648E-15));
#13027=CARTESIAN_POINT('Ctrl Pts',(-15.8687982055922,8.54820932690989,-3.87710696880816E-15));
#13028=CARTESIAN_POINT('Ctrl Pts',(-15.8162032016611,8.52387379415743,-2.76458644927628E-15));
#13029=CARTESIAN_POINT('Ctrl Pts',(-15.7623310456534,8.5024200146067,1.66508848905326E-17));
#13030=CARTESIAN_POINT('Ctrl Pts',(-15.7073084503787,8.48409856643006,6.50521303491303E-16));
#13031=CARTESIAN_POINT('Ctrl Pts',(-15.6970481156835,8.4806820756329,7.77638078926068E-16));
#13032=CARTESIAN_POINT('Ctrl Pts',(-15.6867477740167,8.47737461979661,7.70550576036819E-19));
#13033=CARTESIAN_POINT('Ctrl Pts',(-15.676409110153,8.47417610875465,5.55111512312578E-17));
#13034=CARTESIAN_POINT('Ctrl Pts',(-13.3882904778579,9.57816067485776,0.));
#13035=CARTESIAN_POINT('Ctrl Pts',(-13.3657943888576,9.63593729153216,-1.35606369860236E-16));
#13036=CARTESIAN_POINT('Ctrl Pts',(-13.3468720478727,9.69484378534804,4.93527622464658E-16));
#13037=CARTESIAN_POINT('Ctrl Pts',(-13.3313727466823,9.75456994412679,8.32667268468867E-17));
#13038=CARTESIAN_POINT('Ctrl Pts',(-13.3148520480641,9.81823203164207,-3.54030189194023E-16));
#13039=CARTESIAN_POINT('Ctrl Pts',(-13.3022198569086,9.88282590030355,1.2868821931612E-15));
#13040=CARTESIAN_POINT('Ctrl Pts',(-13.2933433599697,9.94801266163332,2.44249065417534E-15));
#13041=CARTESIAN_POINT('Ctrl Pts',(-13.2855764251482,10.0050510777969,3.45364805756272E-15));
#13042=CARTESIAN_POINT('Ctrl Pts',(-13.2806856940185,10.0625444259155,-6.74181128899614E-16));
#13043=CARTESIAN_POINT('Ctrl Pts',(-13.2786147667243,10.1202805657223,-6.10622663543836E-16));
#13044=CARTESIAN_POINT('Ctrl Pts',(-13.2775753306189,10.1492593852438,-5.78721512847333E-16));
#13045=CARTESIAN_POINT('Ctrl Pts',(-13.2772467443753,10.1782995334297,1.05553020072304E-15));
#13046=CARTESIAN_POINT('Ctrl Pts',(-13.2776247899912,10.2073748299843,1.16573417585641E-15));
#13047=CARTESIAN_POINT('Ctrl Pts',(-13.2777972103524,10.2206355925021,1.21599638865992E-15));
#13048=CARTESIAN_POINT('Ctrl Pts',(-13.2781168265499,10.233905381765,-2.37994547501183E-15));
#13049=CARTESIAN_POINT('Ctrl Pts',(-13.2785822538993,10.2471601602663,-2.16493489801906E-15));
#13050=CARTESIAN_POINT('Ctrl Pts',(-13.2809328514967,10.3141021879349,-1.07904394987729E-15));
#13051=CARTESIAN_POINT('Ctrl Pts',(-13.2869989993311,10.3807814420985,-1.19769074053069E-15));
#13052=CARTESIAN_POINT('Ctrl Pts',(-13.2966470399663,10.4468654449278,-8.88178419700125E-16));
#13053=CARTESIAN_POINT('Ctrl Pts',(-13.306465606786,10.5141174624129,-5.73195562712684E-16));
#13054=CARTESIAN_POINT('Ctrl Pts',(-13.3199936655056,10.5807540009591,2.66789730521724E-15));
#13055=CARTESIAN_POINT('Ctrl Pts',(-13.3371416047229,10.6464404711977,2.94209101525666E-15));
#13056=CARTESIAN_POINT('Ctrl Pts',(-13.3514848727063,10.7013834374385,3.17143833289168E-15));
#13057=CARTESIAN_POINT('Ctrl Pts',(-13.3683616484046,10.755662308463,1.19948474334804E-15));
#13058=CARTESIAN_POINT('Ctrl Pts',(-13.3877471973421,10.8090815757484,9.99200722162641E-16));
#13059=CARTESIAN_POINT('Ctrl Pts',(-13.396683355205,10.8337062591617,9.06875782771859E-16));
#13060=CARTESIAN_POINT('Ctrl Pts',(-13.406152962408,10.8581482388832,2.06346452769943E-15));
#13061=CARTESIAN_POINT('Ctrl Pts',(-13.4161553992987,10.8823879424951,2.22044604925031E-15));
#13062=CARTESIAN_POINT('Ctrl Pts',(-13.4205138927756,10.892950227589,2.28884967380167E-15));
#13063=CARTESIAN_POINT('Ctrl Pts',(-13.4249735407989,10.9034737969884,6.01283625265369E-16));
#13064=CARTESIAN_POINT('Ctrl Pts',(-13.4295285164776,10.9139442825721,6.66133814775094E-16));
#13065=CARTESIAN_POINT('Ctrl Pts',(-13.4575211485423,10.9782907184605,1.06467106772917E-15));
#13066=CARTESIAN_POINT('Ctrl Pts',(-13.4891600706501,11.0407558305742,3.69548560173297E-15));
#13067=CARTESIAN_POINT('Ctrl Pts',(-13.5243384304155,11.1009910327419,3.41393580072236E-15));
#13068=CARTESIAN_POINT('Ctrl Pts',(-13.5557931413997,11.1548503055419,3.16218820141692E-15));
#13069=CARTESIAN_POINT('Ctrl Pts',(-13.5900783758293,11.2069274748198,4.73664851661874E-16));
#13070=CARTESIAN_POINT('Ctrl Pts',(-13.6271528815519,11.2569698990377,8.04911692853238E-16));
#13071=CARTESIAN_POINT('Ctrl Pts',(-13.6675377331972,11.3114805617862,1.17809376743549E-15));
#13072=CARTESIAN_POINT('Ctrl Pts',(-13.7112315791046,11.3635781179213,1.8548613205985E-15));
#13073=CARTESIAN_POINT('Ctrl Pts',(-13.7579205122475,11.4131764577819,1.84574577843932E-15));
#13074=CARTESIAN_POINT('Ctrl Pts',(-13.7759296243692,11.432307802267,1.84222968137425E-15));
#13075=CARTESIAN_POINT('Ctrl Pts',(-13.7943848362944,11.4510670204427,2.04120230226521E-16));
#13076=CARTESIAN_POINT('Ctrl Pts',(-13.8132698004889,11.4694480131946,-1.38777878078145E-17));
#13077=CARTESIAN_POINT('Ctrl Pts',(-13.8215554419107,11.4775125407918,-1.09522841168832E-16));
#13078=CARTESIAN_POINT('Ctrl Pts',(-13.8299234502305,11.485503775114,4.05044125615248E-15));
#13079=CARTESIAN_POINT('Ctrl Pts',(-13.8383624555639,11.4934121444084,3.92741394961149E-15));
#13080=CARTESIAN_POINT('Ctrl Pts',(-13.8893881936728,11.5412294362029,3.18353965687582E-15));
#13081=CARTESIAN_POINT('Ctrl Pts',(-13.9430957557082,11.586107963496,3.38934266541307E-15));
#13082=CARTESIAN_POINT('Ctrl Pts',(-13.9991081910456,11.6279861648249,3.09474668114262E-15));
#13083=CARTESIAN_POINT('Ctrl Pts',(-14.0564205721683,11.6708362823183,2.7933136649555E-15));
#13084=CARTESIAN_POINT('Ctrl Pts',(-14.1161466797624,11.7105458009547,1.50938421367961E-15));
#13085=CARTESIAN_POINT('Ctrl Pts',(-14.1779316897435,11.747021082115,1.41553435639707E-15));
#13086=CARTESIAN_POINT('Ctrl Pts',(-14.2252011257199,11.7749269765716,1.34373328650058E-15));
#13087=CARTESIAN_POINT('Ctrl Pts',(-14.2736767913047,11.8009393030142,-9.76164430457898E-17));
#13088=CARTESIAN_POINT('Ctrl Pts',(-14.3232147340873,11.8250021795641,-4.37150315946155E-16));
#13089=CARTESIAN_POINT('Ctrl Pts',(-14.3540404755327,11.8399756719881,-6.48430453756458E-16));
#13090=CARTESIAN_POINT('Ctrl Pts',(-14.3852777833939,11.8541940595482,2.95554805743735E-15));
#13091=CARTESIAN_POINT('Ctrl Pts',(-14.4168938523755,11.8676411051472,3.06005221162309E-15));
#13092=CARTESIAN_POINT('Ctrl Pts',(-14.4346635095532,11.875198951459,3.11878826114919E-15));
#13093=CARTESIAN_POINT('Ctrl Pts',(-14.4525588814166,11.8825153089168,3.62295386493415E-15));
#13094=CARTESIAN_POINT('Ctrl Pts',(-14.4705415223192,11.889574578414,3.62210261783957E-15));
#13095=CARTESIAN_POINT('Ctrl Pts',(-14.5401794861377,11.9169116729204,3.61880615461739E-15));
#13096=CARTESIAN_POINT('Ctrl Pts',(-14.6111927842436,11.9404289151015,2.34519441392117E-15));
#13097=CARTESIAN_POINT('Ctrl Pts',(-14.6832097355402,11.9600120506473,2.49106291150269E-15));
#13098=CARTESIAN_POINT('Ctrl Pts',(-14.7370845061574,11.9746618923373,2.60018488495465E-15));
#13099=CARTESIAN_POINT('Ctrl Pts',(-14.7915219084323,11.9871094077609,9.59298669237085E-16));
#13100=CARTESIAN_POINT('Ctrl Pts',(-14.8463768906533,11.9972908526876,5.30825383648903E-16));
#13101=CARTESIAN_POINT('Ctrl Pts',(-14.8634609542423,12.0004617670789,3.97381445453818E-16));
#13102=CARTESIAN_POINT('Ctrl Pts',(-14.8805855708211,12.0034127746477,-1.21629321462611E-15));
#13103=CARTESIAN_POINT('Ctrl Pts',(-14.8977464763661,12.0061416440875,-1.23165366794353E-15));
#13104=CARTESIAN_POINT('Ctrl Pts',(-14.9143450435635,12.008781092376,-1.24651078115971E-15));
#13105=CARTESIAN_POINT('Ctrl Pts',(-14.9309691166948,12.0112113262329,1.37759135887431E-15));
#13106=CARTESIAN_POINT('Ctrl Pts',(-14.9476086885424,12.0134301728835,1.19002030452009E-15));
#13107=CARTESIAN_POINT('Ctrl Pts',(-15.0222847381472,12.0233880434379,3.48227890169128E-16));
#13108=CARTESIAN_POINT('Ctrl Pts',(-15.0973088346763,12.0290980641533,1.29347754135401E-16));
#13109=CARTESIAN_POINT('Ctrl Pts',(-15.1723239977792,12.0304219868111,1.2195106036117E-15));
#13110=CARTESIAN_POINT('Ctrl Pts',(-15.2297783091666,12.0314359826685,2.05446920699172E-15));
#13111=CARTESIAN_POINT('Ctrl Pts',(-15.2872280829805,12.029876276423,1.66503248027151E-15));
#13112=CARTESIAN_POINT('Ctrl Pts',(-15.3445188409063,12.0256608695019,1.6605640473788E-15));
#13113=CARTESIAN_POINT('Ctrl Pts',(-15.3577646096558,12.0246862567147,1.64941776864115E-15));
#13114=CARTESIAN_POINT('Ctrl Pts',(-15.371001888815,12.0235696055055,1.03965794060541E-15));
#13115=CARTESIAN_POINT('Ctrl Pts',(-15.384229221931,12.022312258029,1.0547118733939E-15));
#13116=CARTESIAN_POINT('Ctrl Pts',(13.6609982804014,11.5585480285869,0.));
#13117=CARTESIAN_POINT('Ctrl Pts',(13.6101587848434,11.505843297701,1.58535375005519E-16));
#13118=CARTESIAN_POINT('Ctrl Pts',(13.562541153526,11.4503742643279,2.04729506994165E-15));
#13119=CARTESIAN_POINT('Ctrl Pts',(13.5181883216384,11.3924875417427,2.02615701994091E-15));
#13120=CARTESIAN_POINT('Ctrl Pts',(13.4726057261298,11.3329958035915,2.00443287873015E-15));
#13121=CARTESIAN_POINT('Ctrl Pts',(13.4304710888115,11.2709494929059,-1.04515563626232E-15));
#13122=CARTESIAN_POINT('Ctrl Pts',(13.3918785046867,11.2066981958572,-9.99200722162641E-16));
#13123=CARTESIAN_POINT('Ctrl Pts',(13.359268347745,11.1524068098827,-9.60369506398756E-16));
#13124=CARTESIAN_POINT('Ctrl Pts',(13.329187972469,11.0965402628436,1.19891982664628E-15));
#13125=CARTESIAN_POINT('Ctrl Pts',(13.3017224576139,11.0393031054692,2.05391259555654E-15));
#13126=CARTESIAN_POINT('Ctrl Pts',(13.2895238929487,11.0138817300036,2.43365004577085E-15));
#13127=CARTESIAN_POINT('Ctrl Pts',(13.2778414898473,10.9881899564878,1.38699052202662E-15));
#13128=CARTESIAN_POINT('Ctrl Pts',(13.2666844138171,10.9622457275511,1.36002320516582E-15));
#13129=CARTESIAN_POINT('Ctrl Pts',(13.2605518218175,10.9479852375819,1.34520036527618E-15));
#13130=CARTESIAN_POINT('Ctrl Pts',(13.2545779632859,10.9336484761084,3.15224287654931E-15));
#13131=CARTESIAN_POINT('Ctrl Pts',(13.2487644993064,10.9192384434638,3.1641356201817E-15));
#13132=CARTESIAN_POINT('Ctrl Pts',(13.2434047935862,10.9059531569865,3.17510009958671E-15));
#13133=CARTESIAN_POINT('Ctrl Pts',(13.2381807873077,10.8926036056845,3.12885909062377E-16));
#13134=CARTESIAN_POINT('Ctrl Pts',(13.2331013908405,10.8792129532788,3.33066907387547E-16));
#13135=CARTESIAN_POINT('Ctrl Pts',(13.2071399443245,10.8107716121686,4.36214577006048E-16));
#13136=CARTESIAN_POINT('Ctrl Pts',(13.1849034774407,10.7411406550117,-1.22541225100052E-15));
#13137=CARTESIAN_POINT('Ctrl Pts',(13.1664766897913,10.6706483399882,-1.08246744900953E-15));
#13138=CARTESIAN_POINT('Ctrl Pts',(13.1481934814117,10.6007052924391,-9.40636455386775E-16));
#13139=CARTESIAN_POINT('Ctrl Pts',(13.1336607394114,10.5299132424147,1.19000295853796E-15));
#13140=CARTESIAN_POINT('Ctrl Pts',(13.1230120693126,10.4585904251542,1.11022302462516E-15));
#13141=CARTESIAN_POINT('Ctrl Pts',(13.1141610384968,10.399307862394,1.04391102068517E-15));
#13142=CARTESIAN_POINT('Ctrl Pts',(13.1079942623606,10.3396582998303,-8.10480048155446E-17));
#13143=CARTESIAN_POINT('Ctrl Pts',(13.1046161658339,10.2798306198277,0.));
#13144=CARTESIAN_POINT('Ctrl Pts',(13.1032063285254,10.2548617372976,3.38251142524164E-17));
#13145=CARTESIAN_POINT('Ctrl Pts',(13.1022825254872,10.229861934867,7.93924619007334E-16));
#13146=CARTESIAN_POINT('Ctrl Pts',(13.1018536821348,10.2048454927203,5.82867087928207E-16));
#13147=CARTESIAN_POINT('Ctrl Pts',(13.1016550834447,10.1932603005737,4.85125689003432E-16));
#13148=CARTESIAN_POINT('Ctrl Pts',(13.1015626471952,10.1816715452178,3.96242804970713E-16));
#13149=CARTESIAN_POINT('Ctrl Pts',(13.1015773179414,10.1700806750858,3.33066907387547E-16));
#13150=CARTESIAN_POINT('Ctrl Pts',(13.1015926049752,10.1580028966096,2.67237121758476E-16));
#13151=CARTESIAN_POINT('Ctrl Pts',(13.1017242047727,10.1459311332672,2.51600957460125E-15));
#13152=CARTESIAN_POINT('Ctrl Pts',(13.1019725701435,10.1338714084625,2.44249065417534E-15));
#13153=CARTESIAN_POINT('Ctrl Pts',(13.1033877505433,10.06515536275,2.02358146855792E-15));
#13154=CARTESIAN_POINT('Ctrl Pts',(13.1085900250014,9.99678230711821,1.45205686412796E-15));
#13155=CARTESIAN_POINT('Ctrl Pts',(13.1176922379213,9.92903302435398,1.04083408558608E-15));
#13156=CARTESIAN_POINT('Ctrl Pts',(13.1259450381762,9.86760606115364,6.67986352680291E-16));
#13157=CARTESIAN_POINT('Ctrl Pts',(13.1374044059322,9.80669148153412,4.49301831864335E-16));
#13158=CARTESIAN_POINT('Ctrl Pts',(13.152189704592,9.74651016097886,5.27355936696949E-16));
#13159=CARTESIAN_POINT('Ctrl Pts',(13.1696765010495,9.67533280248825,6.06618167751903E-16));
#13160=CARTESIAN_POINT('Ctrl Pts',(13.1918157822245,9.60517950813245,1.45195337725464E-15));
#13161=CARTESIAN_POINT('Ctrl Pts',(13.2183559139599,9.5363993371827,1.48492329543615E-15));
#13162=CARTESIAN_POINT('Ctrl Pts',(13.2242003063607,9.5212532816756,1.49218358868559E-15));
#13163=CARTESIAN_POINT('Ctrl Pts',(13.2302582723953,9.50617398307989,1.82761809169572E-15));
#13164=CARTESIAN_POINT('Ctrl Pts',(13.2365273868373,9.49116547782453,1.97064586870965E-15));
#13165=CARTESIAN_POINT('Ctrl Pts',(13.2429830702302,9.47571031920141,2.11793015476297E-15));
#13166=CARTESIAN_POINT('Ctrl Pts',(13.2496653021317,9.46032471587291,-4.47659329837229E-17));
#13167=CARTESIAN_POINT('Ctrl Pts',(13.2565571899036,9.44504393340732,8.32667268468867E-17));
#13168=CARTESIAN_POINT('Ctrl Pts',(13.2847562783215,9.38252055082999,6.07129623986592E-16));
#13169=CARTESIAN_POINT('Ctrl Pts',(13.316492584851,9.32166832971813,1.1675802761368E-15));
#13170=CARTESIAN_POINT('Ctrl Pts',(13.3515103647051,9.26274008818287,1.11022302462516E-15));
#13171=CARTESIAN_POINT('Ctrl Pts',(13.3865208536858,9.20382411579612,1.0528777151742E-15));
#13172=CARTESIAN_POINT('Ctrl Pts',(13.4248123241401,9.1468305524612,1.81328320611437E-15));
#13173=CARTESIAN_POINT('Ctrl Pts',(13.4661673690105,9.09204711620811,1.52655665885959E-15));
#13174=CARTESIAN_POINT('Ctrl Pts',(13.4961036636995,9.05239021106192,1.31899962583875E-15));
#13175=CARTESIAN_POINT('Ctrl Pts',(13.5276461316194,9.01389212746855,1.12431972020032E-15));
#13176=CARTESIAN_POINT('Ctrl Pts',(13.5607209276105,8.97667688443461,1.38777878078145E-15));
#13177=CARTESIAN_POINT('Ctrl Pts',(13.585527516553,8.94876489862573,1.58537699486414E-15));
#13178=CARTESIAN_POINT('Ctrl Pts',(13.6111962317832,8.92157478749522,9.51776285385933E-16));
#13179=CARTESIAN_POINT('Ctrl Pts',(13.637697633009,8.89516434107376,1.29757316003065E-15));
#13180=CARTESIAN_POINT('Ctrl Pts',(13.6465045264423,8.88638767356186,1.41248769600548E-15));
#13181=CARTESIAN_POINT('Ctrl Pts',(13.655396492531,8.87770402312783,3.58625279291791E-15));
#13182=CARTESIAN_POINT('Ctrl Pts',(13.6643718842665,8.86911537146476,3.39311911901063E-15));
#13183=CARTESIAN_POINT('Ctrl Pts',(13.7119765765409,8.82356191468833,2.3687550148941E-15));
#13184=CARTESIAN_POINT('Ctrl Pts',(13.7619291420876,8.78067465781436,8.91728926236411E-16));
#13185=CARTESIAN_POINT('Ctrl Pts',(13.8140393370137,8.7407331665078,1.15879528195251E-15));
#13186=CARTESIAN_POINT('Ctrl Pts',(13.8507161652704,8.71262106255111,1.34676515762891E-15));
#13187=CARTESIAN_POINT('Ctrl Pts',(13.8884623801383,8.68596907806574,4.57265468878883E-16));
#13188=CARTESIAN_POINT('Ctrl Pts',(13.9272161038781,8.66088946010809,6.21031004399697E-16));
#13189=CARTESIAN_POINT('Ctrl Pts',(13.9396522240711,8.65284137818927,6.73583577073472E-16));
#13190=CARTESIAN_POINT('Ctrl Pts',(13.9521938582917,8.64495425547895,-6.90481307027163E-16));
#13191=CARTESIAN_POINT('Ctrl Pts',(13.9648334399852,8.63723548509471,-4.78783679369599E-16));
#13192=CARTESIAN_POINT('Ctrl Pts',(14.0186777326348,8.60435372195212,4.23042764994196E-16));
#13193=CARTESIAN_POINT('Ctrl Pts',(14.0741898629058,8.57458852180253,1.67668390097511E-15));
#13194=CARTESIAN_POINT('Ctrl Pts',(14.1312020138798,8.54820924684521,9.10729824887824E-16));
#13195=CARTESIAN_POINT('Ctrl Pts',(14.1837968242759,8.52387385621248,2.04122396196814E-16));
#13196=CARTESIAN_POINT('Ctrl Pts',(14.237668785338,8.50242019207491,4.24437901475045E-16));
#13197=CARTESIAN_POINT('Ctrl Pts',(14.292691187472,8.48409882756164,7.38124839028131E-16));
#13198=CARTESIAN_POINT('Ctrl Pts',(14.3029515183617,8.48068234164015,8.02378731734645E-16));
#13199=CARTESIAN_POINT('Ctrl Pts',(14.3132518565374,8.47737489025808,-2.18489316463771E-17));
#13200=CARTESIAN_POINT('Ctrl Pts',(14.3235905172155,8.47417638326182,1.38777878078145E-17));
#13201=CARTESIAN_POINT('Ctrl Pts',(16.6117095221421,9.57816067485776,0.));
#13202=CARTESIAN_POINT('Ctrl Pts',(16.6342056260937,9.63593732993143,-5.64453285222628E-17));
#13203=CARTESIAN_POINT('Ctrl Pts',(16.6531279845489,9.69484386095271,2.56255980870842E-15));
#13204=CARTESIAN_POINT('Ctrl Pts',(16.6686273043538,9.75457005573485,2.22044604925031E-15));
#13205=CARTESIAN_POINT('Ctrl Pts',(16.6851480105456,9.8182321343534,1.85578740775209E-15));
#13206=CARTESIAN_POINT('Ctrl Pts',(16.6977802163463,9.88282599137373,2.5349006953864E-16));
#13207=CARTESIAN_POINT('Ctrl Pts',(16.7066567330792,9.94801273908534,1.0547118733939E-15));
#13208=CARTESIAN_POINT('Ctrl Pts',(16.7144236852204,10.005051143333,1.75578095176725E-15));
#13209=CARTESIAN_POINT('Ctrl Pts',(16.719314437616,10.0625444780201,6.09173409191634E-16));
#13210=CARTESIAN_POINT('Ctrl Pts',(16.7213853889065,10.1202806033607,2.22044604925031E-16));
#13211=CARTESIAN_POINT('Ctrl Pts',(16.722424837962,10.1492594408788,2.77374419265692E-17));
#13212=CARTESIAN_POINT('Ctrl Pts',(16.7227534366055,10.1782996069071,1.90884567343023E-15));
#13213=CARTESIAN_POINT('Ctrl Pts',(16.7223754026995,10.2073749211407,2.22044604925031E-15));
#13214=CARTESIAN_POINT('Ctrl Pts',(16.7222029883378,10.2206356410525,2.36256129089315E-15));
#13215=CARTESIAN_POINT('Ctrl Pts',(16.7218833791234,10.2339053875377,5.13100323005786E-16));
#13216=CARTESIAN_POINT('Ctrl Pts',(16.7214179597069,10.247160123306,5.27355936696949E-16));
#13217=CARTESIAN_POINT('Ctrl Pts',(16.7190673940356,10.3141021669321,5.99352838808771E-16));
#13218=CARTESIAN_POINT('Ctrl Pts',(16.7130012766232,10.3807814360522,-1.43723603342314E-15));
#13219=CARTESIAN_POINT('Ctrl Pts',(16.7033532632529,10.446865453063,-1.22124532708767E-15));
#13220=CARTESIAN_POINT('Ctrl Pts',(16.6935347267057,10.5141174676801,-1.00143710723863E-15));
#13221=CARTESIAN_POINT('Ctrl Pts',(16.6800066968994,10.5807540028731,2.94558620309747E-15));
#13222=CARTESIAN_POINT('Ctrl Pts',(16.6628587834113,10.6464404697601,3.63598040564739E-15));
#13223=CARTESIAN_POINT('Ctrl Pts',(16.6485155430073,10.7013834099898,4.21345532861642E-15));
#13224=CARTESIAN_POINT('Ctrl Pts',(16.6316387948011,10.7556622555645,8.18121107440506E-16));
#13225=CARTESIAN_POINT('Ctrl Pts',(16.6122532721583,10.8090814984855,4.44089209850063E-16));
#13226=CARTESIAN_POINT('Ctrl Pts',(16.6033171160797,10.8337061991522,2.71671500158053E-16));
#13227=CARTESIAN_POINT('Ctrl Pts',(16.5938475091728,10.8581481959351,1.39602086560423E-15));
#13228=CARTESIAN_POINT('Ctrl Pts',(16.5838450709829,10.8823879164002,1.41553435639707E-15));
#13229=CARTESIAN_POINT('Ctrl Pts',(16.5794865922092,10.8929501718345,1.42403719678521E-15));
#13230=CARTESIAN_POINT('Ctrl Pts',(16.5750269593375,10.9034737117046,1.48442318111539E-15));
#13231=CARTESIAN_POINT('Ctrl Pts',(16.570471999173,10.9139441680789,1.52655665885959E-15));
#13232=CARTESIAN_POINT('Ctrl Pts',(16.5424793917532,10.9782905869741,1.78548886883269E-15));
#13233=CARTESIAN_POINT('Ctrl Pts',(16.5108404898856,11.0407556838492,-1.7236150121703E-16));
#13234=CARTESIAN_POINT('Ctrl Pts',(16.4756621440164,11.100990873284,0.));
#13235=CARTESIAN_POINT('Ctrl Pts',(16.444207459148,11.1548501112569,1.54116874181183E-16));
#13236=CARTESIAN_POINT('Ctrl Pts',(16.409922248227,11.2069272492601,1.27367449426832E-15));
#13237=CARTESIAN_POINT('Ctrl Pts',(16.3728477619717,11.2569696466227,6.38378239159465E-16));
#13238=CARTESIAN_POINT('Ctrl Pts',(16.3324629238938,11.3114802904279,-5.21238641377393E-17));
#13239=CARTESIAN_POINT('Ctrl Pts',(16.2887690855124,11.3635778319471,2.57197908009856E-15));
#13240=CARTESIAN_POINT('Ctrl Pts',(16.2420801551,11.4131761610744,2.05391259555654E-15));
#13241=CARTESIAN_POINT('Ctrl Pts',(16.2240710321118,11.4323075140818,1.85408100905903E-15));
#13242=CARTESIAN_POINT('Ctrl Pts',(16.2056158080157,11.4510667408658,4.27898362178755E-16));
#13243=CARTESIAN_POINT('Ctrl Pts',(16.186730830448,11.4694477422767,1.38777878078145E-17));
#13244=CARTESIAN_POINT('Ctrl Pts',(16.1784451837245,11.4775122731223,-1.6777073166606E-16));
#13245=CARTESIAN_POINT('Ctrl Pts',(16.1700771698675,11.4855035107274,2.9199856936581E-15));
#13246=CARTESIAN_POINT('Ctrl Pts',(16.1616381587957,11.4934118833135,2.92821322744885E-15));
#13247=CARTESIAN_POINT('Ctrl Pts',(16.1106124187267,11.5412291643329,2.97796028869198E-15));
#13248=CARTESIAN_POINT('Ctrl Pts',(16.0569048507137,11.5861076850411,4.00406114414307E-15));
#13249=CARTESIAN_POINT('Ctrl Pts',(16.0008924066742,11.627985883466,3.77475828372553E-15));
#13250=CARTESIAN_POINT('Ctrl Pts',(15.9435800064801,11.6708360055897,3.54013368329494E-15));
#13251=CARTESIAN_POINT('Ctrl Pts',(15.8838538761052,11.7105455315968,2.16385081713861E-15));
#13252=CARTESIAN_POINT('Ctrl Pts',(15.8220688411562,11.7470208223532,1.04083408558608E-15));
#13253=CARTESIAN_POINT('Ctrl Pts',(15.7747993280594,11.7749267584029,1.81654283488492E-16));
#13254=CARTESIAN_POINT('Ctrl Pts',(15.726323581113,11.8009391230971,2.17035692847852E-15));
#13255=CARTESIAN_POINT('Ctrl Pts',(15.6767855539149,11.825002034133,1.99146255042137E-15));
#13256=CARTESIAN_POINT('Ctrl Pts',(15.6459597802179,11.839975538167,1.88014286480683E-15));
#13257=CARTESIAN_POINT('Ctrl Pts',(15.6147224394625,11.8541939368713,2.96650020135072E-15));
#13258=CARTESIAN_POINT('Ctrl Pts',(15.5831063371564,11.8676409930684,3.44169137633799E-15));
#13259=CARTESIAN_POINT('Ctrl Pts',(15.5653366958438,11.8751988306228,3.70876973573554E-15));
#13260=CARTESIAN_POINT('Ctrl Pts',(15.5474413401978,11.882515180091,1.95911521127522E-15));
#13261=CARTESIAN_POINT('Ctrl Pts',(15.5294587157909,11.8895744424011,1.99146255042137E-15));
#13262=CARTESIAN_POINT('Ctrl Pts',(15.4598207086011,11.916911551178,2.11672815042826E-15));
#13263=CARTESIAN_POINT('Ctrl Pts',(15.3888073670723,11.9404288078564,3.08329528087669E-15));
#13264=CARTESIAN_POINT('Ctrl Pts',(15.3167903740727,11.9600119575184,2.22044604925031E-15));
#13265=CARTESIAN_POINT('Ctrl Pts',(15.2629155692888,11.9746618105761,1.57496181038276E-15));
#13266=CARTESIAN_POINT('Ctrl Pts',(15.2084781337459,11.9871093369122,5.48219519405437E-16));
#13267=CARTESIAN_POINT('Ctrl Pts',(15.1536231199128,11.9972907920356,4.82253126321552E-16));
#13268=CARTESIAN_POINT('Ctrl Pts',(15.1365390543032,12.0004617081502,4.61708528686322E-16));
#13269=CARTESIAN_POINT('Ctrl Pts',(15.1194144359014,12.0034127175744,2.83080269845694E-15));
#13270=CARTESIAN_POINT('Ctrl Pts',(15.1022535287486,12.0061415889966,3.01147995429574E-15));
#13271=CARTESIAN_POINT('Ctrl Pts',(15.0856549463322,12.0087810413753,3.18623681855123E-15));
#13272=CARTESIAN_POINT('Ctrl Pts',(15.0690308581054,12.0112112791014,-3.4217463351498E-16));
#13273=CARTESIAN_POINT('Ctrl Pts',(15.0523912713646,12.0134301293824,-4.19803081186387E-16));
#13274=CARTESIAN_POINT('Ctrl Pts',(14.977715184966,12.0233880122238,-7.68188456112627E-16));
#13275=CARTESIAN_POINT('Ctrl Pts',(14.9026910556725,12.0290980438973,1.15979021628154E-15));
#13276=CARTESIAN_POINT('Ctrl Pts',(14.8276758656066,12.0304219755773,1.86656246015104E-15));
#13277=CARTESIAN_POINT('Ctrl Pts',(14.7702215268349,12.0314359784637,2.40788125035953E-15));
#13278=CARTESIAN_POINT('Ctrl Pts',(14.7127717290399,12.0298762775092,7.42876097831855E-16));
#13279=CARTESIAN_POINT('Ctrl Pts',(14.655480951399,12.0256608738343,-1.99493199737333E-17));
#13280=CARTESIAN_POINT('Ctrl Pts',(14.642235179624,12.0246862619105,-1.99785920673064E-16));
#13281=CARTESIAN_POINT('Ctrl Pts',(14.6289978976654,12.0235696114882,1.00718411817654E-15));
#13282=CARTESIAN_POINT('Ctrl Pts',(14.6157705619694,12.0223122647246,1.04083408558608E-15));
#13283=CARTESIAN_POINT('Origin',(15.,10.,9.54592528053767));
#13284=CARTESIAN_POINT('Ctrl Pts',(12.9434528818545,10.0014882284141,7.79592528053768));
#13285=CARTESIAN_POINT('Ctrl Pts',(12.9426313256354,10.0998548223026,7.79057696270225));
#13286=CARTESIAN_POINT('Ctrl Pts',(12.9937604030143,10.8787658748103,7.74818159569048));
#13287=CARTESIAN_POINT('Ctrl Pts',(13.989390948843,12.2086082123096,7.66873917950236));
#13288=CARTESIAN_POINT('Ctrl Pts',(16.3073490337982,12.0466292797422,7.55759803197335));
#13289=CARTESIAN_POINT('Ctrl Pts',(17.4286195856453,10.0116469634969,7.44645688444433));
#13290=CARTESIAN_POINT('Ctrl Pts',(16.3268236193488,7.9657970755479,7.33531573691531));
#13291=CARTESIAN_POINT('Ctrl Pts',(14.0105079180419,7.78208259180166,7.22417458938629));
#13292=CARTESIAN_POINT('Ctrl Pts',(12.9977472036765,9.10777343312236,7.14437777059375));
#13293=CARTESIAN_POINT('Ctrl Pts',(12.9427343174564,9.89346179907822,7.10162800097754));
#13294=CARTESIAN_POINT('Ctrl Pts',(12.9436341942584,9.99839713117394,7.09592528053768));
#13295=CARTESIAN_POINT('Ctrl Pts',(12.9473113968994,9.99752941021421,7.85407471946233));
#13296=CARTESIAN_POINT('Ctrl Pts',(12.9508756442256,10.4678337643571,7.82862238128887));
#13297=CARTESIAN_POINT('Ctrl Pts',(13.3435591556684,11.6297989150585,7.76612299393907));
#13298=CARTESIAN_POINT('Ctrl Pts',(15.2723377259255,12.4126882042673,7.66657655741295));
#13299=CARTESIAN_POINT('Ctrl Pts',(17.1748665662283,11.0807510628696,7.55543540988391));
#13300=CARTESIAN_POINT('Ctrl Pts',(17.0874397300721,8.75827685188236,7.44429426235491));
#13301=CARTESIAN_POINT('Ctrl Pts',(15.0888245216199,7.57307606901691,7.33315311482588));
#13302=CARTESIAN_POINT('Ctrl Pts',(13.2786046599163,8.4748124919398,7.23641326719502));
#13303=CARTESIAN_POINT('Ctrl Pts',(12.9501053395568,9.58221924013019,7.1767204687405));
#13304=CARTESIAN_POINT('Ctrl Pts',(12.9479405474349,10.0011587877502,7.15407471946232));
#13305=CARTESIAN_POINT('Ctrl Pts',(16.2690708798524,11.0793586530485,8.));
#13306=CARTESIAN_POINT('Ctrl Pts',(16.6279938291456,10.657350026192,7.96295295082366));
#13307=CARTESIAN_POINT('Ctrl Pts',(16.8854598801969,9.43433251832768,7.88885885247098));
#13308=CARTESIAN_POINT('Ctrl Pts',(15.5448845996416,8.10642602073482,7.77771770494196));
#13309=CARTESIAN_POINT('Ctrl Pts',(13.7057107168279,8.51663622362914,7.66657655741294));
#13310=CARTESIAN_POINT('Ctrl Pts',(13.0512228488578,10.282272228723,7.55543540988393));
#13311=CARTESIAN_POINT('Ctrl Pts',(14.1805939023105,11.7907488899904,7.4442942623549));
#13312=CARTESIAN_POINT('Ctrl Pts',(16.0600041320393,11.6594156856311,7.33315311482588));
#13313=CARTESIAN_POINT('Ctrl Pts',(16.9691350430393,10.0094434073176,7.22201196729686));
#13314=CARTESIAN_POINT('Ctrl Pts',(16.075794208461,8.35065965585243,7.11087081976784));
#13315=CARTESIAN_POINT('Ctrl Pts',(14.1977156303481,8.20170317456703,6.99972967223882));
#13316=CARTESIAN_POINT('Ctrl Pts',(13.0540155464189,9.69879197844384,6.8885885247098));
#13317=CARTESIAN_POINT('Ctrl Pts',(13.6915931588825,11.4716176684,6.77744737718079));
#13318=CARTESIAN_POINT('Ctrl Pts',(15.5268344256012,11.8973708763893,6.66630622965175));
#13319=CARTESIAN_POINT('Ctrl Pts',(16.8798324113308,10.5863519109992,6.55516508212275));
#13320=CARTESIAN_POINT('Ctrl Pts',(16.5121060647823,8.73860643490976,6.44402393459371));
#13321=CARTESIAN_POINT('Ctrl Pts',(14.7602576417037,8.04549238469812,6.33288278706472));
#13322=CARTESIAN_POINT('Ctrl Pts',(13.2278598780647,9.14145649340251,6.22174163953567));
#13323=CARTESIAN_POINT('Ctrl Pts',(13.3176091277843,11.0232978176747,6.11060049200667));
#13324=CARTESIAN_POINT('Ctrl Pts',(14.9473524627353,11.9684525532754,5.99945934447763));
#13325=CARTESIAN_POINT('Ctrl Pts',(16.6252872741601,11.1117637611562,5.88831819694864));
#13326=CARTESIAN_POINT('Ctrl Pts',(16.8154983706705,9.23741031714155,5.7771770494196));
#13327=CARTESIAN_POINT('Ctrl Pts',(15.3438740364888,8.06110134986314,5.66603590189059));
#13328=CARTESIAN_POINT('Ctrl Pts',(13.5574810043252,8.65958353517834,5.55489475436156));
#13329=CARTESIAN_POINT('Ctrl Pts',(13.091512829808,10.4850299660946,5.44375360683254));
#13330=CARTESIAN_POINT('Ctrl Pts',(14.372498357211,11.866499137894,5.33261245930353));
#13331=CARTESIAN_POINT('Ctrl Pts',(16.2278740796803,11.5394487945932,5.22147131177451));
#13332=CARTESIAN_POINT('Ctrl Pts',(16.9593024145856,9.80324788695935,5.11033016424548));
#13333=CARTESIAN_POINT('Ctrl Pts',(15.8972627818015,8.24714608542604,4.99918901671647));
#13334=CARTESIAN_POINT('Ctrl Pts',(14.0139042725623,8.29553745649413,4.88804786918744));
#13335=CARTESIAN_POINT('Ctrl Pts',(13.0331788061281,9.90412645273168,4.77690672165843));
#13336=CARTESIAN_POINT('Ctrl Pts',(13.852803700691,11.6004743036209,4.6657655741294));
#13337=CARTESIAN_POINT('Ctrl Pts',(15.7225267323057,11.8318112530665,4.55462442660039));
#13338=CARTESIAN_POINT('Ctrl Pts',(16.9308773588479,10.3863806035781,4.44348327907136));
#13339=CARTESIAN_POINT('Ctrl Pts',(16.3717791899039,8.58727242545577,4.33234213154234));
#13340=CARTESIAN_POINT('Ctrl Pts',(14.557008584925,8.08131921573479,4.22120098401333));
#13341=CARTESIAN_POINT('Ctrl Pts',(13.1477348072808,9.33165053933164,4.1100598364843));
#13342=CARTESIAN_POINT('Ctrl Pts',(13.4339513562445,11.1937625354845,3.99891868895529));
#13343=CARTESIAN_POINT('Ctrl Pts',(15.1536669186984,11.9631515030262,3.88777754142627));
#13344=CARTESIAN_POINT('Ctrl Pts',(16.7327218591219,10.9355491994844,3.77663639389724));
#13345=CARTESIAN_POINT('Ctrl Pts',(16.72571171427,9.0515821464321,3.66549524636823));
#13346=CARTESIAN_POINT('Ctrl Pts',(15.1390532935877,8.03575930006501,3.5543540988392));
#13347=CARTESIAN_POINT('Ctrl Pts',(13.4251109855405,8.81792473257162,3.44321295131019));
#13348=CARTESIAN_POINT('Ctrl Pts',(13.1527598168138,10.6821151305718,3.33207180378117));
#13349=CARTESIAN_POINT('Ctrl Pts',(14.5712992796378,11.9219243060325,3.22093065625215));
#13350=CARTESIAN_POINT('Ctrl Pts',(16.3822544328478,11.4024799565668,3.10978950872313));
#13351=CARTESIAN_POINT('Ctrl Pts',(16.9279485267848,9.5992609030834,2.99864836119411));
#13352=CARTESIAN_POINT('Ctrl Pts',(15.7088747623015,8.1628625752935,2.88750721366509));
#13353=CARTESIAN_POINT('Ctrl Pts',(13.8409250663671,8.40810721351364,2.77636606613607));
#13354=CARTESIAN_POINT('Ctrl Pts',(13.0339467396719,10.1105075714153,2.66522491860705));
#13355=CARTESIAN_POINT('Ctrl Pts',(14.0266158380486,11.7117536680222,2.55408377107803));
#13356=CARTESIAN_POINT('Ctrl Pts',(15.9102823145912,11.7461281313822,2.44294262354901));
#13357=CARTESIAN_POINT('Ctrl Pts',(16.9607123494012,10.182165940018,2.33180147601999));
#13358=CARTESIAN_POINT('Ctrl Pts',(16.2163838173521,8.45145624507036,2.22066032849097));
#13359=CARTESIAN_POINT('Ctrl Pts',(14.3586256307264,8.13822228853373,2.10951918096195));
#13360=CARTESIAN_POINT('Ctrl Pts',(13.0879561823328,9.52918602651344,1.99837803343293));
#13361=CARTESIAN_POINT('Ctrl Pts',(13.567496054586,11.3511142921827,1.88723688590391));
#13362=CARTESIAN_POINT('Ctrl Pts',(15.3582933952052,11.9362858933093,1.77609573837489));
#13363=CARTESIAN_POINT('Ctrl Pts',(16.8211231428988,10.7490580544729,1.66495459084587));
#13364=CARTESIAN_POINT('Ctrl Pts',(16.6169687348735,8.87617186592661,1.55381344331685));
#13365=CARTESIAN_POINT('Ctrl Pts',(14.9327051338352,8.0319939487841,1.44267229578783));
#13366=CARTESIAN_POINT('Ctrl Pts',(13.3100404788966,8.98925013270617,1.33153114825881));
#13367=CARTESIAN_POINT('Ctrl Pts',(13.2342981763212,10.8717083962423,1.22039000072979));
#13368=CARTESIAN_POINT('Ctrl Pts',(14.7748090869154,11.9562361327899,1.10924885320077));
#13369=CARTESIAN_POINT('Ctrl Pts',(16.5214516854989,11.2501087122817,0.99810770567175));
#13370=CARTESIAN_POINT('Ctrl Pts',(16.875415955447,9.39966945781174,0.886966558142732));
#13371=CARTESIAN_POINT('Ctrl Pts',(15.5127017221989,8.09877181111676,0.775825410613711));
#13372=CARTESIAN_POINT('Ctrl Pts',(13.6806745613723,8.53813915273012,0.664684263084692));
#13373=CARTESIAN_POINT('Ctrl Pts',(13.0563174575166,10.3157216649401,0.553543115555672));
#13374=CARTESIAN_POINT('Ctrl Pts',(14.2111078058336,11.8041392084987,0.442401968026652));
#13375=CARTESIAN_POINT('Ctrl Pts',(16.0880628853469,11.6414405555679,0.331260820497632));
#13376=CARTESIAN_POINT('Ctrl Pts',(16.9689629398242,9.97560865889059,0.220119672968611));
#13377=CARTESIAN_POINT('Ctrl Pts',(16.0477171708735,8.33331419534448,0.108978525439592));
#13378=CARTESIAN_POINT('Ctrl Pts',(14.167115703941,8.21427174764607,-0.00216262208942877));
#13379=CARTESIAN_POINT('Ctrl Pts',(13.0494874512438,9.73459567298507,-0.113303769618448));
#13380=CARTESIAN_POINT('Ctrl Pts',(13.4941166421103,10.9026562341787,-0.187397867971127));
#13381=CARTESIAN_POINT('Ctrl Pts',(13.9143317362933,11.2636773406136,-0.224444917147467));
#13382=CARTESIAN_POINT('Ctrl Pts',(16.3677806246588,11.1633123698097,8.07481497238249));
#13383=CARTESIAN_POINT('Ctrl Pts',(16.7546210002301,10.7084794424949,8.03776792320615));
#13384=CARTESIAN_POINT('Ctrl Pts',(17.032113047149,9.39033427232925,7.96367382485347));
#13385=CARTESIAN_POINT('Ctrl Pts',(15.5872663299559,7.95914173013072,7.85253267732445));
#13386=CARTESIAN_POINT('Ctrl Pts',(13.6050394565572,8.40125853894243,7.74139152979544));
#13387=CARTESIAN_POINT('Ctrl Pts',(12.8996447941346,10.3042276766854,7.6302503822664));
#13388=CARTESIAN_POINT('Ctrl Pts',(14.116859584488,11.9300353307635,7.5191092347374));
#13389=CARTESIAN_POINT('Ctrl Pts',(16.1424524326256,11.7884868836682,7.40796808720837));
#13390=CARTESIAN_POINT('Ctrl Pts',(17.1222965572413,10.010177926044,7.29682693967936));
#13391=CARTESIAN_POINT('Ctrl Pts',(16.1594706787569,8.22237212908425,7.18568579215033));
#13392=CARTESIAN_POINT('Ctrl Pts',(14.1353130595794,8.06182964697857,7.07454464462131));
#13393=CARTESIAN_POINT('Ctrl Pts',(12.9026547108187,9.67536368344986,6.9634034970923));
#13394=CARTESIAN_POINT('Ctrl Pts',(13.5898238192497,11.5860817277419,6.85226234956327));
#13395=CARTESIAN_POINT('Ctrl Pts',(15.5678121932987,12.0449504938755,6.74112120203425));
#13396=CARTESIAN_POINT('Ctrl Pts',(17.0260478674942,10.6319590149209,6.62998005450523));
#13397=CARTESIAN_POINT('Ctrl Pts',(16.6297193566359,8.64049384018613,6.51883890697621));
#13398=CARTESIAN_POINT('Ctrl Pts',(14.7416102143752,7.89346860809774,6.4076977594472));
#13399=CARTESIAN_POINT('Ctrl Pts',(13.0900208479722,9.07467802437696,6.29655661191817));
#13400=CARTESIAN_POINT('Ctrl Pts',(13.1867508941761,11.102891060296,6.18541546438915));
#13401=CARTESIAN_POINT('Ctrl Pts',(14.9432574787194,12.1215609826643,6.07427431686013));
#13402=CARTESIAN_POINT('Ctrl Pts',(16.7517039263869,11.1982379832749,5.96313316933111));
#13403=CARTESIAN_POINT('Ctrl Pts',(16.9567098535833,9.17809524326976,5.8519920218021));
#13404=CARTESIAN_POINT('Ctrl Pts',(15.3706209415879,7.91029165593742,5.74085087427306));
#13405=CARTESIAN_POINT('Ctrl Pts',(13.4452802721186,8.55532445140494,5.62970972674406));
#13406=CARTESIAN_POINT('Ctrl Pts',(12.9430685746236,10.5227561364266,5.51856857921503));
#13407=CARTESIAN_POINT('Ctrl Pts',(14.3236905813738,12.0116775172169,5.40742743168601));
#13408=CARTESIAN_POINT('Ctrl Pts',(16.3233794915402,11.6591888343887,5.296286284157));
#13409=CARTESIAN_POINT('Ctrl Pts',(17.1116991360081,9.78794428873115,5.18514513662797));
#13410=CARTESIAN_POINT('Ctrl Pts',(15.9670528791255,8.11080715799694,5.07400398909896));
#13411=CARTESIAN_POINT('Ctrl Pts',(13.937204649905,8.16296246373945,4.96286284156993));
#13412=CARTESIAN_POINT('Ctrl Pts',(12.8801972656884,9.89666930157111,4.85172169404092));
#13413=CARTESIAN_POINT('Ctrl Pts',(13.763573496338,11.7249609753961,4.74058054651189));
#13414=CARTESIAN_POINT('Ctrl Pts',(15.7787256653157,11.9742915701193,4.62943939898287));
#13415=CARTESIAN_POINT('Ctrl Pts',(17.0810631478139,10.4164337167515,4.51829825145386));
#13416=CARTESIAN_POINT('Ctrl Pts',(16.4784777013235,8.47738890312604,4.40715710392483));
#13417=CARTESIAN_POINT('Ctrl Pts',(14.5225522198569,7.93208208990784,4.29601595639582));
#13418=CARTESIAN_POINT('Ctrl Pts',(13.003663560048,9.27966557477885,4.18487480886679));
#13419=CARTESIAN_POINT('Ctrl Pts',(13.3121423505903,11.2866147134897,4.07373366133777));
#13420=CARTESIAN_POINT('Ctrl Pts',(15.1656193025807,12.1158476108296,3.96259251380876));
#13421=CARTESIAN_POINT('Ctrl Pts',(16.8674948928822,11.0083172569673,3.85145136627974));
#13422=CARTESIAN_POINT('Ctrl Pts',(16.8599394911652,8.97781315071892,3.74031021875072));
#13423=CARTESIAN_POINT('Ctrl Pts',(15.1498690134521,7.88297847331436,3.6291690712217));
#13424=CARTESIAN_POINT('Ctrl Pts',(13.3026143660185,8.72598160327735,3.51802792369268));
#13425=CARTESIAN_POINT('Ctrl Pts',(13.0090794204125,10.7351708042433,3.40688677616366));
#13426=CARTESIAN_POINT('Ctrl Pts',(14.5379544607021,12.0714137165907,3.29574562863464));
#13427=CARTESIAN_POINT('Ctrl Pts',(16.4897677203167,11.5115664077704,3.18460448110562));
#13428=CARTESIAN_POINT('Ctrl Pts',(17.0779065079348,9.56809097032502,3.0734633335766));
#13429=CARTESIAN_POINT('Ctrl Pts',(15.7640118298975,8.01996798268554,2.96232218604758));
#13430=CARTESIAN_POINT('Ctrl Pts',(13.750770928622,8.28428802168758,2.85118103851856));
#13431=CARTESIAN_POINT('Ctrl Pts',(12.8810249299575,10.1191029732536,2.74003989098954));
#13432=CARTESIAN_POINT('Ctrl Pts',(13.9509049350957,11.8448957725527,2.62889874346052));
#13433=CARTESIAN_POINT('Ctrl Pts',(15.9810850856591,11.8819439199126,2.5177575959315));
#13434=CARTESIAN_POINT('Ctrl Pts',(17.1132187371223,10.1963350094821,2.40661644840248));
#13435=CARTESIAN_POINT('Ctrl Pts',(16.3109955038258,8.33100878914221,2.29547530087346));
#13436=CARTESIAN_POINT('Ctrl Pts',(14.3087388187906,7.99341114701062,2.18433415334444));
#13437=CARTESIAN_POINT('Ctrl Pts',(12.9392352871511,9.49256559190101,2.07319300581542));
#13438=CARTESIAN_POINT('Ctrl Pts',(13.4560743041299,11.4562054648689,1.9620518582864));
#13439=CARTESIAN_POINT('Ctrl Pts',(15.3861618540659,12.0868923641024,1.85091071075738));
#13440=CARTESIAN_POINT('Ctrl Pts',(16.9627721268528,10.8073206232357,1.73976956322836));
#13441=CARTESIAN_POINT('Ctrl Pts',(16.7427383618607,8.78875926346142,1.62862841569934));
#13442=CARTESIAN_POINT('Ctrl Pts',(14.927470864283,7.87892024882208,1.51748726817032));
#13443=CARTESIAN_POINT('Ctrl Pts',(13.1785935473582,8.91063288362445,1.4063461206413));
#13444=CARTESIAN_POINT('Ctrl Pts',(13.0969599242293,10.9395108450296,1.29520497311228));
#13445=CARTESIAN_POINT('Ctrl Pts',(14.7572934871832,12.1083943554034,1.18406382558326));
#13446=CARTESIAN_POINT('Ctrl Pts',(16.6397918901283,11.3473435586001,1.07292267805424));
#13447=CARTESIAN_POINT('Ctrl Pts',(17.0212878947587,9.35297508040565,0.961781530525221));
#13448=CARTESIAN_POINT('Ctrl Pts',(15.552580232504,7.95089216757367,0.8506403829962));
#13449=CARTESIAN_POINT('Ctrl Pts',(13.5780559610789,8.42443398978971,0.739499235467181));
#13450=CARTESIAN_POINT('Ctrl Pts',(12.9051356671224,10.3402788472622,0.62835808793816));
#13451=CARTESIAN_POINT('Ctrl Pts',(14.1497468933721,11.9444671631413,0.517216940409142));
#13452=CARTESIAN_POINT('Ctrl Pts',(16.1726936269793,11.7691136279923,0.40607579288012));
#13453=CARTESIAN_POINT('Ctrl Pts',(17.1221110676466,9.97371147324507,0.2949346453511));
#13454=CARTESIAN_POINT('Ctrl Pts',(16.1292097779517,8.20367751936212,0.183793497822081));
#13455=CARTESIAN_POINT('Ctrl Pts',(14.1023330368556,8.07537581765355,0.0726523502930604));
#13456=CARTESIAN_POINT('Ctrl Pts',(12.8977744153637,9.71395222918213,-0.0384887972359591));
#13457=CARTESIAN_POINT('Ctrl Pts',(13.3769873593213,10.9728658402285,-0.112582895588638));
#13458=CARTESIAN_POINT('Ctrl Pts',(13.829887250996,11.361967569938,-0.149629944764978));
#13459=CARTESIAN_POINT('Ctrl Pts',(16.4664903694653,11.247266086571,8.14962994476498));
#13460=CARTESIAN_POINT('Ctrl Pts',(16.8812481713146,10.7596088587978,8.11258289558864));
#13461=CARTESIAN_POINT('Ctrl Pts',(17.1787662141011,9.34633602633083,8.03848879723595));
#13462=CARTESIAN_POINT('Ctrl Pts',(15.6296480602701,7.81185743952661,7.92734764970694));
#13463=CARTESIAN_POINT('Ctrl Pts',(13.5043681962864,8.28588085425572,7.81620650217792));
#13464=CARTESIAN_POINT('Ctrl Pts',(12.7480667394114,10.3261831246478,7.7050653546489));
#13465=CARTESIAN_POINT('Ctrl Pts',(14.0531252666655,12.0693217715365,7.59392420711989));
#13466=CARTESIAN_POINT('Ctrl Pts',(16.2249007332119,11.9175580817052,7.48278305959085));
#13467=CARTESIAN_POINT('Ctrl Pts',(17.2754580714433,10.0109124447704,7.37164191206185));
#13468=CARTESIAN_POINT('Ctrl Pts',(16.2431471490529,8.09408460231609,7.26050076453282));
#13469=CARTESIAN_POINT('Ctrl Pts',(14.0729104888107,7.92195611939011,7.1493596170038));
#13470=CARTESIAN_POINT('Ctrl Pts',(12.7512938752185,9.65193538845589,7.03821846947478));
#13471=CARTESIAN_POINT('Ctrl Pts',(13.488054479617,11.7005457870837,6.92707732194576));
#13472=CARTESIAN_POINT('Ctrl Pts',(15.6087899609963,12.1925301113618,6.81593617441674));
#13473=CARTESIAN_POINT('Ctrl Pts',(17.1722633236576,10.6775661188427,6.70479502688772));
#13474=CARTESIAN_POINT('Ctrl Pts',(16.7473326484895,8.54238124546246,6.5936538793587));
#13475=CARTESIAN_POINT('Ctrl Pts',(14.7229627870467,7.7414448314974,6.48251273182969));
#13476=CARTESIAN_POINT('Ctrl Pts',(12.9521818178798,9.00789955535137,6.37137158430065));
#13477=CARTESIAN_POINT('Ctrl Pts',(13.0558926605679,11.1824843029172,6.26023043677165));
#13478=CARTESIAN_POINT('Ctrl Pts',(14.9391624947034,12.2746694120531,6.14908928924261));
#13479=CARTESIAN_POINT('Ctrl Pts',(16.8781205786138,11.2847122053937,6.03794814171361));
#13480=CARTESIAN_POINT('Ctrl Pts',(17.0979213364961,9.11878016939794,5.92680699418458));
#13481=CARTESIAN_POINT('Ctrl Pts',(15.3973678466869,7.75948196201174,5.81566584665556));
#13482=CARTESIAN_POINT('Ctrl Pts',(13.333079539912,8.45106536763152,5.70452469912655));
#13483=CARTESIAN_POINT('Ctrl Pts',(12.794624319439,10.5604823067586,5.59338355159752));
#13484=CARTESIAN_POINT('Ctrl Pts',(14.2748828055367,12.1568558965399,5.4822424040685));
#13485=CARTESIAN_POINT('Ctrl Pts',(16.4188849034001,11.7789288741843,5.37110125653949));
#13486=CARTESIAN_POINT('Ctrl Pts',(17.2640958574308,9.77264069050295,5.25996010901046));
#13487=CARTESIAN_POINT('Ctrl Pts',(16.0368429764495,7.97446823056785,5.14881896148145));
#13488=CARTESIAN_POINT('Ctrl Pts',(13.8605050272477,8.03038747098476,5.03767781395242));
#13489=CARTESIAN_POINT('Ctrl Pts',(12.7272157252487,9.88921215041053,4.92653666642341));
#13490=CARTESIAN_POINT('Ctrl Pts',(13.6743432919849,11.8494476471713,4.81539551889438));
#13491=CARTESIAN_POINT('Ctrl Pts',(15.8349245983256,12.116771887172,4.70425437136536));
#13492=CARTESIAN_POINT('Ctrl Pts',(17.23124893678,10.446486829925,4.59311322383634));
#13493=CARTESIAN_POINT('Ctrl Pts',(16.5851762127431,8.36750538079628,4.48197207630733));
#13494=CARTESIAN_POINT('Ctrl Pts',(14.4880958547888,7.78284496408089,4.3708309287783));
#13495=CARTESIAN_POINT('Ctrl Pts',(12.8595923128151,9.22768061022607,4.25968978124929));
#13496=CARTESIAN_POINT('Ctrl Pts',(13.190333344936,11.3794668914948,4.14854863372026));
#13497=CARTESIAN_POINT('Ctrl Pts',(15.177571686463,12.268543718633,4.03740748619125));
#13498=CARTESIAN_POINT('Ctrl Pts',(17.0022679266424,11.0810853144502,3.92626633866222));
#13499=CARTESIAN_POINT('Ctrl Pts',(16.9941672680604,8.90404415500574,3.81512519113321));
#13500=CARTESIAN_POINT('Ctrl Pts',(15.1606847333165,7.73019764656371,3.70398404360418));
#13501=CARTESIAN_POINT('Ctrl Pts',(13.1801177464964,8.63403847398308,3.59284289607517));
#13502=CARTESIAN_POINT('Ctrl Pts',(12.8653990240112,10.7882264779147,3.48170174854614));
#13503=CARTESIAN_POINT('Ctrl Pts',(14.5046096417664,12.220903127149,3.37056060101713));
#13504=CARTESIAN_POINT('Ctrl Pts',(16.5972810077856,11.620652858974,3.2594194534881));
#13505=CARTESIAN_POINT('Ctrl Pts',(17.2278644890848,9.53692103756665,3.14827830595909));
#13506=CARTESIAN_POINT('Ctrl Pts',(15.8191488974935,7.87707339007757,3.03713715843007));
#13507=CARTESIAN_POINT('Ctrl Pts',(13.660616790877,8.16046882986155,2.92599601090105));
#13508=CARTESIAN_POINT('Ctrl Pts',(12.7281031202431,10.1276983750918,2.81485486337203));
#13509=CARTESIAN_POINT('Ctrl Pts',(13.8751940321428,11.9780378770833,2.703713715843));
#13510=CARTESIAN_POINT('Ctrl Pts',(16.051887856727,12.017759708443,2.59257256831399));
#13511=CARTESIAN_POINT('Ctrl Pts',(17.2657251248433,10.2105040789463,2.48143142078496));
#13512=CARTESIAN_POINT('Ctrl Pts',(16.4056071902996,8.21056133321405,2.37029027325595));
#13513=CARTESIAN_POINT('Ctrl Pts',(14.2588520068548,7.84860000548751,2.25914912572693));
#13514=CARTESIAN_POINT('Ctrl Pts',(12.7905143919695,9.45594515728858,2.14800797819791));
#13515=CARTESIAN_POINT('Ctrl Pts',(13.3446525536738,11.5612966375552,2.03686683066889));
#13516=CARTESIAN_POINT('Ctrl Pts',(15.4140303129267,12.2374988348955,1.92572568313987));
#13517=CARTESIAN_POINT('Ctrl Pts',(17.1044211108068,10.8655831919985,1.81458453561085));
#13518=CARTESIAN_POINT('Ctrl Pts',(16.868507988848,8.70134666099622,1.70344338808183));
#13519=CARTESIAN_POINT('Ctrl Pts',(14.9222365947309,7.72584654886007,1.59230224055281));
#13520=CARTESIAN_POINT('Ctrl Pts',(13.0471466158198,8.83201563454272,1.48116109302379));
#13521=CARTESIAN_POINT('Ctrl Pts',(12.9596216721374,11.007313293817,1.37001994549477));
#13522=CARTESIAN_POINT('Ctrl Pts',(14.7397778874509,12.2605525780168,1.25887879796575));
#13523=CARTESIAN_POINT('Ctrl Pts',(16.7581320947577,11.4445784049186,1.14773765043673));
#13524=CARTESIAN_POINT('Ctrl Pts',(17.1671598340705,9.30628070299953,1.03659650290771));
#13525=CARTESIAN_POINT('Ctrl Pts',(15.5924587428091,7.80301252403059,0.925455355378689));
#13526=CARTESIAN_POINT('Ctrl Pts',(13.4754373607854,8.3107288268493,0.81431420784967));
#13527=CARTESIAN_POINT('Ctrl Pts',(12.7539538767281,10.3648360295842,0.703173060320649));
#13528=CARTESIAN_POINT('Ctrl Pts',(14.0883859809107,12.084795117784,0.592031912791631));
#13529=CARTESIAN_POINT('Ctrl Pts',(16.2573243686117,11.8967867004167,0.480890765262609));
#13530=CARTESIAN_POINT('Ctrl Pts',(17.2752591954691,9.97181428759956,0.36974961773359));
#13531=CARTESIAN_POINT('Ctrl Pts',(16.21070238503,8.07404084337976,0.25860847020457));
#13532=CARTESIAN_POINT('Ctrl Pts',(14.0375503697701,7.93647988766104,0.147467322675549));
#13533=CARTESIAN_POINT('Ctrl Pts',(12.7460613794835,9.6933087853792,0.03632617514653));
#13534=CARTESIAN_POINT('Ctrl Pts',(13.2598580765322,11.0430754462783,-0.0377679232061492));
#13535=CARTESIAN_POINT('Ctrl Pts',(13.7454427656987,11.4602577992624,-0.0748149723824891));
#13536=CARTESIAN_POINT('Ctrl Pts',(16.5652001142717,11.3312198033322,8.22444491714747));
#13537=CARTESIAN_POINT('Ctrl Pts',(17.0078753423991,10.8107382751008,8.18739786797113));
#13538=CARTESIAN_POINT('Ctrl Pts',(17.3254193810532,9.3023377803324,8.11330376961845));
#13539=CARTESIAN_POINT('Ctrl Pts',(15.6720297905844,7.66457314892251,8.00216262208943));
#13540=CARTESIAN_POINT('Ctrl Pts',(13.4036969360157,8.170503169569,7.89102147456041));
#13541=CARTESIAN_POINT('Ctrl Pts',(12.5964886846882,10.3481385726101,7.77988032703139));
#13542=CARTESIAN_POINT('Ctrl Pts',(13.989390948843,12.2086082123096,7.66873917950236));
#13543=CARTESIAN_POINT('Ctrl Pts',(16.3073490337982,12.0466292797422,7.55759803197335));
#13544=CARTESIAN_POINT('Ctrl Pts',(17.4286195856453,10.0116469634969,7.44645688444433));
#13545=CARTESIAN_POINT('Ctrl Pts',(16.3268236193488,7.9657970755479,7.33531573691531));
#13546=CARTESIAN_POINT('Ctrl Pts',(14.0105079180419,7.78208259180166,7.22417458938629));
#13547=CARTESIAN_POINT('Ctrl Pts',(12.5999330396184,9.6285070934619,7.11303344185727));
#13548=CARTESIAN_POINT('Ctrl Pts',(13.3862851399842,11.8150098464255,7.00189229432825));
#13549=CARTESIAN_POINT('Ctrl Pts',(15.6497677286939,12.3401097288481,6.89075114679923));
#13550=CARTESIAN_POINT('Ctrl Pts',(17.3184787798211,10.7231732227644,6.77960999927021));
#13551=CARTESIAN_POINT('Ctrl Pts',(16.864945940343,8.44426865073882,6.66846885174118));
#13552=CARTESIAN_POINT('Ctrl Pts',(14.7043153597183,7.58942105489702,6.55732770421218));
#13553=CARTESIAN_POINT('Ctrl Pts',(12.8143427877872,8.94112108632582,6.44618655668314));
#13554=CARTESIAN_POINT('Ctrl Pts',(12.9250344269597,11.2620775455385,6.33504540915413));
#13555=CARTESIAN_POINT('Ctrl Pts',(14.9350675106875,12.4277778414421,6.22390426162511));
#13556=CARTESIAN_POINT('Ctrl Pts',(17.0045372308406,11.3711864275124,6.1127631140961));
#13557=CARTESIAN_POINT('Ctrl Pts',(17.2391328194089,9.05946509552617,6.00162196656707));
#13558=CARTESIAN_POINT('Ctrl Pts',(15.424114751786,7.608672268086,5.89048081903805));
#13559=CARTESIAN_POINT('Ctrl Pts',(13.2208788077054,8.34680628385815,5.77933967150903));
#13560=CARTESIAN_POINT('Ctrl Pts',(12.6461800642546,10.5982084770906,5.66819852398001));
#13561=CARTESIAN_POINT('Ctrl Pts',(14.2260750296995,12.3020342758629,5.55705737645099));
#13562=CARTESIAN_POINT('Ctrl Pts',(16.51439031526,11.8986689139798,5.44591622892198));
#13563=CARTESIAN_POINT('Ctrl Pts',(17.4164925788533,9.75733709227475,5.33477508139295));
#13564=CARTESIAN_POINT('Ctrl Pts',(16.1066330737735,7.83812930313874,5.22363393386394));
#13565=CARTESIAN_POINT('Ctrl Pts',(13.7838054045903,7.89781247823008,5.11249278633491));
#13566=CARTESIAN_POINT('Ctrl Pts',(12.574234184809,9.88175499924995,5.0013516388059));
#13567=CARTESIAN_POINT('Ctrl Pts',(13.5851130876319,11.9739343189466,4.89021049127687));
#13568=CARTESIAN_POINT('Ctrl Pts',(15.8911235313356,12.2592522042247,4.77906934374785));
#13569=CARTESIAN_POINT('Ctrl Pts',(17.381434725746,10.4765399430985,4.66792819621883));
#13570=CARTESIAN_POINT('Ctrl Pts',(16.6918747241627,8.25762185846654,4.55678704868982));
#13571=CARTESIAN_POINT('Ctrl Pts',(14.4536394897207,7.63360783825394,4.44564590116079));
#13572=CARTESIAN_POINT('Ctrl Pts',(12.7155210655824,9.17569564567328,4.33450475363177));
#13573=CARTESIAN_POINT('Ctrl Pts',(13.0685243392818,11.4723190694999,4.22336360610275));
#13574=CARTESIAN_POINT('Ctrl Pts',(15.1895240703454,12.4212398264365,4.11222245857373));
#13575=CARTESIAN_POINT('Ctrl Pts',(17.1370409604027,11.1538533719331,4.00108131104472));
#13576=CARTESIAN_POINT('Ctrl Pts',(17.1283950449557,8.83027515929254,3.88994016351569));
#13577=CARTESIAN_POINT('Ctrl Pts',(15.1715004531809,7.57741681981306,3.77879901598667));
#13578=CARTESIAN_POINT('Ctrl Pts',(13.0576211269744,8.54209534468881,3.66765786845765));
#13579=CARTESIAN_POINT('Ctrl Pts',(12.7217186276099,10.8412821515861,3.55651672092863));
#13580=CARTESIAN_POINT('Ctrl Pts',(14.4712648228307,12.3703925377072,3.44537557339962));
#13581=CARTESIAN_POINT('Ctrl Pts',(16.7047942952545,11.7297393101775,3.33423442587059));
#13582=CARTESIAN_POINT('Ctrl Pts',(17.3778224702348,9.50575110480829,3.22309327834158));
#13583=CARTESIAN_POINT('Ctrl Pts',(15.8742859650895,7.73417879746959,3.11195213081255));
#13584=CARTESIAN_POINT('Ctrl Pts',(13.5704626531319,8.0366496380355,3.00081098328354));
#13585=CARTESIAN_POINT('Ctrl Pts',(12.5751813105287,10.1362937769301,2.88966983575452));
#13586=CARTESIAN_POINT('Ctrl Pts',(13.79948312919,12.1111799816138,2.77852868822549));
#13587=CARTESIAN_POINT('Ctrl Pts',(16.1226906277949,12.1535754969733,2.66738754069648));
#13588=CARTESIAN_POINT('Ctrl Pts',(17.4182315125643,10.2246731484105,2.55624639316745));
#13589=CARTESIAN_POINT('Ctrl Pts',(16.5002188767733,8.09011387728591,2.44510524563844));
#13590=CARTESIAN_POINT('Ctrl Pts',(14.208965194919,7.70378886396441,2.33396409810942));
#13591=CARTESIAN_POINT('Ctrl Pts',(12.6417934967878,9.41932472267615,2.2228229505804));
#13592=CARTESIAN_POINT('Ctrl Pts',(13.2332308032177,11.6663878102415,2.11168180305138));
#13593=CARTESIAN_POINT('Ctrl Pts',(15.4418987717874,12.3881053056886,2.00054065552236));
#13594=CARTESIAN_POINT('Ctrl Pts',(17.2460700947607,10.9238457607613,1.88939950799334));
#13595=CARTESIAN_POINT('Ctrl Pts',(16.9942776158352,8.61393405853105,1.77825836046432));
#13596=CARTESIAN_POINT('Ctrl Pts',(14.9170023251788,7.57277284889803,1.6671172129353));
#13597=CARTESIAN_POINT('Ctrl Pts',(12.9156996842814,8.75339838546101,1.55597606540628));
#13598=CARTESIAN_POINT('Ctrl Pts',(12.8222834200456,11.0751157426043,1.44483491787726));
#13599=CARTESIAN_POINT('Ctrl Pts',(14.7222622877187,12.4127108006303,1.33369377034824));
#13600=CARTESIAN_POINT('Ctrl Pts',(16.8764722993871,11.541813251237,1.22255262281922));
#13601=CARTESIAN_POINT('Ctrl Pts',(17.3130317733822,9.25958632559344,1.1114114752902));
#13602=CARTESIAN_POINT('Ctrl Pts',(15.6323372531142,7.65513288048749,1.00027032776118));
#13603=CARTESIAN_POINT('Ctrl Pts',(13.372818760492,8.19702366390889,0.889129180232159));
#13604=CARTESIAN_POINT('Ctrl Pts',(12.6027720863339,10.3893932119062,0.777988032703138));
#13605=CARTESIAN_POINT('Ctrl Pts',(14.0270250684493,12.2251230724266,0.66684688517412));
#13606=CARTESIAN_POINT('Ctrl Pts',(16.3419551102441,12.024459772841,0.555705737645098));
#13607=CARTESIAN_POINT('Ctrl Pts',(17.4284073232916,9.96991710195404,0.444564590116078));
#13608=CARTESIAN_POINT('Ctrl Pts',(16.2921949921082,7.9444041673974,0.333423442587059));
#13609=CARTESIAN_POINT('Ctrl Pts',(13.9727677026847,7.79758395766853,0.222282295058038));
#13610=CARTESIAN_POINT('Ctrl Pts',(12.5943483436034,9.67266534157626,0.111141147529019));
#13611=CARTESIAN_POINT('Ctrl Pts',(13.1427287937432,11.1132850523281,0.0370470491763399));
#13612=CARTESIAN_POINT('Ctrl Pts',(13.6609982804014,11.5585480285869,0.));
#13613=CARTESIAN_POINT('Ctrl Pts',(16.2690708798524,11.0793586530485,8.));
#13614=CARTESIAN_POINT('Ctrl Pts',(16.314784652283,11.0367125551188,8.));
#13615=CARTESIAN_POINT('Ctrl Pts',(16.357765226135,10.9914157787626,8.));
#13616=CARTESIAN_POINT('Ctrl Pts',(16.3980010208502,10.943805412763,8.));
#13617=CARTESIAN_POINT('Ctrl Pts',(16.4235329118048,10.9135939385864,8.));
#13618=CARTESIAN_POINT('Ctrl Pts',(16.4479591518653,10.8824498539581,8.));
#13619=CARTESIAN_POINT('Ctrl Pts',(16.4712714314018,10.8504502532411,8.));
#13620=CARTESIAN_POINT('Ctrl Pts',(16.4873491735028,10.8283811404005,8.));
#13621=CARTESIAN_POINT('Ctrl Pts',(16.5028969805187,10.8059049651785,8.));
#13622=CARTESIAN_POINT('Ctrl Pts',(16.5179108032207,10.7830453876846,8.));
#13623=CARTESIAN_POINT('Ctrl Pts',(16.5257295949839,10.7711407395634,8.));
#13624=CARTESIAN_POINT('Ctrl Pts',(16.5334031154624,10.759132546163,8.));
#13625=CARTESIAN_POINT('Ctrl Pts',(16.5409237973063,10.7470358005141,8.));
#13626=CARTESIAN_POINT('Ctrl Pts',(16.5757596995797,10.6910035074322,8.));
#13627=CARTESIAN_POINT('Ctrl Pts',(16.607360581433,10.6330123468312,8.));
#13628=CARTESIAN_POINT('Ctrl Pts',(16.6356935185973,10.5734135013109,8.));
#13629=CARTESIAN_POINT('Ctrl Pts',(16.65611782791,10.5304505974462,8.));
#13630=CARTESIAN_POINT('Ctrl Pts',(16.6748433410819,10.4866511989788,8.));
#13631=CARTESIAN_POINT('Ctrl Pts',(16.6918460893235,10.4421348904576,8.));
#13632=CARTESIAN_POINT('Ctrl Pts',(16.6965919783289,10.4297092839518,8.));
#13633=CARTESIAN_POINT('Ctrl Pts',(16.7012035820491,10.4172277727484,8.));
#13634=CARTESIAN_POINT('Ctrl Pts',(16.7056802275322,10.4046928500131,8.));
#13635=CARTESIAN_POINT('Ctrl Pts',(16.710058403887,10.3924336477742,8.));
#13636=CARTESIAN_POINT('Ctrl Pts',(16.7143044894992,10.380131701097,8.));
#13637=CARTESIAN_POINT('Ctrl Pts',(16.7184173516006,10.367792630208,8.));
#13638=CARTESIAN_POINT('Ctrl Pts',(16.7398742805331,10.3034193153175,8.));
#13639=CARTESIAN_POINT('Ctrl Pts',(16.7577174338981,10.2380126755093,8.));
#13640=CARTESIAN_POINT('Ctrl Pts',(16.7719142685079,10.1719289098357,8.));
#13641=CARTESIAN_POINT('Ctrl Pts',(16.7863147862362,10.1048970351052,8.));
#13642=CARTESIAN_POINT('Ctrl Pts',(16.796964156607,10.0371675551568,8.));
#13643=CARTESIAN_POINT('Ctrl Pts',(16.8037861146634,9.96908054818257,8.));
#13644=CARTESIAN_POINT('Ctrl Pts',(16.8080115895847,9.92690791415968,8.));
#13645=CARTESIAN_POINT('Ctrl Pts',(16.8107678210036,9.88459754218389,8.));
#13646=CARTESIAN_POINT('Ctrl Pts',(16.8120273023581,9.8422266950913,8.));
#13647=CARTESIAN_POINT('Ctrl Pts',(16.813060369613,9.80747275885079,8.));
#13648=CARTESIAN_POINT('Ctrl Pts',(16.8130863293521,9.77267806685123,8.));
#13649=CARTESIAN_POINT('Ctrl Pts',(16.8120860218337,9.73788470224784,8.));
#13650=CARTESIAN_POINT('Ctrl Pts',(16.8116793102994,9.7237381898587,8.));
#13651=CARTESIAN_POINT('Ctrl Pts',(16.8111026395985,9.70958947886931,8.));
#13652=CARTESIAN_POINT('Ctrl Pts',(16.810356201727,9.69546521518563,8.));
#13653=CARTESIAN_POINT('Ctrl Pts',(16.8066366250451,9.62508255663006,8.));
#13654=CARTESIAN_POINT('Ctrl Pts',(16.7987033737293,9.55518330023832,8.));
#13655=CARTESIAN_POINT('Ctrl Pts',(16.7864936208905,9.48612488219693,8.));
#13656=CARTESIAN_POINT('Ctrl Pts',(16.7851385866999,9.47846080260131,8.));
#13657=CARTESIAN_POINT('Ctrl Pts',(16.7837308318786,9.47080705979357,8.));
#13658=CARTESIAN_POINT('Ctrl Pts',(16.782270233023,9.46316412952721,8.));
#13659=CARTESIAN_POINT('Ctrl Pts',(16.7696151815605,9.39694356837038,8.));
#13660=CARTESIAN_POINT('Ctrl Pts',(16.7529975308864,9.33153486627218,8.));
#13661=CARTESIAN_POINT('Ctrl Pts',(16.7326883279903,9.26714561729205,8.));
#13662=CARTESIAN_POINT('Ctrl Pts',(16.7108362800783,9.19786486014313,8.));
#13663=CARTESIAN_POINT('Ctrl Pts',(16.6847107136327,9.12976334731771,8.));
#13664=CARTESIAN_POINT('Ctrl Pts',(16.6545852471777,9.06310545296145,8.));
#13665=CARTESIAN_POINT('Ctrl Pts',(16.6490327135744,9.05081949553446,8.));
#13666=CARTESIAN_POINT('Ctrl Pts',(16.6433441297437,9.03858262010034,8.));
#13667=CARTESIAN_POINT('Ctrl Pts',(16.6375209875576,9.02639654643794,8.));
#13668=CARTESIAN_POINT('Ctrl Pts',(16.6325866305862,9.01607043115377,8.));
#13669=CARTESIAN_POINT('Ctrl Pts',(16.6275597790168,9.0057894375504,8.));
#13670=CARTESIAN_POINT('Ctrl Pts',(16.6224422427912,8.99555531601222,8.));
#13671=CARTESIAN_POINT('Ctrl Pts',(16.5906563609555,8.93198945862292,8.));
#13672=CARTESIAN_POINT('Ctrl Pts',(16.5553715219545,8.87022144200131,8.));
#13673=CARTESIAN_POINT('Ctrl Pts',(16.5168958154538,8.81047563769863,8.));
#13674=CARTESIAN_POINT('Ctrl Pts',(16.4776074025218,8.74946784748795,8.));
#13675=CARTESIAN_POINT('Ctrl Pts',(16.4349915420324,8.69056773410278,8.));
#13676=CARTESIAN_POINT('Ctrl Pts',(16.3893217542466,8.63402247023065,8.));
#13677=CARTESIAN_POINT('Ctrl Pts',(16.3433740602154,8.5771331215108,8.));
#13678=CARTESIAN_POINT('Ctrl Pts',(16.2943346227761,8.522626437839,8.));
#13679=CARTESIAN_POINT('Ctrl Pts',(16.2424343742239,8.47077604070952,8.));
#13680=CARTESIAN_POINT('Ctrl Pts',(16.2296036049381,8.45795759568269,8.));
#13681=CARTESIAN_POINT('Ctrl Pts',(16.2165977853048,8.44530163917201,8.));
#13682=CARTESIAN_POINT('Ctrl Pts',(16.2034200194896,8.43281261409566,8.));
#13683=CARTESIAN_POINT('Ctrl Pts',(16.1931256240804,8.42305625901894,8.));
#13684=CARTESIAN_POINT('Ctrl Pts',(16.1827250344693,8.41340078989772,8.));
#13685=CARTESIAN_POINT('Ctrl Pts',(16.172235821794,8.40386260566874,8.));
#13686=CARTESIAN_POINT('Ctrl Pts',(16.1164871858091,8.35316854721106,8.));
#13687=CARTESIAN_POINT('Ctrl Pts',(16.0581411327798,8.30569128093942,8.));
#13688=CARTESIAN_POINT('Ctrl Pts',(15.9974954185764,8.26168435413653,8.));
#13689=CARTESIAN_POINT('Ctrl Pts',(15.9367829241817,8.2176289689879,8.));
#13690=CARTESIAN_POINT('Ctrl Pts',(15.873765062306,8.17705063925328,8.));
#13691=CARTESIAN_POINT('Ctrl Pts',(15.8086958538675,8.14023020006429,8.));
#13692=CARTESIAN_POINT('Ctrl Pts',(15.745109232976,8.10424870645226,8.));
#13693=CARTESIAN_POINT('Ctrl Pts',(15.6795629473788,8.07185507016062,8.));
#13694=CARTESIAN_POINT('Ctrl Pts',(15.6122617289213,8.0433487143013,8.));
#13695=CARTESIAN_POINT('Ctrl Pts',(15.597755809183,8.03720453267124,8.));
#13696=CARTESIAN_POINT('Ctrl Pts',(15.5831682628234,8.03124110383924,8.));
#13697=CARTESIAN_POINT('Ctrl Pts',(15.5685009870302,8.0254617116896,8.));
#13698=CARTESIAN_POINT('Ctrl Pts',(15.5561467177936,8.02059372068384,8.));
#13699=CARTESIAN_POINT('Ctrl Pts',(15.5437358816804,8.01585630076653,8.));
#13700=CARTESIAN_POINT('Ctrl Pts',(15.531270276981,8.01124903105919,8.));
#13701=CARTESIAN_POINT('Ctrl Pts',(13.3326898978632,9.99870038716915,6.87148036339021));
#13702=CARTESIAN_POINT('Ctrl Pts',(13.331960273942,9.91361837560012,6.87718308383007));
#13703=CARTESIAN_POINT('Ctrl Pts',(13.3379104352826,9.82863878514235,6.88288580426994));
#13704=CARTESIAN_POINT('Ctrl Pts',(13.3508951624844,9.74474812612374,6.8885885247098));
#13705=CARTESIAN_POINT('Ctrl Pts',(13.4352489077286,9.19976237715157,6.92563557388614));
#13706=CARTESIAN_POINT('Ctrl Pts',(13.8164822690384,8.7007327758593,6.96268262306248));
#13707=CARTESIAN_POINT('Ctrl Pts',(14.3201120460454,8.4760440554274,6.99972967223882));
#13708=CARTESIAN_POINT('Ctrl Pts',(14.8237418230524,8.2513553349955,7.03677672141516));
#13709=CARTESIAN_POINT('Ctrl Pts',(15.4497680157567,8.30100749542397,7.0738237705915));
#13710=CARTESIAN_POINT('Ctrl Pts',(15.9116712512052,8.60229753421573,7.11087081976784));
#13711=CARTESIAN_POINT('Ctrl Pts',(16.3735744866537,8.90358757300749,7.14791786894418));
#13712=CARTESIAN_POINT('Ctrl Pts',(16.6713547648465,9.45651549016254,7.18496491812052));
#13713=CARTESIAN_POINT('Ctrl Pts',(16.6687230854429,10.007974828459,7.22201196729686));
#13714=CARTESIAN_POINT('Ctrl Pts',(16.6660914060393,10.5594341667554,7.2590590164732));
#13715=CARTESIAN_POINT('Ctrl Pts',(16.3630477690393,11.1094249261933,7.29610606564954));
#13716=CARTESIAN_POINT('Ctrl Pts',(15.8982909122512,11.4063091733054,7.33315311482588));
#13717=CARTESIAN_POINT('Ctrl Pts',(15.433534055463,11.7031934204176,7.37020016400222));
#13718=CARTESIAN_POINT('Ctrl Pts',(14.8070639788868,11.746971155204,7.40724721317856));
#13719=CARTESIAN_POINT('Ctrl Pts',(14.3056004316898,11.5174472457193,7.4442942623549));
#13720=CARTESIAN_POINT('Ctrl Pts',(13.8041368844929,11.2879233362346,7.48134131153124));
#13721=CARTESIAN_POINT('Ctrl Pts',(13.4276798666754,10.7850977824788,7.51838836070758));
#13722=CARTESIAN_POINT('Ctrl Pts',(13.3485326690949,10.2394123380852,7.55543540988392));
#13723=CARTESIAN_POINT('Ctrl Pts',(13.3371065399469,10.1606341557557,7.56078372771935));
#13724=CARTESIAN_POINT('Ctrl Pts',(13.3318767677375,10.0809627127174,7.56613204555478));
#13725=CARTESIAN_POINT('Ctrl Pts',(13.3325428889984,10.0012066618994,7.57148036339021));
#13726=CARTESIAN_POINT('Ctrl Pts',(14.4698297828114,8.01482567432828,8.));
#13727=CARTESIAN_POINT('Ctrl Pts',(13.8096927451188,8.1911250512252,7.96295295082366));
#13728=CARTESIAN_POINT('Ctrl Pts',(12.6905567406518,9.25114015972233,7.88885885247099));
#13729=CARTESIAN_POINT('Ctrl Pts',(13.1189039003815,11.5386115720214,7.77771770494195));
#13730=CARTESIAN_POINT('Ctrl Pts',(15.2723377259255,12.4126882042673,7.66657655741295));
#13731=CARTESIAN_POINT('Ctrl Pts',(17.1748665662283,11.0807510628696,7.55543540988391));
#13732=CARTESIAN_POINT('Ctrl Pts',(17.0874397300721,8.75827685188236,7.44429426235491));
#13733=CARTESIAN_POINT('Ctrl Pts',(15.0888245216199,7.57307606901691,7.33315311482588));
#13734=CARTESIAN_POINT('Ctrl Pts',(13.0091239883167,8.60905062621059,7.22201196729686));
#13735=CARTESIAN_POINT('Ctrl Pts',(12.7516785328344,10.9184180508126,7.11087081976784));
#13736=CARTESIAN_POINT('Ctrl Pts',(14.552316547407,12.3870127270114,6.99972967223883));
#13737=CARTESIAN_POINT('Ctrl Pts',(16.7627159052523,11.6706763447836,6.8885885247098));
#13738=CARTESIAN_POINT('Ctrl Pts',(17.359610496679,9.42504513942049,6.77744737718079));
#13739=CARTESIAN_POINT('Ctrl Pts',(15.796602835303,7.70571713781293,6.66630622965176));
#13740=CARTESIAN_POINT('Ctrl Pts',(13.5044206094209,8.08647863727104,6.55516508212274));
#13741=CARTESIAN_POINT('Ctrl Pts',(12.581230473367,10.218805203436,6.44402393459371));
#13742=CARTESIAN_POINT('Ctrl Pts',(13.8720874462699,12.1508444526632,6.33288278706471));
#13743=CARTESIAN_POINT('Ctrl Pts',(16.1953904039119,12.1140865945272,6.22174163953568));
#13744=CARTESIAN_POINT('Ctrl Pts',(17.4244805427636,10.1421770013196,6.11060049200667));
#13745=CARTESIAN_POINT('Ctrl Pts',(16.4342968937075,8.04012443367538,5.99945934447764));
#13746=CARTESIAN_POINT('Ctrl Pts',(14.1312146531314,7.73206435471271,5.88831819694863));
#13747=CARTESIAN_POINT('Ctrl Pts',(12.6233841302342,9.49998296241927,5.77717704941961));
#13748=CARTESIAN_POINT('Ctrl Pts',(13.2910138340933,11.7255973659335,5.66603590189058));
#13749=CARTESIAN_POINT('Ctrl Pts',(15.5229818972268,12.3716681799822,5.55489475436157));
#13750=CARTESIAN_POINT('Ctrl Pts',(17.2762330137476,10.8468076994282,5.44375360683255));
#13751=CARTESIAN_POINT('Ctrl Pts',(16.9459104193154,8.54681293441946,5.33261245930352));
#13752=CARTESIAN_POINT('Ctrl Pts',(14.8343783616792,7.57700815405708,5.22147131177451));
#13753=CARTESIAN_POINT('Ctrl Pts',(12.874449803007,8.82511431568684,5.11033016424549));
#13754=CARTESIAN_POINT('Ctrl Pts',(12.8601658597075,11.1486643820772,4.99918901671646));
#13755=CARTESIAN_POINT('Ctrl Pts',(14.8046014881481,12.4207724868025,4.88804786918745));
#13756=CARTESIAN_POINT('Ctrl Pts',(16.9278971892049,11.4770011641531,4.77690672165842));
#13757=CARTESIAN_POINT('Ctrl Pts',(17.2864720241886,9.18124137035986,4.66576557412941));
#13758=CARTESIAN_POINT('Ctrl Pts',(15.5521007657847,7.63494085580992,4.55462442660038));
#13759=CARTESIAN_POINT('Ctrl Pts',(13.3123582941187,8.25352197734149,4.44348327907137));
#13760=CARTESIAN_POINT('Ctrl Pts',(12.6174163177399,10.4707600323777,4.33234213154234));
#13761=CARTESIAN_POINT('Ctrl Pts',(14.1033972467191,12.2570829656611,4.22120098401333));
#13762=CARTESIAN_POINT('Ctrl Pts',(16.4100928881365,11.9773613877815,4.11005983648431));
#13763=CARTESIAN_POINT('Ctrl Pts',(17.4260452489189,9.88764137211515,3.99891868895528));
#13764=CARTESIAN_POINT('Ctrl Pts',(16.2212917045089,7.90077000222407,3.88777754142627));
#13765=CARTESIAN_POINT('Ctrl Pts',(13.8986160185493,7.83545077753679,3.77663639389725));
#13766=CARTESIAN_POINT('Ctrl Pts',(12.584103685101,9.7514743338816,3.66549524636823));
#13767=CARTESIAN_POINT('Ctrl Pts',(13.4810073238894,11.8949884593291,3.5543540988392));
#13768=CARTESIAN_POINT('Ctrl Pts',(15.7683368037833,12.3039050690097,3.44321295131019));
#13769=CARTESIAN_POINT('Ctrl Pts',(17.3523611503097,10.6039180652812,3.33207180378117));
#13770=CARTESIAN_POINT('Ctrl Pts',(16.7831271023553,8.35112834097283,3.22093065625215));
#13771=CARTESIAN_POINT('Ctrl Pts',(14.5816890022697,7.60765054388266,3.10978950872313));
#13772=CARTESIAN_POINT('Ctrl Pts',(12.7631562512648,9.05403485540002,2.99864836119411));
#13773=CARTESIAN_POINT('Ctrl Pts',(12.9921418323749,11.366318260873,2.88750721366509));
#13774=CARTESIAN_POINT('Ctrl Pts',(15.0590413979142,12.4279279486728,2.77636606613607));
#13775=CARTESIAN_POINT('Ctrl Pts',(17.071896801884,11.2671083826901,2.66522491860705));
#13776=CARTESIAN_POINT('Ctrl Pts',(17.1882197878565,8.94642789870889,2.55408377107803));
#13777=CARTESIAN_POINT('Ctrl Pts',(15.3015328924376,7.59014566366572,2.44294262354901));
#13778=CARTESIAN_POINT('Ctrl Pts',(13.138834709854,8.43974881014599,2.33180147601999));
#13779=CARTESIAN_POINT('Ctrl Pts',(12.6797736488162,10.7175442146931,2.22066032849097));
#13780=CARTESIAN_POINT('Ctrl Pts',(14.3445560622211,12.3385280047513,2.10951918096195));
#13781=CARTESIAN_POINT('Ctrl Pts',(16.6093059338468,11.8189157324019,1.99837803343293));
#13782=CARTESIAN_POINT('Ctrl Pts',(17.4009607961183,9.63433987693309,1.88723688590391));
#13783=CARTESIAN_POINT('Ctrl Pts',(15.9948710360845,7.78447490731078,1.77609573837489));
#13784=CARTESIAN_POINT('Ctrl Pts',(13.6781157275128,7.96261388733151,1.66495459084587));
#13785=CARTESIAN_POINT('Ctrl Pts',(12.5713608945246,10.0056958124789,1.55381344331685));
#13786=CARTESIAN_POINT('Ctrl Pts',(13.6876865240177,12.0435635368564,1.44267229578783));
#13787=CARTESIAN_POINT('Ctrl Pts',(16.0052515541106,12.2108349221453,1.33153114825881));
#13788=CARTESIAN_POINT('Ctrl Pts',(17.402649969509,10.3543936274306,1.22039000072979));
#13789=CARTESIAN_POINT('Ctrl Pts',(16.6007558214423,8.1735579042694,1.10924885320077));
#13790=CARTESIAN_POINT('Ctrl Pts',(14.333596515509,7.6645683089416,0.998107705671753));
#13791=CARTESIAN_POINT('Ctrl Pts',(12.6764299583764,9.29335364338448,0.886966558142731));
#13792=CARTESIAN_POINT('Ctrl Pts',(13.1461804472137,11.5689497437289,0.775825410613713));
#13793=CARTESIAN_POINT('Ctrl Pts',(15.3128190766481,12.4084404416678,0.664684263084692));
#13794=CARTESIAN_POINT('Ctrl Pts',(17.1931639076296,11.0432447117585,0.553543115555672));
#13795=CARTESIAN_POINT('Ctrl Pts',(17.0658793839574,8.72328862566383,0.442401968026654));
#13796=CARTESIAN_POINT('Ctrl Pts',(15.0477523711852,7.57162591137588,0.331260820497632));
#13797=CARTESIAN_POINT('Ctrl Pts',(12.985562223504,8.64349423686535,0.220119672968612));
#13798=CARTESIAN_POINT('Ctrl Pts',(12.7679935470831,10.9557088479816,0.108978525439593));
#13799=CARTESIAN_POINT('Ctrl Pts',(14.592171500868,12.3957303731543,-0.00216262208942797));
#13800=CARTESIAN_POINT('Ctrl Pts',(16.7924309645196,11.6375318213583,-0.113303769618446));
#13801=CARTESIAN_POINT('Ctrl Pts',(17.160799328377,10.1407345153594,-0.187397867971127));
#13802=CARTESIAN_POINT('Ctrl Pts',(16.9877912008532,9.47972727890995,-0.224444917147467));
#13803=CARTESIAN_POINT('Ctrl Pts',(14.5032651029123,8.14002119999724,8.07481497238249));
#13804=CARTESIAN_POINT('Ctrl Pts',(13.8847597760366,8.30520221168044,8.03776792320615));
#13805=CARTESIAN_POINT('Ctrl Pts',(12.8362023694098,9.29836719673542,7.96367382485347));
#13806=CARTESIAN_POINT('Ctrl Pts',(13.2375357061529,11.4415786404201,7.85253267732445));
#13807=CARTESIAN_POINT('Ctrl Pts',(15.2551626777114,12.2605314066992,7.74139152979544));
#13808=CARTESIAN_POINT('Ctrl Pts',(17.0377080509797,11.012593221171,7.63025038226641));
#13809=CARTESIAN_POINT('Ctrl Pts',(16.955794810566,8.83658643923375,7.51910923473739));
#13810=CARTESIAN_POINT('Ctrl Pts',(15.0832227804868,7.7261306463247,7.40796808720837));
#13811=CARTESIAN_POINT('Ctrl Pts',(13.1346790922697,8.69677120358184,7.29682693967935));
#13812=CARTESIAN_POINT('Ctrl Pts',(12.8934695001639,10.8604977819634,7.18568579215033));
#13813=CARTESIAN_POINT('Ctrl Pts',(14.5805498186396,12.2364751599715,7.07454464462132));
#13814=CARTESIAN_POINT('Ctrl Pts',(16.6515497766613,11.5653147145716,6.96340349709228));
#13815=CARTESIAN_POINT('Ctrl Pts',(17.2108010582909,9.46130481449049,6.85226234956328));
#13816=CARTESIAN_POINT('Ctrl Pts',(15.7463648741197,7.85040667225349,6.74112120203425));
#13817=CARTESIAN_POINT('Ctrl Pts',(13.5987397055133,8.2071553505388,6.62998005450523));
#13818=CARTESIAN_POINT('Ctrl Pts',(12.7337707910827,10.2050061974197,6.51883890697622));
#13819=CARTESIAN_POINT('Ctrl Pts',(13.94321953943,12.0152008981395,6.40769775944718));
#13820=CARTESIAN_POINT('Ctrl Pts',(16.1200028029027,11.9807611837112,6.29655661191817));
#13821=CARTESIAN_POINT('Ctrl Pts',(17.2715800583576,10.1332105724332,6.18541546438915));
#13822=CARTESIAN_POINT('Ctrl Pts',(16.3438425939259,8.16372448662726,6.07427431686013));
#13823=CARTESIAN_POINT('Ctrl Pts',(14.1860048228349,7.87509229519298,5.96313316933112));
#13824=CARTESIAN_POINT('Ctrl Pts',(12.7732660168176,9.53151666455001,5.85199202180209));
#13825=CARTESIAN_POINT('Ctrl Pts',(13.398791482955,11.6167721275012,5.74085087427307));
#13826=CARTESIAN_POINT('Ctrl Pts',(15.4899999103595,12.2220983207182,5.62970972674405));
#13827=CARTESIAN_POINT('Ctrl Pts',(17.132681797607,10.7934035556714,5.51856857921503));
#13828=CARTESIAN_POINT('Ctrl Pts',(16.823191081925,8.63845854771295,5.40742743168601));
#13829=CARTESIAN_POINT('Ctrl Pts',(14.8448233325836,7.72981475341796,5.296286284157));
#13830=CARTESIAN_POINT('Ctrl Pts',(13.0084981688392,8.8992087813196,5.18514513662797));
#13831=CARTESIAN_POINT('Ctrl Pts',(12.9951150460706,11.0762235695643,5.07400398909895));
#13832=CARTESIAN_POINT('Ctrl Pts',(14.8169243451838,12.2681058518924,4.96286284156994));
#13833=CARTESIAN_POINT('Ctrl Pts',(16.8063138607702,11.3838537086533,4.85172169404091));
#13834=CARTESIAN_POINT('Ctrl Pts',(17.1422750822405,9.23287659236945,4.7405805465119));
#13835=CARTESIAN_POINT('Ctrl Pts',(15.5172823900376,7.78409391454438,4.62943939898287));
#13836=CARTESIAN_POINT('Ctrl Pts',(13.4187898491597,8.3636640597211,4.51829825145385));
#13837=CARTESIAN_POINT('Ctrl Pts',(12.7676745659418,10.4410714307495,4.40715710392483));
#13838=CARTESIAN_POINT('Ctrl Pts',(14.15994172826,12.1147394521922,4.29601595639582));
#13839=CARTESIAN_POINT('Ctrl Pts',(16.3211650201456,11.8526585870353,4.18487480886679));
#13840=CARTESIAN_POINT('Ctrl Pts',(17.2730460859198,9.89472729766818,4.07373366133777));
#13841=CARTESIAN_POINT('Ctrl Pts',(16.1442706313649,8.033158477973,3.96259251380876));
#13842=CARTESIAN_POINT('Ctrl Pts',(13.9680750805259,7.97195862686682,3.85145136627974));
#13843=CARTESIAN_POINT('Ctrl Pts',(12.7364628029851,9.76714766846464,3.74031021875072));
#13844=CARTESIAN_POINT('Ctrl Pts',(13.5768029848114,11.7754805283458,3.62916907122169));
#13845=CARTESIAN_POINT('Ctrl Pts',(15.7198814470942,12.1586087076392,3.51802792369268));
#13846=CARTESIAN_POINT('Ctrl Pts',(17.2040088938011,10.5658318183123,3.40688677616365));
#13847=CARTESIAN_POINT('Ctrl Pts',(16.670673736408,8.45511485311085,3.29574562863464));
#13848=CARTESIAN_POINT('Ctrl Pts',(14.6080698921375,7.75852467310611,3.18460448110562));
#13849=CARTESIAN_POINT('Ctrl Pts',(12.9042233733512,9.11369238875171,3.0734633335766));
#13850=CARTESIAN_POINT('Ctrl Pts',(13.1187679203279,11.2801510509262,2.96232218604758));
#13851=CARTESIAN_POINT('Ctrl Pts',(15.0553179370813,12.274810052733,2.85118103851855));
#13852=CARTESIAN_POINT('Ctrl Pts',(16.9412321011123,11.1871978690395,2.74003989098954));
#13853=CARTESIAN_POINT('Ctrl Pts',(17.0502191482768,9.01287169225666,2.62889874346052));
#13854=CARTESIAN_POINT('Ctrl Pts',(15.2825166435939,7.7421237426291,2.5177575959315));
#13855=CARTESIAN_POINT('Ctrl Pts',(13.2562095740377,8.53814644977055,2.40661644840248));
#13856=CARTESIAN_POINT('Ctrl Pts',(12.8260993160138,10.6722921056024,2.29547530087346));
#13857=CARTESIAN_POINT('Ctrl Pts',(14.3858918014937,12.191048139099,2.18433415334444));
#13858=CARTESIAN_POINT('Ctrl Pts',(16.5078146442685,11.7042053473638,2.07319300581542));
#13859=CARTESIAN_POINT('Ctrl Pts',(17.2495435905392,9.65740032594834,1.9620518582864));
#13860=CARTESIAN_POINT('Ctrl Pts',(15.9321292402005,7.92419756291088,1.85091071075738));
#13861=CARTESIAN_POINT('Ctrl Pts',(13.7614806966379,8.09110216267724,1.73976956322836));
#13862=CARTESIAN_POINT('Ctrl Pts',(12.7245236397496,10.0053366046107,1.62862841569934));
#13863=CARTESIAN_POINT('Ctrl Pts',(13.7704479084177,11.9146856806772,1.51748726817032));
#13864=CARTESIAN_POINT('Ctrl Pts',(15.9418551082072,12.0714080533479,1.4063461206413));
#13865=CARTESIAN_POINT('Ctrl Pts',(17.2511262357788,10.332043702839,1.29520497311228));
#13866=CARTESIAN_POINT('Ctrl Pts',(16.4998037468857,8.28874294133233,1.18406382558326));
#13867=CARTESIAN_POINT('Ctrl Pts',(14.3756234213931,7.81185290478036,1.07292267805424));
#13868=CARTESIAN_POINT('Ctrl Pts',(12.8229664962652,9.33791847627317,0.961781530525221));
#13869=CARTESIAN_POINT('Ctrl Pts',(13.2630920505954,11.4700035275835,0.850640382996202));
#13870=CARTESIAN_POINT('Ctrl Pts',(15.2930910617157,12.2565515303325,0.739499235467181));
#13871=CARTESIAN_POINT('Ctrl Pts',(17.0548514658741,10.9774522176682,0.628358087938162));
#13872=CARTESIAN_POINT('Ctrl Pts',(16.9355941731834,8.80380475443427,0.517216940409142));
#13873=CARTESIAN_POINT('Ctrl Pts',(15.0447408557051,7.72477194324555,0.406075792880122));
#13874=CARTESIAN_POINT('Ctrl Pts',(13.1126032561702,8.72904261913709,0.294934645351101));
#13875=CARTESIAN_POINT('Ctrl Pts',(12.9087556038737,10.8954368254885,0.183793497822082));
#13876=CARTESIAN_POINT('Ctrl Pts',(14.6178913092855,12.2446430255347,0.0726523502930609));
#13877=CARTESIAN_POINT('Ctrl Pts',(16.6793908481296,11.5342604589779,-0.0384887972359571));
#13878=CARTESIAN_POINT('Ctrl Pts',(17.0245279670748,10.1318590572183,-0.112582895588638));
#13879=CARTESIAN_POINT('Ctrl Pts',(16.8624306412829,9.51253841089255,-0.149629944764978));
#13880=CARTESIAN_POINT('Ctrl Pts',(14.5367004230132,8.26521672566619,8.14962994476498));
#13881=CARTESIAN_POINT('Ctrl Pts',(13.9598268069544,8.41927937213568,8.11258289558864));
#13882=CARTESIAN_POINT('Ctrl Pts',(12.9818479981678,9.34559423374852,8.03848879723595));
#13883=CARTESIAN_POINT('Ctrl Pts',(13.3561675119244,11.3445457088188,7.92734764970695));
#13884=CARTESIAN_POINT('Ctrl Pts',(15.2379876294974,12.1083746091312,7.81620650217792));
#13885=CARTESIAN_POINT('Ctrl Pts',(16.9005495357311,10.9444353794724,7.7050653546489));
#13886=CARTESIAN_POINT('Ctrl Pts',(16.8241498910599,8.91489602658511,7.59392420711988));
#13887=CARTESIAN_POINT('Ctrl Pts',(15.0776210393537,7.87918522363254,7.48278305959087));
#13888=CARTESIAN_POINT('Ctrl Pts',(13.2602341962226,8.78449178095305,7.37164191206184));
#13889=CARTESIAN_POINT('Ctrl Pts',(13.0352604674934,10.8025775131143,7.26050076453282));
#13890=CARTESIAN_POINT('Ctrl Pts',(14.6087830898722,12.0859375929316,7.1493596170038));
#13891=CARTESIAN_POINT('Ctrl Pts',(16.5403836480704,11.4599530843595,7.03821846947479));
#13892=CARTESIAN_POINT('Ctrl Pts',(17.0619916199027,9.49756448956049,6.92707732194575));
#13893=CARTESIAN_POINT('Ctrl Pts',(15.6961269129365,7.99509620669406,6.81593617441675));
#13894=CARTESIAN_POINT('Ctrl Pts',(13.6930588016057,8.32783206380658,6.70479502688771));
#13895=CARTESIAN_POINT('Ctrl Pts',(12.8863111087983,10.1912071914035,6.59365387935871));
#13896=CARTESIAN_POINT('Ctrl Pts',(14.0143516325902,11.8795573436157,6.48251273182967));
#13897=CARTESIAN_POINT('Ctrl Pts',(16.0446152018935,11.8474357728952,6.37137158430067));
#13898=CARTESIAN_POINT('Ctrl Pts',(17.1186795739517,10.1242441435468,6.26023043677163));
#13899=CARTESIAN_POINT('Ctrl Pts',(16.2533882941443,8.28732453957915,6.14908928924263));
#13900=CARTESIAN_POINT('Ctrl Pts',(14.2407949925385,8.01812023567324,6.0379481417136));
#13901=CARTESIAN_POINT('Ctrl Pts',(12.9231479034009,9.56305036668077,5.92680699418458));
#13902=CARTESIAN_POINT('Ctrl Pts',(13.5065691318168,11.5079468890688,5.81566584665556));
#13903=CARTESIAN_POINT('Ctrl Pts',(15.4570179234921,12.0725284614542,5.70452469912655));
#13904=CARTESIAN_POINT('Ctrl Pts',(16.9891305814665,10.7399994119146,5.59338355159752));
#13905=CARTESIAN_POINT('Ctrl Pts',(16.7004717445346,8.73010416100646,5.4822424040685));
#13906=CARTESIAN_POINT('Ctrl Pts',(14.8552683034879,7.88262135277884,5.37110125653948));
#13907=CARTESIAN_POINT('Ctrl Pts',(13.1425465346714,8.97330324695236,5.25996010901047));
#13908=CARTESIAN_POINT('Ctrl Pts',(13.1300642324337,11.0037827570514,5.14881896148144));
#13909=CARTESIAN_POINT('Ctrl Pts',(14.8292472022195,12.1154392169823,5.03767781395242));
#13910=CARTESIAN_POINT('Ctrl Pts',(16.6847305323356,11.2907062531535,4.92653666642341));
#13911=CARTESIAN_POINT('Ctrl Pts',(16.9980781402925,9.28451181437904,4.81539551889438));
#13912=CARTESIAN_POINT('Ctrl Pts',(15.4824640142906,7.93324697327884,4.70425437136536));
#13913=CARTESIAN_POINT('Ctrl Pts',(13.5252214042007,8.4738061421007,4.59311322383634));
#13914=CARTESIAN_POINT('Ctrl Pts',(12.9179328141437,10.4113828291212,4.48197207630733));
#13915=CARTESIAN_POINT('Ctrl Pts',(14.2164862098008,11.9723959387232,4.3708309287783));
#13916=CARTESIAN_POINT('Ctrl Pts',(16.2322371521546,11.727955786289,4.25968978124929));
#13917=CARTESIAN_POINT('Ctrl Pts',(17.1200469229207,9.90181322322121,4.14854863372026));
#13918=CARTESIAN_POINT('Ctrl Pts',(16.0672495582209,8.16554695372194,4.03740748619125));
#13919=CARTESIAN_POINT('Ctrl Pts',(14.0375341425024,8.10846647619684,3.92626633866222));
#13920=CARTESIAN_POINT('Ctrl Pts',(12.8888219208692,9.78282100304769,3.81512519113321));
#13921=CARTESIAN_POINT('Ctrl Pts',(13.6725986457333,11.6559725973624,3.70398404360418));
#13922=CARTESIAN_POINT('Ctrl Pts',(15.6714260904051,12.0133123462689,3.59284289607517));
#13923=CARTESIAN_POINT('Ctrl Pts',(17.0556566372925,10.5277455713434,3.48170174854614));
#13924=CARTESIAN_POINT('Ctrl Pts',(16.5582203704607,8.55910136524887,3.37056060101713));
#13925=CARTESIAN_POINT('Ctrl Pts',(14.6344507820053,7.90939880232955,3.2594194534881));
#13926=CARTESIAN_POINT('Ctrl Pts',(13.0452904954375,9.17334992210343,3.14827830595909));
#13927=CARTESIAN_POINT('Ctrl Pts',(13.2453940082809,11.1939838409794,3.03713715843007));
#13928=CARTESIAN_POINT('Ctrl Pts',(15.0515944762484,12.1216921567933,2.92599601090104));
#13929=CARTESIAN_POINT('Ctrl Pts',(16.8105674003405,11.1072873553889,2.81485486337203));
#13930=CARTESIAN_POINT('Ctrl Pts',(16.9122185086971,9.07931548580447,2.703713715843));
#13931=CARTESIAN_POINT('Ctrl Pts',(15.2635003947501,7.89410182159245,2.59257256831399));
#13932=CARTESIAN_POINT('Ctrl Pts',(13.3735844382213,8.63654408939513,2.48143142078496));
#13933=CARTESIAN_POINT('Ctrl Pts',(12.9724249832114,10.6270399965118,2.37029027325595));
#13934=CARTESIAN_POINT('Ctrl Pts',(14.4272275407664,12.0435682734467,2.25914912572692));
#13935=CARTESIAN_POINT('Ctrl Pts',(16.4063233546902,11.5894949623257,2.14800797819791));
#13936=CARTESIAN_POINT('Ctrl Pts',(17.0981263849601,9.6804607749636,2.03686683066889));
#13937=CARTESIAN_POINT('Ctrl Pts',(15.8693874443165,8.06392021851098,1.92572568313987));
#13938=CARTESIAN_POINT('Ctrl Pts',(13.844845665763,8.21959043802295,1.81458453561085));
#13939=CARTESIAN_POINT('Ctrl Pts',(12.8776863849747,10.0049773967426,1.70344338808183));
#13940=CARTESIAN_POINT('Ctrl Pts',(13.8532092928178,11.7858078244979,1.59230224055281));
#13941=CARTESIAN_POINT('Ctrl Pts',(15.8784586623037,11.9319811845506,1.48116109302379));
#13942=CARTESIAN_POINT('Ctrl Pts',(17.0996025020485,10.3096937782474,1.37001994549477));
#13943=CARTESIAN_POINT('Ctrl Pts',(16.398851672329,8.40392797839529,1.25887879796575));
#13944=CARTESIAN_POINT('Ctrl Pts',(14.4176503272771,7.95913750061909,1.14773765043673));
#13945=CARTESIAN_POINT('Ctrl Pts',(12.969503034154,9.3824833091619,1.03659650290771));
#13946=CARTESIAN_POINT('Ctrl Pts',(13.3800036539771,11.371057311438,0.92545535537869));
#13947=CARTESIAN_POINT('Ctrl Pts',(15.2733630467833,12.1046626189973,0.814314207849671));
#13948=CARTESIAN_POINT('Ctrl Pts',(16.9165390241187,10.9116597235779,0.70317306032065));
#13949=CARTESIAN_POINT('Ctrl Pts',(16.8053089624094,8.88432088320471,0.592031912791632));
#13950=CARTESIAN_POINT('Ctrl Pts',(15.041729340225,7.87791797511523,0.480890765262611));
#13951=CARTESIAN_POINT('Ctrl Pts',(13.2396442888365,8.81459100140882,0.36974961773359));
#13952=CARTESIAN_POINT('Ctrl Pts',(13.0495176606643,10.8351648029955,0.258608470204571));
#13953=CARTESIAN_POINT('Ctrl Pts',(14.643611117703,12.0935556779152,0.14746732267555));
#13954=CARTESIAN_POINT('Ctrl Pts',(16.5663507317396,11.4309890965976,0.0363261751465319));
#13955=CARTESIAN_POINT('Ctrl Pts',(16.8882566057727,10.1229835990773,-0.0377679232061492));
#13956=CARTESIAN_POINT('Ctrl Pts',(16.7370700817125,9.54534954287515,-0.0748149723824891));
#13957=CARTESIAN_POINT('Ctrl Pts',(14.5701357431141,8.39041225133515,8.22444491714747));
#13958=CARTESIAN_POINT('Ctrl Pts',(14.0348938378722,8.53335653259092,8.18739786797113));
#13959=CARTESIAN_POINT('Ctrl Pts',(13.1274936269258,9.39282127076158,8.11330376961845));
#13960=CARTESIAN_POINT('Ctrl Pts',(13.4747993176958,11.2475127772175,8.00216262208943));
#13961=CARTESIAN_POINT('Ctrl Pts',(15.2208125812833,11.9562178115631,7.89102147456041));
#13962=CARTESIAN_POINT('Ctrl Pts',(16.7633910204825,10.8762775377738,7.77988032703138));
#13963=CARTESIAN_POINT('Ctrl Pts',(16.6925049715538,8.99320561393648,7.66873917950237));
#13964=CARTESIAN_POINT('Ctrl Pts',(15.0720192982206,8.03223980094035,7.55759803197335));
#13965=CARTESIAN_POINT('Ctrl Pts',(13.3857893001755,8.87221235832429,7.44645688444433));
#13966=CARTESIAN_POINT('Ctrl Pts',(13.1770514348228,10.7446572442652,7.33531573691531));
#13967=CARTESIAN_POINT('Ctrl Pts',(14.6370163611048,11.9354000258917,7.22417458938629));
#13968=CARTESIAN_POINT('Ctrl Pts',(16.4292175194794,11.3545914541475,7.11303344185728));
#13969=CARTESIAN_POINT('Ctrl Pts',(16.9131821815146,9.53382416463051,7.00189229432824));
#13970=CARTESIAN_POINT('Ctrl Pts',(15.6458889517532,8.1397857411346,6.89075114679924));
#13971=CARTESIAN_POINT('Ctrl Pts',(13.7873778976981,8.44850877707437,6.7796099992702));
#13972=CARTESIAN_POINT('Ctrl Pts',(13.0388514265139,10.1774081853872,6.6684688517412));
#13973=CARTESIAN_POINT('Ctrl Pts',(14.0854837257504,11.743913789092,6.55732770421216));
#13974=CARTESIAN_POINT('Ctrl Pts',(15.9692276008844,11.7141103620792,6.44618655668316));
#13975=CARTESIAN_POINT('Ctrl Pts',(16.9657790895458,10.1152777146604,6.33504540915412));
#13976=CARTESIAN_POINT('Ctrl Pts',(16.1629339943627,8.41092459253105,6.22390426162512));
#13977=CARTESIAN_POINT('Ctrl Pts',(14.295585162242,8.16114817615349,6.11276311409608));
#13978=CARTESIAN_POINT('Ctrl Pts',(13.0730297899843,9.59458406881153,6.00162196656708));
#13979=CARTESIAN_POINT('Ctrl Pts',(13.6143467806786,11.3991216506364,5.89048081903804));
#13980=CARTESIAN_POINT('Ctrl Pts',(15.4240359366248,11.9229586021902,5.77933967150904));
#13981=CARTESIAN_POINT('Ctrl Pts',(16.8455793653259,10.6865952681579,5.66819852398001));
#13982=CARTESIAN_POINT('Ctrl Pts',(16.5777524071442,8.82174977429995,5.55705737645099));
#13983=CARTESIAN_POINT('Ctrl Pts',(14.8657132743923,8.03542795213972,5.44591622892198));
#13984=CARTESIAN_POINT('Ctrl Pts',(13.2765949005036,9.04739771258512,5.33477508139295));
#13985=CARTESIAN_POINT('Ctrl Pts',(13.2650134187968,10.9313419445386,5.22363393386393));
#13986=CARTESIAN_POINT('Ctrl Pts',(14.8415700592552,11.9627725820722,5.11249278633491));
#13987=CARTESIAN_POINT('Ctrl Pts',(16.5631472039009,11.1975587976537,5.0013516388059));
#13988=CARTESIAN_POINT('Ctrl Pts',(16.8538811983444,9.33614703638862,4.89021049127687));
#13989=CARTESIAN_POINT('Ctrl Pts',(15.4476456385435,8.08240003201331,4.77906934374786));
#13990=CARTESIAN_POINT('Ctrl Pts',(13.6316529592416,8.58394822448031,4.66792819621882));
#13991=CARTESIAN_POINT('Ctrl Pts',(13.0681910623456,10.381694227493,4.55678704868982));
#13992=CARTESIAN_POINT('Ctrl Pts',(14.2730306913416,11.8300524252543,4.44564590116079));
#13993=CARTESIAN_POINT('Ctrl Pts',(16.1433092841637,11.6032529855428,4.33450475363178));
#13994=CARTESIAN_POINT('Ctrl Pts',(16.9670477599216,9.90889914877423,4.22336360610275));
#13995=CARTESIAN_POINT('Ctrl Pts',(15.9902284850769,8.29793542947089,4.11222245857374));
#13996=CARTESIAN_POINT('Ctrl Pts',(14.106993204479,8.24497432552685,4.00108131104471));
#13997=CARTESIAN_POINT('Ctrl Pts',(13.0411810387533,9.79849433763074,3.8899401635157));
#13998=CARTESIAN_POINT('Ctrl Pts',(13.7683943066552,11.536464666379,3.77879901598667));
#13999=CARTESIAN_POINT('Ctrl Pts',(15.622970733716,11.8680159848985,3.66765786845765));
#14000=CARTESIAN_POINT('Ctrl Pts',(16.907304380784,10.4896593243745,3.55651672092864));
#14001=CARTESIAN_POINT('Ctrl Pts',(16.4457670045134,8.66308787738691,3.44537557339961));
#14002=CARTESIAN_POINT('Ctrl Pts',(14.6608316718731,8.06027293155299,3.3342344258706));
#14003=CARTESIAN_POINT('Ctrl Pts',(13.1863576175239,9.23300745545514,3.22309327834157));
#14004=CARTESIAN_POINT('Ctrl Pts',(13.3720200962339,11.1078166310327,3.11195213081256));
#14005=CARTESIAN_POINT('Ctrl Pts',(15.0478710154155,11.9685742608536,3.00081098328353));
#14006=CARTESIAN_POINT('Ctrl Pts',(16.6799026995687,11.0273768417383,2.88966983575452));
#14007=CARTESIAN_POINT('Ctrl Pts',(16.7742178691174,9.14575927935223,2.77852868822549));
#14008=CARTESIAN_POINT('Ctrl Pts',(15.2444841459064,8.04607990055583,2.66738754069648));
#14009=CARTESIAN_POINT('Ctrl Pts',(13.490959302405,8.73494172901969,2.55624639316745));
#14010=CARTESIAN_POINT('Ctrl Pts',(13.118750650409,10.5817878874212,2.44510524563844));
#14011=CARTESIAN_POINT('Ctrl Pts',(14.468563280039,11.8960884077944,2.33396409810942));
#14012=CARTESIAN_POINT('Ctrl Pts',(16.304832065112,11.4747845772875,2.2228229505804));
#14013=CARTESIAN_POINT('Ctrl Pts',(16.946709179381,9.70352122397884,2.11168180305138));
#14014=CARTESIAN_POINT('Ctrl Pts',(15.8066456484325,8.20364287411109,2.00054065552236));
#14015=CARTESIAN_POINT('Ctrl Pts',(13.9282106348881,8.34807871336868,1.88939950799334));
#14016=CARTESIAN_POINT('Ctrl Pts',(13.0308491301998,10.0046181888745,1.77825836046432));
#14017=CARTESIAN_POINT('Ctrl Pts',(13.9359706772179,11.6569299683187,1.6671172129353));
#14018=CARTESIAN_POINT('Ctrl Pts',(15.8150622164002,11.7925543157533,1.55597606540628));
#14019=CARTESIAN_POINT('Ctrl Pts',(16.9480787683183,10.2873438536559,1.44483491787726));
#14020=CARTESIAN_POINT('Ctrl Pts',(16.2978995977724,8.51911301545824,1.33369377034824));
#14021=CARTESIAN_POINT('Ctrl Pts',(14.4596772331612,8.10642209645783,1.22255262281922));
#14022=CARTESIAN_POINT('Ctrl Pts',(13.1160395720428,9.42704814205063,1.1114114752902));
#14023=CARTESIAN_POINT('Ctrl Pts',(13.4969152573589,11.2721110952926,1.00027032776118));
#14024=CARTESIAN_POINT('Ctrl Pts',(15.2536350318509,11.952773707662,0.88912918023216));
#14025=CARTESIAN_POINT('Ctrl Pts',(16.7782265823633,10.8458672294876,0.777988032703139));
#14026=CARTESIAN_POINT('Ctrl Pts',(16.6750237516355,8.96483701197515,0.666846885174121));
#14027=CARTESIAN_POINT('Ctrl Pts',(15.0387178247449,8.0310640069849,0.555705737645099));
#14028=CARTESIAN_POINT('Ctrl Pts',(13.3666853215027,8.90013938368058,0.44456459011608));
#14029=CARTESIAN_POINT('Ctrl Pts',(13.1902797174549,10.7748927805024,0.33342344258706));
#14030=CARTESIAN_POINT('Ctrl Pts',(14.6693309261205,11.9424683302957,0.222282295058039));
#14031=CARTESIAN_POINT('Ctrl Pts',(16.4533106153496,11.3277177342173,0.111141147529021));
#14032=CARTESIAN_POINT('Ctrl Pts',(16.7519852444706,10.1141081409362,0.0370470491763399));
#14033=CARTESIAN_POINT('Ctrl Pts',(16.6117095221421,9.57816067485776,0.));
#14034=CARTESIAN_POINT('Ctrl Pts',(13.3361815072522,10.0009395500142,7.3785196366098));
#14035=CARTESIAN_POINT('Ctrl Pts',(13.3350652939176,10.2169537828321,7.36411833671163));
#14036=CARTESIAN_POINT('Ctrl Pts',(13.3741036482068,10.4325813967082,7.34971703681347));
#14037=CARTESIAN_POINT('Ctrl Pts',(13.4551685667619,10.6310402268794,7.33531573691531));
#14038=CARTESIAN_POINT('Ctrl Pts',(13.6637064102501,11.1415715048073,7.29826868773897));
#14039=CARTESIAN_POINT('Ctrl Pts',(14.1503613856775,11.5384857653495,7.26122163856263));
#14040=CARTESIAN_POINT('Ctrl Pts',(14.6923890664536,11.6401414669966,7.22417458938629));
#14041=CARTESIAN_POINT('Ctrl Pts',(15.2344167472297,11.7417971686436,7.18712754020995));
#14042=CARTESIAN_POINT('Ctrl Pts',(15.8318171333545,11.5481943113955,7.15008049103361));
#14043=CARTESIAN_POINT('Ctrl Pts',(16.2111781034228,11.147931667852,7.11303344185727));
#14044=CARTESIAN_POINT('Ctrl Pts',(16.5905390734911,10.7476690243085,7.07598639268093));
#14045=CARTESIAN_POINT('Ctrl Pts',(16.7518606275029,10.1407465944695,7.03893934350459));
#14046=CARTESIAN_POINT('Ctrl Pts',(16.6213058662152,9.60494564230069,7.00189229432825));
#14047=CARTESIAN_POINT('Ctrl Pts',(16.4907511049275,9.06914469013187,6.9648452451519));
#14048=CARTESIAN_POINT('Ctrl Pts',(16.0683200283403,8.60446521563324,6.92779819597557));
#14049=CARTESIAN_POINT('Ctrl Pts',(15.5473526477042,8.42357931770721,6.89075114679923));
#14050=CARTESIAN_POINT('Ctrl Pts',(15.0263852670682,8.24269341978119,6.85370409762289));
#14051=CARTESIAN_POINT('Ctrl Pts',(14.4068815823831,8.34560109842778,6.81665704844655));
#14052=CARTESIAN_POINT('Ctrl Pts',(13.9723753281766,8.68520483913655,6.77960999927021));
#14053=CARTESIAN_POINT('Ctrl Pts',(13.5771626118018,8.99409732470422,6.74591321171674));
#14054=CARTESIAN_POINT('Ctrl Pts',(13.3350006419844,9.49881149769819,6.71221642416327));
#14055=CARTESIAN_POINT('Ctrl Pts',(13.3318213113649,10.0008675364682,6.6785196366098));
#14056=CARTESIAN_POINT('Ctrl Pts',(14.4698297828114,8.01482567432828,8.));
#14057=CARTESIAN_POINT('Ctrl Pts',(14.3998214936988,8.04074714826579,8.));
#14058=CARTESIAN_POINT('Ctrl Pts',(14.3314995809058,8.07074117787574,8.));
#14059=CARTESIAN_POINT('Ctrl Pts',(14.2650833692488,8.10452090745416,8.));
#14060=CARTESIAN_POINT('Ctrl Pts',(14.2004102705822,8.13741407810413,8.));
#14061=CARTESIAN_POINT('Ctrl Pts',(14.1375437306998,8.1738977671453,8.));
#14062=CARTESIAN_POINT('Ctrl Pts',(14.0767171887106,8.21374090711945,8.));
#14063=CARTESIAN_POINT('Ctrl Pts',(14.0631405149643,8.22263402013834,8.));
#14064=CARTESIAN_POINT('Ctrl Pts',(14.0496638268926,8.23169584191256,8.));
#14065=CARTESIAN_POINT('Ctrl Pts',(14.036295680768,8.240920018892,8.));
#14066=CARTESIAN_POINT('Ctrl Pts',(13.9749539654965,8.28324651896258,8.));
#14067=CARTESIAN_POINT('Ctrl Pts',(13.9160153999523,8.32890389170504,8.));
#14068=CARTESIAN_POINT('Ctrl Pts',(13.8597185778864,8.37762279724655,8.));
#14069=CARTESIAN_POINT('Ctrl Pts',(13.8201934931154,8.41182754985629,8.));
#14070=CARTESIAN_POINT('Ctrl Pts',(13.7819713009793,8.44754226231406,8.));
#14071=CARTESIAN_POINT('Ctrl Pts',(13.7451474325163,8.48468212230948,8.));
#14072=CARTESIAN_POINT('Ctrl Pts',(13.7311387285853,8.49881103717989,8.));
#14073=CARTESIAN_POINT('Ctrl Pts',(13.7173325138727,8.51314626010991,8.));
#14074=CARTESIAN_POINT('Ctrl Pts',(13.7037345023968,8.52768330428626,8.));
#14075=CARTESIAN_POINT('Ctrl Pts',(13.6908096643821,8.54150068791797,8.));
#14076=CARTESIAN_POINT('Ctrl Pts',(13.6780691038482,8.55550494493883,8.));
#14077=CARTESIAN_POINT('Ctrl Pts',(13.6655397272255,8.56966702391835,8.));
#14078=CARTESIAN_POINT('Ctrl Pts',(13.6174406383793,8.62403390230305,8.));
#14079=CARTESIAN_POINT('Ctrl Pts',(13.5723959858275,8.68077902345639,8.));
#14080=CARTESIAN_POINT('Ctrl Pts',(13.5306283225234,8.73965444066073,8.));
#14081=CARTESIAN_POINT('Ctrl Pts',(13.4897585658688,8.79726417469265,8.));
#14082=CARTESIAN_POINT('Ctrl Pts',(13.4520260621303,8.85691446263185,8.));
#14083=CARTESIAN_POINT('Ctrl Pts',(13.4176844468098,8.91839214182768,8.));
#14084=CARTESIAN_POINT('Ctrl Pts',(13.3840956014734,8.97852222711571,8.));
#14085=CARTESIAN_POINT('Ctrl Pts',(13.3537503389223,9.0404011858163,8.));
#14086=CARTESIAN_POINT('Ctrl Pts',(13.3269342184203,9.10383656685819,8.));
#14087=CARTESIAN_POINT('Ctrl Pts',(13.318222609287,9.12444447861096,8.));
#14088=CARTESIAN_POINT('Ctrl Pts',(13.3098838590006,9.1452166622322,8.));
#14089=CARTESIAN_POINT('Ctrl Pts',(13.3019289624212,9.16614649473232,8.));
#14090=CARTESIAN_POINT('Ctrl Pts',(13.2974345589444,9.17797155254661,8.));
#14091=CARTESIAN_POINT('Ctrl Pts',(13.2930623430191,9.18984821638012,8.));
#14092=CARTESIAN_POINT('Ctrl Pts',(13.2888201205526,9.20175830442571,8.));
#14093=CARTESIAN_POINT('Ctrl Pts',(13.2659037845155,9.26609617968757,8.));
#14094=CARTESIAN_POINT('Ctrl Pts',(13.2467332556311,9.3315197201952,8.));
#14095=CARTESIAN_POINT('Ctrl Pts',(13.2315368288626,9.39782942737589,8.));
#14096=CARTESIAN_POINT('Ctrl Pts',(13.2293394455293,9.40741772386231,8.));
#14097=CARTESIAN_POINT('Ctrl Pts',(13.2272252438361,9.41702456272481,8.));
#14098=CARTESIAN_POINT('Ctrl Pts',(13.2251950049826,9.42664935181928,8.));
#14099=CARTESIAN_POINT('Ctrl Pts',(13.2108763834671,9.49452989305377,8.));
#14100=CARTESIAN_POINT('Ctrl Pts',(13.2007298389188,9.56330380603441,8.));
#14101=CARTESIAN_POINT('Ctrl Pts',(13.1946587081026,9.63261524468971,8.));
#14102=CARTESIAN_POINT('Ctrl Pts',(13.1889946919687,9.69727883351621,8.));
#14103=CARTESIAN_POINT('Ctrl Pts',(13.1868786273274,9.76241098193826,8.));
#14104=CARTESIAN_POINT('Ctrl Pts',(13.1882701725515,9.82771039931623,8.));
#14105=CARTESIAN_POINT('Ctrl Pts',(13.1885789791415,9.84220140547489,8.));
#14106=CARTESIAN_POINT('Ctrl Pts',(13.1890606579093,9.85670057589872,8.));
#14107=CARTESIAN_POINT('Ctrl Pts',(13.1897149907357,9.87120447799809,8.));
#14108=CARTESIAN_POINT('Ctrl Pts',(13.1902222155533,9.8824475928177,8.));
#14109=CARTESIAN_POINT('Ctrl Pts',(13.1908332280675,9.89369266287328,8.));
#14110=CARTESIAN_POINT('Ctrl Pts',(13.1915468679667,9.90492535693582,8.));
#14111=CARTESIAN_POINT('Ctrl Pts',(13.1958826255629,9.97317019394023,8.));
#14112=CARTESIAN_POINT('Ctrl Pts',(13.2040074350011,10.0410843826852,8.));
#14113=CARTESIAN_POINT('Ctrl Pts',(13.2158110352946,10.1083321091977,8.));
#14114=CARTESIAN_POINT('Ctrl Pts',(13.2275596947567,10.1752668256192,8.));
#14115=CARTESIAN_POINT('Ctrl Pts',(13.2429534648895,10.2415422967115,8.));
#14116=CARTESIAN_POINT('Ctrl Pts',(13.2619307505069,10.306807573732,8.));
#14117=CARTESIAN_POINT('Ctrl Pts',(13.2805005504678,10.3706714562232,8.));
#14118=CARTESIAN_POINT('Ctrl Pts',(13.3025021612721,10.4335688734512,8.));
#14119=CARTESIAN_POINT('Ctrl Pts',(13.3279154052132,10.4951385987467,8.));
#14120=CARTESIAN_POINT('Ctrl Pts',(13.3333017419517,10.5081883012605,8.));
#14121=CARTESIAN_POINT('Ctrl Pts',(13.3388414595185,10.5211782174638,8.));
#14122=CARTESIAN_POINT('Ctrl Pts',(13.344534554462,10.5341046634128,8.));
#14123=CARTESIAN_POINT('Ctrl Pts',(13.3498584076977,10.546192728301,8.));
#14124=CARTESIAN_POINT('Ctrl Pts',(13.3553171624044,10.5582266610946,8.));
#14125=CARTESIAN_POINT('Ctrl Pts',(13.3609016527936,10.5701845006962,8.));
#14126=CARTESIAN_POINT('Ctrl Pts',(13.3885543554232,10.6293960955872,8.));
#14127=CARTESIAN_POINT('Ctrl Pts',(13.419333021235,10.6868524927592,8.));
#14128=CARTESIAN_POINT('Ctrl Pts',(13.4531736194346,10.7422401797738,8.));
#14129=CARTESIAN_POINT('Ctrl Pts',(13.4863693140172,10.7965723381752,8.));
#14130=CARTESIAN_POINT('Ctrl Pts',(13.5225118662568,10.8489145978588,8.));
#14131=CARTESIAN_POINT('Ctrl Pts',(13.5615753972507,10.8989353051115,8.));
#14132=CARTESIAN_POINT('Ctrl Pts',(13.5993684169907,10.9473291273931,8.));
#14133=CARTESIAN_POINT('Ctrl Pts',(13.6398959829063,10.9935504147084,8.));
#14134=CARTESIAN_POINT('Ctrl Pts',(13.6831600007655,11.0372567515148,8.));
#14135=CARTESIAN_POINT('Ctrl Pts',(13.6903680308745,11.0445384744625,8.));
#14136=CARTESIAN_POINT('Ctrl Pts',(13.6976520674348,11.0517502824926,8.));
#14137=CARTESIAN_POINT('Ctrl Pts',(13.7050121765453,11.0588904602709,8.));
#14138=CARTESIAN_POINT('Ctrl Pts',(13.7127728136493,11.0664191976529,8.));
#14139=CARTESIAN_POINT('Ctrl Pts',(13.7206180292613,11.0738682961014,8.));
#14140=CARTESIAN_POINT('Ctrl Pts',(13.7285463279864,11.0812370110871,8.));
#14141=CARTESIAN_POINT('Origin',(-15.,10.,9.54592528053767));
#14142=CARTESIAN_POINT('Ctrl Pts',(-17.056546936061,10.0014880949897,7.79592528053768));
#14143=CARTESIAN_POINT('Ctrl Pts',(-17.0573685174097,10.0998546456676,7.79057696270225));
#14144=CARTESIAN_POINT('Ctrl Pts',(-17.0062396152572,10.8787654055349,7.74818159569048));
#14145=CARTESIAN_POINT('Ctrl Pts',(-16.0106087131083,12.2086083874229,7.66873917950237));
#14146=CARTESIAN_POINT('Ctrl Pts',(-13.6926512300581,12.0466287931598,7.55759803197335));
#14147=CARTESIAN_POINT('Ctrl Pts',(-12.5713806281451,10.011647112944,7.44645688444433));
#14148=CARTESIAN_POINT('Ctrl Pts',(-13.673176561786,7.96579721763555,7.33531573691531));
#14149=CARTESIAN_POINT('Ctrl Pts',(-15.989491953976,7.78208289239259,7.22417458938629));
#14150=CARTESIAN_POINT('Ctrl Pts',(-17.0022525717684,9.10777352753874,7.14437777059374));
#14151=CARTESIAN_POINT('Ctrl Pts',(-17.0572654529527,9.89346180187816,7.10162800097754));
#14152=CARTESIAN_POINT('Ctrl Pts',(-17.0563655762952,9.99839712210779,7.09592528053768));
#14153=CARTESIAN_POINT('Ctrl Pts',(-17.052688542414,9.99752997529134,7.85407471946233));
#14154=CARTESIAN_POINT('Ctrl Pts',(-17.0491243489968,10.4678340862227,7.82862238128887));
#14155=CARTESIAN_POINT('Ctrl Pts',(-16.6564410380322,11.6297982528173,7.76612299393908));
#14156=CARTESIAN_POINT('Ctrl Pts',(-14.7276622354211,12.4126888235087,7.66657655741294));
#14157=CARTESIAN_POINT('Ctrl Pts',(-12.8251333276493,11.0807508020576,7.55543540988392));
#14158=CARTESIAN_POINT('Ctrl Pts',(-12.9125602025977,8.75827697936691,7.4442942623549));
#14159=CARTESIAN_POINT('Ctrl Pts',(-14.9111754557965,7.5730758609676,7.33315311482589));
#14160=CARTESIAN_POINT('Ctrl Pts',(-16.7213954228828,8.4748124655939,7.23641326719502));
#14161=CARTESIAN_POINT('Ctrl Pts',(-17.0498947507887,9.58221923747805,7.1767204687405));
#14162=CARTESIAN_POINT('Ctrl Pts',(-17.0520595406494,10.0011587933795,7.15407471946232));
#14163=CARTESIAN_POINT('Ctrl Pts',(-13.7309291201476,11.0793586530485,8.));
#14164=CARTESIAN_POINT('Ctrl Pts',(-13.3720061708544,10.657350026192,7.96295295082366));
#14165=CARTESIAN_POINT('Ctrl Pts',(-13.114537813302,9.43433491073641,7.88885885247098));
#14166=CARTESIAN_POINT('Ctrl Pts',(-14.4551167789601,8.1064248597425,7.77771770494196));
#14167=CARTESIAN_POINT('Ctrl Pts',(-16.2942884601245,8.51663726829463,7.66657655741294));
#14168=CARTESIAN_POINT('Ctrl Pts',(-16.9487772812347,10.2822716397578,7.55543540988393));
#14169=CARTESIAN_POINT('Ctrl Pts',(-15.8194058235982,11.790749031973,7.4442942623549));
#14170=CARTESIAN_POINT('Ctrl Pts',(-13.9399960818965,11.659415291108,7.33315311482589));
#14171=CARTESIAN_POINT('Ctrl Pts',(-13.0308651303028,10.0094435284899,7.22201196729686));
#14172=CARTESIAN_POINT('Ctrl Pts',(-13.9242059384039,8.3506597710577,7.11087081976784));
#14173=CARTESIAN_POINT('Ctrl Pts',(-15.8022842658834,8.20170341828741,6.99972967223882));
#14174=CARTESIAN_POINT('Ctrl Pts',(-16.9459842407539,9.69879198933349,6.8885885247098));
#14175=CARTESIAN_POINT('Ctrl Pts',(-16.3084066898541,11.4716175152832,6.77744737718078));
#14176=CARTESIAN_POINT('Ctrl Pts',(-14.4731656357203,11.8973706549213,6.66630622965176));
#14177=CARTESIAN_POINT('Ctrl Pts',(-13.1201677999229,10.5863518488495,6.55516508212274));
#14178=CARTESIAN_POINT('Ctrl Pts',(-13.4878941064161,8.73860657507213,6.44402393459372));
#14179=CARTESIAN_POINT('Ctrl Pts',(-15.2397423309735,8.0454926065714,6.3328827870647));
#14180=CARTESIAN_POINT('Ctrl Pts',(-16.7721399220139,9.14145658964824,6.22174163953569));
#14181=CARTESIAN_POINT('Ctrl Pts',(-16.6823906822222,11.023297702524,6.11060049200666));
#14182=CARTESIAN_POINT('Ctrl Pts',(-15.0526475313575,11.9684523308575,5.99945934447764));
#14183=CARTESIAN_POINT('Ctrl Pts',(-13.3747129092986,11.111763635759,5.88831819694862));
#14184=CARTESIAN_POINT('Ctrl Pts',(-13.1845018342894,9.23741040317065,5.77717704941961));
#14185=CARTESIAN_POINT('Ctrl Pts',(-14.6561260023258,8.06110156877586,5.66603590189058));
#14186=CARTESIAN_POINT('Ctrl Pts',(-16.4425188328326,8.6595836864797,5.55489475436157));
#14187=CARTESIAN_POINT('Ctrl Pts',(-16.908486954743,10.4850299113492,5.44375360683254));
#14188=CARTESIAN_POINT('Ctrl Pts',(-15.6275015719515,11.8664989271813,5.33261245930353));
#14189=CARTESIAN_POINT('Ctrl Pts',(-13.7721260589331,11.5394486208087,5.2214713117745));
#14190=CARTESIAN_POINT('Ctrl Pts',(-13.0406978065988,9.80324790916912,5.11033016424548));
#14191=CARTESIAN_POINT('Ctrl Pts',(-14.1027373194897,8.24714628330515,4.99918901671647));
#14192=CARTESIAN_POINT('Ctrl Pts',(-15.9860956161181,8.2955376489092,4.88804786918745));
#14193=CARTESIAN_POINT('Ctrl Pts',(-16.9668209718389,9.90412646355499,4.77690672165843));
#14194=CARTESIAN_POINT('Ctrl Pts',(-16.1471961698029,11.6004741229444,4.66576557412941));
#14195=CARTESIAN_POINT('Ctrl Pts',(-14.2774733492598,11.8318110462748,4.55462442660038));
#14196=CARTESIAN_POINT('Ctrl Pts',(-13.0691228591274,10.3863805599598,4.44348327907137));
#14197=CARTESIAN_POINT('Ctrl Pts',(-13.6282209649552,8.58727258493754,4.33234213154234));
#14198=CARTESIAN_POINT('Ctrl Pts',(-15.442991365066,8.0813194323332,4.22120098401333));
#14199=CARTESIAN_POINT('Ctrl Pts',(-16.8522649836184,9.3316506147811,4.11005983648431));
#14200=CARTESIAN_POINT('Ctrl Pts',(-16.5660484669655,11.1937624007216,3.99891868895529));
#14201=CARTESIAN_POINT('Ctrl Pts',(-14.846333098649,11.9631512814075,3.88777754142627));
#14202=CARTESIAN_POINT('Ctrl Pts',(-13.2672783364837,10.9355490938709,3.77663639389725));
#14203=CARTESIAN_POINT('Ctrl Pts',(-13.2742884805443,9.05158225349828,3.66549524636823));
#14204=CARTESIAN_POINT('Ctrl Pts',(-14.8609467221099,8.03575952180664,3.5543540988392));
#14205=CARTESIAN_POINT('Ctrl Pts',(-16.5748888366715,8.8179248660152,3.44321295131019));
#14206=CARTESIAN_POINT('Ctrl Pts',(-16.8472399746527,10.6821150535684,3.33207180378116));
#14207=CARTESIAN_POINT('Ctrl Pts',(-15.4287006719665,11.921924089068,3.22093065625215));
#14208=CARTESIAN_POINT('Ctrl Pts',(-13.6177457231939,11.4024797982418,3.10978950872313));
#14209=CARTESIAN_POINT('Ctrl Pts',(-13.0720516908598,9.59926094832275,2.99864836119411));
#14210=CARTESIAN_POINT('Ctrl Pts',(-14.2911253177228,8.16286278268615,2.88750721366509));
#14211=CARTESIAN_POINT('Ctrl Pts',(-16.1590748027858,8.40810739322197,2.77636606613607));
#14212=CARTESIAN_POINT('Ctrl Pts',(-16.9660530383818,10.1105075589387,2.66522491860705));
#14213=CARTESIAN_POINT('Ctrl Pts',(-15.9733840520667,11.7117534747863,2.55408377107803));
#14214=CARTESIAN_POINT('Ctrl Pts',(-14.08971778817,11.7461279342581,2.44294262354901));
#14215=CARTESIAN_POINT('Ctrl Pts',(-13.039287871942,10.1821659194628,2.33180147601999));
#14216=CARTESIAN_POINT('Ctrl Pts',(-13.7836163199646,8.45145641986686,2.22066032849097));
#14217=CARTESIAN_POINT('Ctrl Pts',(-15.6413742968694,8.13822249874073,2.10951918096195));
#14218=CARTESIAN_POINT('Ctrl Pts',(-16.9120436018175,9.52918607960339,1.99837803343293));
#14219=CARTESIAN_POINT('Ctrl Pts',(-16.4325037837013,11.351114139767,1.88723688590391));
#14220=CARTESIAN_POINT('Ctrl Pts',(-14.6417066452378,11.9362856745195,1.77609573837489));
#14221=CARTESIAN_POINT('Ctrl Pts',(-13.1788770626978,10.7490579702873,1.66495459084587));
#14222=CARTESIAN_POINT('Ctrl Pts',(-13.3830314476372,8.87617199210746,1.55381344331685));
#14223=CARTESIAN_POINT('Ctrl Pts',(-15.0672948586319,8.03199417220646,1.44267229578783));
#14224=CARTESIAN_POINT('Ctrl Pts',(-16.6899593301811,8.98925024452329,1.33153114825881));
#14225=CARTESIAN_POINT('Ctrl Pts',(-16.7657016246685,10.8717083019789,1.22039000072979));
#14226=CARTESIAN_POINT('Ctrl Pts',(-15.22519088697,11.9562359044779,1.10924885320077));
#14227=CARTESIAN_POINT('Ctrl Pts',(-13.4785484877468,11.2501085845661,0.998107705671749));
#14228=CARTESIAN_POINT('Ctrl Pts',(-13.1245842530937,9.39966950168421,0.886966558142732));
#14229=CARTESIAN_POINT('Ctrl Pts',(-14.4872983423832,8.09877206801491,0.77582541061371));
#14230=CARTESIAN_POINT('Ctrl Pts',(-16.3193252756259,8.53813924368035,0.664684263084692));
#14231=CARTESIAN_POINT('Ctrl Pts',(-16.9436823523983,10.315721757665,0.553543115555671));
#14232=CARTESIAN_POINT('Ctrl Pts',(-15.7888920442232,11.8041387854927,0.442401968026653));
#14233=CARTESIAN_POINT('Ctrl Pts',(-13.9119373633139,11.6414407384693,0.331260820497631));
#14234=CARTESIAN_POINT('Ctrl Pts',(-13.0310370233095,9.97560805685666,0.220119672968611));
#14235=CARTESIAN_POINT('Ctrl Pts',(-13.9522834796021,8.33331535535093,0.108978525439592));
#14236=CARTESIAN_POINT('Ctrl Pts',(-15.8328831148959,8.21427038628653,-0.00216262208942864));
#14237=CARTESIAN_POINT('Ctrl Pts',(-16.9505144549114,9.73459839514212,-0.113303769618448));
#14238=CARTESIAN_POINT('Ctrl Pts',(-16.5058833578897,10.9026562341787,-0.187397867971127));
#14239=CARTESIAN_POINT('Ctrl Pts',(-16.0856682637067,11.2636773406135,-0.224444917147467));
#14240=CARTESIAN_POINT('Ctrl Pts',(-13.6322193753412,11.1633123698098,8.07481497238249));
#14241=CARTESIAN_POINT('Ctrl Pts',(-13.2453789997699,10.7084794424949,8.03776792320615));
#14242=CARTESIAN_POINT('Ctrl Pts',(-12.9678844669477,9.3903368508222,7.96367382485348));
#14243=CARTESIAN_POINT('Ctrl Pts',(-14.412735155875,7.95914047883512,7.85253267732443));
#14244=CARTESIAN_POINT('Ctrl Pts',(-16.3949596563776,8.40125966486316,7.74139152979544));
#14245=CARTESIAN_POINT('Ctrl Pts',(-17.1003553460767,10.3042270419099,7.6302503822664));
#14246=CARTESIAN_POINT('Ctrl Pts',(-15.8831401201015,11.9300354837897,7.51910923473739));
#14247=CARTESIAN_POINT('Ctrl Pts',(-13.8575477979503,11.7884864584586,7.40796808720837));
#14248=CARTESIAN_POINT('Ctrl Pts',(-12.8777036295836,10.0101780566413,7.29682693967935));
#14249=CARTESIAN_POINT('Ctrl Pts',(-13.8405294795313,8.22237225325032,7.18568579215033));
#14250=CARTESIAN_POINT('Ctrl Pts',(-15.864686828581,8.0618299096558,7.07454464462131));
#14251=CARTESIAN_POINT('Ctrl Pts',(-17.0973450598001,9.67536369518652,6.96340349709229));
#14252=CARTESIAN_POINT('Ctrl Pts',(-16.4101760177214,11.5860815627155,6.85226234956327));
#14253=CARTESIAN_POINT('Ctrl Pts',(-14.4321878727924,12.0449502551816,6.74112120203426));
#14254=CARTESIAN_POINT('Ctrl Pts',(-12.973952360191,10.6319589479372,6.62998005450522));
#14255=CARTESIAN_POINT('Ctrl Pts',(-13.3702808278786,8.64049399125046,6.51883890697622));
#14256=CARTESIAN_POINT('Ctrl Pts',(-15.2583897561767,7.89346884722859,6.40769775944719));
#14257=CARTESIAN_POINT('Ctrl Pts',(-16.9099789365563,9.07467812810877,6.29655661191818));
#14258=CARTESIAN_POINT('Ctrl Pts',(-16.8132489010525,11.1028909361887,6.18541546438915));
#14259=CARTESIAN_POINT('Ctrl Pts',(-15.056742514914,12.1215607429465,6.07427431686013));
#14260=CARTESIAN_POINT('Ctrl Pts',(-13.2482962713414,11.1982378481243,5.96313316933111));
#14261=CARTESIAN_POINT('Ctrl Pts',(-13.0432903673187,9.17809533599028,5.85199202180209));
#14262=CARTESIAN_POINT('Ctrl Pts',(-14.6293791002458,7.91029189187743,5.74085087427308));
#14263=CARTESIAN_POINT('Ctrl Pts',(-16.5547195523731,8.55532461447468,5.62970972674405));
#14264=CARTESIAN_POINT('Ctrl Pts',(-17.0569311931696,10.5227560774231,5.51856857921503));
#14265=CARTESIAN_POINT('Ctrl Pts',(-15.6763093422789,12.0116772901148,5.40742743168601));
#14266=CARTESIAN_POINT('Ctrl Pts',(-13.6766206578547,11.6591886470871,5.296286284157));
#14267=CARTESIAN_POINT('Ctrl Pts',(-12.8883011023801,9.78794431266843,5.18514513662797));
#14268=CARTESIAN_POINT('Ctrl Pts',(-14.0329472300443,8.11080737126729,5.07400398909896));
#14269=CARTESIAN_POINT('Ctrl Pts',(-16.0627952301169,8.16296267112078,4.96286284156994));
#14270=CARTESIAN_POINT('Ctrl Pts',(-17.1198024950087,9.89666931323625,4.85172169404091));
#14271=CARTESIAN_POINT('Ctrl Pts',(-16.2364263640828,11.7249607806665,4.7405805465119));
#14272=CARTESIAN_POINT('Ctrl Pts',(-14.2212744225941,11.9742913472431,4.62943939898287));
#14273=CARTESIAN_POINT('Ctrl Pts',(-12.9189370871157,10.4164336697406,4.51829825145386));
#14274=CARTESIAN_POINT('Ctrl Pts',(-13.5215224655807,8.47738907501246,4.40715710392483));
#14275=CARTESIAN_POINT('Ctrl Pts',(-15.4774477262444,7.9320823233535,4.29601595639582));
#14276=CARTESIAN_POINT('Ctrl Pts',(-16.9963362145871,9.27966565609687,4.18487480886679));
#14277=CARTESIAN_POINT('Ctrl Pts',(-16.6878574588688,11.2866145682447,4.07373366133778));
#14278=CARTESIAN_POINT('Ctrl Pts',(-14.8343807161159,12.1158473719732,3.96259251380876));
#14279=CARTESIAN_POINT('Ctrl Pts',(-13.1325053179379,11.0083171431391,3.85145136627974));
#14280=CARTESIAN_POINT('Ctrl Pts',(-13.140060718802,8.97781326611282,3.74031021875072));
#14281=CARTESIAN_POINT('Ctrl Pts',(-14.8501310034664,7.8829787123033,3.6291690712217));
#14282=CARTESIAN_POINT('Ctrl Pts',(-16.697385442365,8.72598174710033,3.51802792369268));
#14283=CARTESIAN_POINT('Ctrl Pts',(-16.990920354834,10.7351707212503,3.40688677616366));
#14284=CARTESIAN_POINT('Ctrl Pts',(-15.4620454871379,12.0714134827505,3.29574562863464));
#14285=CARTESIAN_POINT('Ctrl Pts',(-13.5102324478621,11.5115662371307,3.18460448110562));
#14286=CARTESIAN_POINT('Ctrl Pts',(-12.9220937266384,9.56809101908315,3.0734633335766));
#14287=CARTESIAN_POINT('Ctrl Pts',(-14.2359882563512,8.0199682062094,2.96232218604758));
#14288=CARTESIAN_POINT('Ctrl Pts',(-16.2492289303534,8.28428821537383,2.85118103851856));
#14289=CARTESIAN_POINT('Ctrl Pts',(-17.118974830833,10.1191029598066,2.74003989098954));
#14290=CARTESIAN_POINT('Ctrl Pts',(-16.0490949464727,11.8448955642867,2.62889874346052));
#14291=CARTESIAN_POINT('Ctrl Pts',(-14.018915025095,11.881943707456,2.5177575959315));
#14292=CARTESIAN_POINT('Ctrl Pts',(-12.8867815014373,10.1963349873281,2.40661644840248));
#14293=CARTESIAN_POINT('Ctrl Pts',(-13.6890046441715,8.33100897753458,2.29547530087345));
#14294=CARTESIAN_POINT('Ctrl Pts',(-15.6912611031735,7.99341137356774,2.18433415334444));
#14295=CARTESIAN_POINT('Ctrl Pts',(-17.0607644802102,9.49256564912037,2.07319300581542));
#14296=CARTESIAN_POINT('Ctrl Pts',(-16.5439255215792,11.4562053005982,1.9620518582864));
#14297=CARTESIAN_POINT('Ctrl Pts',(-14.6138381895228,12.0868921282949,1.85091071075738));
#14298=CARTESIAN_POINT('Ctrl Pts',(-13.0372280947354,10.807320532502,1.73976956322836));
#14299=CARTESIAN_POINT('Ctrl Pts',(-13.2572618348459,8.78875939945676,1.62862841569934));
#14300=CARTESIAN_POINT('Ctrl Pts',(-15.0725291275981,7.87892048962247,1.51748726817032));
#14301=CARTESIAN_POINT('Ctrl Pts',(-16.8214062468694,8.91063300413882,1.4063461206413));
#14302=CARTESIAN_POINT('Ctrl Pts',(-16.9030398612811,10.9395107434343,1.29520497311228));
#14303=CARTESIAN_POINT('Ctrl Pts',(-15.242706484671,12.1083941093329,1.18406382558326));
#14304=CARTESIAN_POINT('Ctrl Pts',(-13.3602082965927,11.3473434209507,1.07292267805424));
#14305=CARTESIAN_POINT('Ctrl Pts',(-12.9787123300025,9.35297512769056,0.961781530525221));
#14306=CARTESIAN_POINT('Ctrl Pts',(-14.4474198371014,7.95089244445364,0.8506403829962));
#14307=CARTESIAN_POINT('Ctrl Pts',(-16.4219438632409,8.42443408781415,0.739499235467181));
#14308=CARTESIAN_POINT('Ctrl Pts',(-17.0948641280075,10.3402789471993,0.628358087938161));
#14309=CARTESIAN_POINT('Ctrl Pts',(-15.8502529450219,11.9444667072335,0.517216940409141));
#14310=CARTESIAN_POINT('Ctrl Pts',(-13.8273066410226,11.7691138251199,0.40607579288012));
#14311=CARTESIAN_POINT('Ctrl Pts',(-12.8778888926195,9.97371082438428,0.294934645351101));
#14312=CARTESIAN_POINT('Ctrl Pts',(-13.8707909231185,8.20367876959515,0.183793497822081));
#14313=CARTESIAN_POINT('Ctrl Pts',(-15.8976656901092,8.07537435040597,0.0726523502930605));
#14314=CARTESIAN_POINT('Ctrl Pts',(-17.1022276390544,9.71395516307158,-0.0384887972359591));
#14315=CARTESIAN_POINT('Ctrl Pts',(-16.6230126406787,10.9728658402285,-0.112582895588638));
#14316=CARTESIAN_POINT('Ctrl Pts',(-16.170112749004,11.361967569938,-0.149629944764978));
#14317=CARTESIAN_POINT('Ctrl Pts',(-13.5335096305347,11.247266086571,8.14962994476498));
#14318=CARTESIAN_POINT('Ctrl Pts',(-13.1187518286854,10.7596088587978,8.11258289558864));
#14319=CARTESIAN_POINT('Ctrl Pts',(-12.8212311205934,9.34633879090798,8.03848879723596));
#14320=CARTESIAN_POINT('Ctrl Pts',(-14.3703535327899,7.81185609792774,7.92734764970693));
#14321=CARTESIAN_POINT('Ctrl Pts',(-16.4956308526308,8.28588206143169,7.81620650217792));
#14322=CARTESIAN_POINT('Ctrl Pts',(-17.2519334109186,10.3261824440619,7.7050653546489));
#14323=CARTESIAN_POINT('Ctrl Pts',(-15.9468744166049,12.0693219356063,7.59392420711988));
#14324=CARTESIAN_POINT('Ctrl Pts',(-13.7750995140042,11.9175576258092,7.48278305959087));
#14325=CARTESIAN_POINT('Ctrl Pts',(-12.7245421288643,10.0109125847927,7.37164191206184));
#14326=CARTESIAN_POINT('Ctrl Pts',(-13.7568530206586,8.09408473544294,7.26050076453282));
#14327=CARTESIAN_POINT('Ctrl Pts',(-15.9270893912785,7.92195640102419,7.1493596170038));
#14328=CARTESIAN_POINT('Ctrl Pts',(-17.2487058788463,9.65193540103954,7.03821846947478));
#14329=CARTESIAN_POINT('Ctrl Pts',(-16.5119453455887,11.7005456101477,6.92707732194576));
#14330=CARTESIAN_POINT('Ctrl Pts',(-14.3912101098645,12.1925298554418,6.81593617441674));
#14331=CARTESIAN_POINT('Ctrl Pts',(-12.8277369204591,10.6775660470248,6.70479502688772));
#14332=CARTESIAN_POINT('Ctrl Pts',(-13.252667549341,8.54238140742879,6.59365387935871));
#14333=CARTESIAN_POINT('Ctrl Pts',(-15.27703718138,7.74144508788578,6.48251273182967));
#14334=CARTESIAN_POINT('Ctrl Pts',(-17.0478179510987,9.0078996665693,6.37137158430067));
#14335=CARTESIAN_POINT('Ctrl Pts',(-16.9441071198828,11.1824841698534,6.26023043677164));
#14336=CARTESIAN_POINT('Ctrl Pts',(-15.0608374984705,12.2746691550355,6.14908928924262));
#14337=CARTESIAN_POINT('Ctrl Pts',(-13.1218796333842,11.2847120604895,6.03794814171361));
#14338=CARTESIAN_POINT('Ctrl Pts',(-12.9020789003479,9.11878026880993,5.92680699418458));
#14339=CARTESIAN_POINT('Ctrl Pts',(-14.6026321981658,7.759482214979,5.81566584665557));
#14340=CARTESIAN_POINT('Ctrl Pts',(-16.6669202719137,8.45106554246967,5.70452469912654));
#14341=CARTESIAN_POINT('Ctrl Pts',(-17.2053754315962,10.5604822434969,5.59338355159752));
#14342=CARTESIAN_POINT('Ctrl Pts',(-15.7251171126062,12.1568556530484,5.4822424040685));
#14343=CARTESIAN_POINT('Ctrl Pts',(-13.5811152567764,11.7789286733654,5.37110125653948));
#14344=CARTESIAN_POINT('Ctrl Pts',(-12.7359043981615,9.77264071616773,5.25996010901047));
#14345=CARTESIAN_POINT('Ctrl Pts',(-13.9631571405989,7.97446845922946,5.14881896148145));
#14346=CARTESIAN_POINT('Ctrl Pts',(-16.1394948441157,8.03038769333235,5.03767781395242));
#14347=CARTESIAN_POINT('Ctrl Pts',(-17.2727840181784,9.88921216291753,4.9265366664234));
#14348=CARTESIAN_POINT('Ctrl Pts',(-16.3256565583627,11.8494474383885,4.81539551889438));
#14349=CARTESIAN_POINT('Ctrl Pts',(-14.1650754959284,12.1167716482113,4.70425437136536));
#14350=CARTESIAN_POINT('Ctrl Pts',(-12.7687513151041,10.4464867795214,4.59311322383634));
#14351=CARTESIAN_POINT('Ctrl Pts',(-13.4148239662062,8.36750556508739,4.48197207630732));
#14352=CARTESIAN_POINT('Ctrl Pts',(-15.5119040874227,7.78284521437382,4.3708309287783));
#14353=CARTESIAN_POINT('Ctrl Pts',(-17.1404074455559,9.22768069741262,4.25968978124929));
#14354=CARTESIAN_POINT('Ctrl Pts',(-16.8096664507721,11.3794667357678,4.14854863372026));
#14355=CARTESIAN_POINT('Ctrl Pts',(-14.8224283335829,12.2685434625389,4.03740748619125));
#14356=CARTESIAN_POINT('Ctrl Pts',(-12.9977322993921,11.0810851924073,3.92626633866222));
#14357=CARTESIAN_POINT('Ctrl Pts',(-13.0058329570596,8.90404427872736,3.81512519113321));
#14358=CARTESIAN_POINT('Ctrl Pts',(-14.839315284823,7.73019790279997,3.70398404360418));
#14359=CARTESIAN_POINT('Ctrl Pts',(-16.8198820480584,8.63403862818544,3.59284289607517));
#14360=CARTESIAN_POINT('Ctrl Pts',(-17.1346007350153,10.7882263889324,3.48170174854614));
#14361=CARTESIAN_POINT('Ctrl Pts',(-15.4953903023094,12.220902876433,3.37056060101713));
#14362=CARTESIAN_POINT('Ctrl Pts',(-13.4027191725303,11.6206526760196,3.2594194534881));
#14363=CARTESIAN_POINT('Ctrl Pts',(-12.7721357624171,9.53692108984355,3.14827830595909));
#14364=CARTESIAN_POINT('Ctrl Pts',(-14.1808511949796,7.87707362973266,3.03713715843006));
#14365=CARTESIAN_POINT('Ctrl Pts',(-16.339383057921,8.16046903752571,2.92599601090105));
#14366=CARTESIAN_POINT('Ctrl Pts',(-17.2718966232842,10.1276983606744,2.81485486337203));
#14367=CARTESIAN_POINT('Ctrl Pts',(-16.1248058408786,11.9780376537872,2.70371371584301));
#14368=CARTESIAN_POINT('Ctrl Pts',(-13.9481122620199,12.0177594806538,2.59257256831399));
#14369=CARTESIAN_POINT('Ctrl Pts',(-12.7342751309326,10.2105040551935,2.48143142078497));
#14370=CARTESIAN_POINT('Ctrl Pts',(-13.5943929683785,8.21056153520229,2.37029027325595));
#14371=CARTESIAN_POINT('Ctrl Pts',(-15.7411479094776,7.84860024839477,2.25914912572693));
#14372=CARTESIAN_POINT('Ctrl Pts',(-17.2094853586029,9.45594521863734,2.14800797819791));
#14373=CARTESIAN_POINT('Ctrl Pts',(-16.6553472594571,11.5612964614294,2.03686683066889));
#14374=CARTESIAN_POINT('Ctrl Pts',(-14.5859697338077,12.2374985820703,1.92572568313987));
#14375=CARTESIAN_POINT('Ctrl Pts',(-12.895579126773,10.8655830947167,1.81458453561085));
#14376=CARTESIAN_POINT('Ctrl Pts',(-13.1314922220546,8.70134680680606,1.70344338808183));
#14377=CARTESIAN_POINT('Ctrl Pts',(-15.0777633965643,7.72584680703849,1.59230224055281));
#14378=CARTESIAN_POINT('Ctrl Pts',(-16.9528531635576,8.83201576375435,1.48116109302379));
#14379=CARTESIAN_POINT('Ctrl Pts',(-17.0403780978937,11.0073131848898,1.37001994549477));
#14380=CARTESIAN_POINT('Ctrl Pts',(-15.260222082372,12.260552314188,1.25887879796575));
#14381=CARTESIAN_POINT('Ctrl Pts',(-13.2418681054385,11.4445782573353,1.14773765043673));
#14382=CARTESIAN_POINT('Ctrl Pts',(-12.8328404069114,9.30628075369691,1.03659650290771));
#14383=CARTESIAN_POINT('Ctrl Pts',(-14.4075413318195,7.80301282089239,0.925455355378688));
#14384=CARTESIAN_POINT('Ctrl Pts',(-16.5245624508558,8.31072893194794,0.814314207849671));
#14385=CARTESIAN_POINT('Ctrl Pts',(-17.2460459036167,10.3648361367336,0.703173060320649));
#14386=CARTESIAN_POINT('Ctrl Pts',(-15.9116138458206,12.0847946289742,0.592031912791631));
#14387=CARTESIAN_POINT('Ctrl Pts',(-13.7426759187313,11.8967869117706,0.480890765262609));
#14388=CARTESIAN_POINT('Ctrl Pts',(-12.7247407619296,9.97181359191189,0.369749617733589));
#14389=CARTESIAN_POINT('Ctrl Pts',(-13.789298366635,8.07404218383939,0.25860847020457));
#14390=CARTESIAN_POINT('Ctrl Pts',(-15.9624482653224,7.93647831452539,0.147467322675549));
#14391=CARTESIAN_POINT('Ctrl Pts',(-17.2539408231974,9.69331193100106,0.03632617514653));
#14392=CARTESIAN_POINT('Ctrl Pts',(-16.7401419234678,11.0430754462783,-0.0377679232061492));
#14393=CARTESIAN_POINT('Ctrl Pts',(-16.2545572343013,11.4602577992624,-0.0748149723824891));
#14394=CARTESIAN_POINT('Ctrl Pts',(-13.4347998857283,11.3312198033322,8.22444491714747));
#14395=CARTESIAN_POINT('Ctrl Pts',(-12.9921246576009,10.8107382751008,8.18739786797113));
#14396=CARTESIAN_POINT('Ctrl Pts',(-12.6745777742391,9.30234073099377,8.11330376961845));
#14397=CARTESIAN_POINT('Ctrl Pts',(-14.3279719097048,7.66457171702036,8.00216262208942));
#14398=CARTESIAN_POINT('Ctrl Pts',(-16.596302048884,8.17050445800021,7.89102147456042));
#14399=CARTESIAN_POINT('Ctrl Pts',(-17.4035114757606,10.3481378462139,7.77988032703138));
#14400=CARTESIAN_POINT('Ctrl Pts',(-16.0106087131083,12.2086083874229,7.66873917950237));
#14401=CARTESIAN_POINT('Ctrl Pts',(-13.6926512300581,12.0466287931598,7.55759803197335));
#14402=CARTESIAN_POINT('Ctrl Pts',(-12.5713806281451,10.011647112944,7.44645688444433));
#14403=CARTESIAN_POINT('Ctrl Pts',(-13.673176561786,7.96579721763555,7.33531573691531));
#14404=CARTESIAN_POINT('Ctrl Pts',(-15.989491953976,7.78208289239259,7.22417458938629));
#14405=CARTESIAN_POINT('Ctrl Pts',(-17.4000666978926,9.62850710689255,7.11303344185727));
#14406=CARTESIAN_POINT('Ctrl Pts',(-16.613714673456,11.81500965758,7.00189229432825));
#14407=CARTESIAN_POINT('Ctrl Pts',(-14.3502323469365,12.3401094557021,6.89075114679924));
#14408=CARTESIAN_POINT('Ctrl Pts',(-12.6815214807272,10.7231731461125,6.77960999927021));
#14409=CARTESIAN_POINT('Ctrl Pts',(-13.1350542708035,8.44426882360712,6.66846885174119));
#14410=CARTESIAN_POINT('Ctrl Pts',(-15.2956846065833,7.58942132854296,6.55732770421217));
#14411=CARTESIAN_POINT('Ctrl Pts',(-17.1856569656411,8.94112120502986,6.44618655668315));
#14412=CARTESIAN_POINT('Ctrl Pts',(-17.0749653387131,11.262077403518,6.33504540915413));
#14413=CARTESIAN_POINT('Ctrl Pts',(-15.0649324820269,12.4277775671245,6.22390426162511));
#14414=CARTESIAN_POINT('Ctrl Pts',(-12.9954629954269,11.3711862728547,6.11276311409609));
#14415=CARTESIAN_POINT('Ctrl Pts',(-12.7608674333771,9.05946520162959,6.00162196656707));
#14416=CARTESIAN_POINT('Ctrl Pts',(-14.5758852960858,7.60867253808055,5.89048081903805));
#14417=CARTESIAN_POINT('Ctrl Pts',(-16.7791209914542,8.34680647046468,5.77933967150903));
#14418=CARTESIAN_POINT('Ctrl Pts',(-17.3538196700229,10.5982084095707,5.66819852398001));
#14419=CARTESIAN_POINT('Ctrl Pts',(-15.7739248829336,12.3020340159819,5.557057376451));
#14420=CARTESIAN_POINT('Ctrl Pts',(-13.485609855698,11.8986686996438,5.44591622892196));
#14421=CARTESIAN_POINT('Ctrl Pts',(-12.5835076939429,9.75733711966703,5.33477508139296));
#14422=CARTESIAN_POINT('Ctrl Pts',(-13.8933670511534,7.83812954719161,5.22363393386392));
#14423=CARTESIAN_POINT('Ctrl Pts',(-16.2161944581144,7.89781271554394,5.11249278633492));
#14424=CARTESIAN_POINT('Ctrl Pts',(-17.4257655413481,9.88175501259879,5.00135163880589));
#14425=CARTESIAN_POINT('Ctrl Pts',(-16.4148867526426,11.9739340961105,4.89021049127687));
#14426=CARTESIAN_POINT('Ctrl Pts',(-14.1088765692626,12.2592519491796,4.77906934374786));
#14427=CARTESIAN_POINT('Ctrl Pts',(-12.6185655430924,10.4765398893022,4.66792819621883));
#14428=CARTESIAN_POINT('Ctrl Pts',(-13.3081254668317,8.25762205516231,4.55678704868981));
#14429=CARTESIAN_POINT('Ctrl Pts',(-15.5463604486011,7.63360810539413,4.44564590116079));
#14430=CARTESIAN_POINT('Ctrl Pts',(-17.2844786765246,9.17569573872837,4.33450475363177));
#14431=CARTESIAN_POINT('Ctrl Pts',(-16.9314754426754,11.4723189032909,4.22336360610276));
#14432=CARTESIAN_POINT('Ctrl Pts',(-14.8104759510498,12.4212395531045,4.11222245857373));
#14433=CARTESIAN_POINT('Ctrl Pts',(-12.8629592808463,11.1538532416754,4.00108131104471));
#14434=CARTESIAN_POINT('Ctrl Pts',(-12.8716051953172,8.83027529134189,3.8899401635157));
#14435=CARTESIAN_POINT('Ctrl Pts',(-14.8284995661796,7.57741709329663,3.77879901598667));
#14436=CARTESIAN_POINT('Ctrl Pts',(-16.9423786537519,8.54209550927056,3.66765786845766));
#14437=CARTESIAN_POINT('Ctrl Pts',(-17.2782811151966,10.8412820566144,3.55651672092863));
#14438=CARTESIAN_POINT('Ctrl Pts',(-15.5287351174808,12.3703922701155,3.44537557339962));
#14439=CARTESIAN_POINT('Ctrl Pts',(-13.2952058971985,11.7297391149084,3.33423442587059));
#14440=CARTESIAN_POINT('Ctrl Pts',(-12.6221777981957,9.50575116060393,3.22309327834158));
#14441=CARTESIAN_POINT('Ctrl Pts',(-14.125714133608,7.73417905325592,3.11195213081255));
#14442=CARTESIAN_POINT('Ctrl Pts',(-16.4295371854886,8.03664985967757,3.00081098328354));
#14443=CARTESIAN_POINT('Ctrl Pts',(-17.4248184157354,10.1362937615422,2.88966983575451));
#14444=CARTESIAN_POINT('Ctrl Pts',(-16.2005167352846,12.1111797432876,2.7785286882255));
#14445=CARTESIAN_POINT('Ctrl Pts',(-13.8773094989449,12.1535752538516,2.66738754069648));
#14446=CARTESIAN_POINT('Ctrl Pts',(-12.5817687604279,10.2246731230589,2.55624639316746));
#14447=CARTESIAN_POINT('Ctrl Pts',(-13.4997812925854,8.09011409287,2.44510524563844));
#14448=CARTESIAN_POINT('Ctrl Pts',(-15.7910347157817,7.70378912322181,2.33396409810942));
#14449=CARTESIAN_POINT('Ctrl Pts',(-17.3582062369956,9.4193247881543,2.2228229505804));
#14450=CARTESIAN_POINT('Ctrl Pts',(-16.766768997335,11.6663876222607,2.11168180305137));
#14451=CARTESIAN_POINT('Ctrl Pts',(-14.5581012780927,12.3881050358458,2.00054065552236));
#14452=CARTESIAN_POINT('Ctrl Pts',(-12.7539301588106,10.9238456569314,1.88939950799334));
#14453=CARTESIAN_POINT('Ctrl Pts',(-13.0057226092633,8.61393421415536,1.77825836046432));
#14454=CARTESIAN_POINT('Ctrl Pts',(-15.0829976655305,7.57277312445451,1.6671172129353));
#14455=CARTESIAN_POINT('Ctrl Pts',(-17.0843000802458,8.75339852336988,1.55597606540628));
#14456=CARTESIAN_POINT('Ctrl Pts',(-17.1777163345064,11.0751156263452,1.44483491787726));
#14457=CARTESIAN_POINT('Ctrl Pts',(-15.277737680073,12.4127105190431,1.33369377034824));
#14458=CARTESIAN_POINT('Ctrl Pts',(-13.1235279142844,11.5418130937198,1.22255262281922));
#14459=CARTESIAN_POINT('Ctrl Pts',(-12.6869684838201,9.25958637970326,1.1114114752902));
#14460=CARTESIAN_POINT('Ctrl Pts',(-14.3676628265377,7.65513319733112,1.00027032776118));
#14461=CARTESIAN_POINT('Ctrl Pts',(-16.6271810384708,8.19702377608174,0.88912918023216));
#14462=CARTESIAN_POINT('Ctrl Pts',(-17.3972276792259,10.3893933262678,0.777988032703138));
#14463=CARTESIAN_POINT('Ctrl Pts',(-15.9729747466193,12.225122550715,0.66684688517412));
#14464=CARTESIAN_POINT('Ctrl Pts',(-13.6580451964401,12.0244599984212,0.555705737645099));
#14465=CARTESIAN_POINT('Ctrl Pts',(-12.5715926312396,9.9699163594395,0.444564590116078));
#14466=CARTESIAN_POINT('Ctrl Pts',(-13.7078058101514,7.94440559808363,0.333423442587059));
#14467=CARTESIAN_POINT('Ctrl Pts',(-16.0272308405357,7.79758227864481,0.222282295058039));
#14468=CARTESIAN_POINT('Ctrl Pts',(-17.4056540073404,9.67266869893052,0.111141147529019));
#14469=CARTESIAN_POINT('Ctrl Pts',(-16.8572712062568,11.1132850523281,0.0370470491763399));
#14470=CARTESIAN_POINT('Ctrl Pts',(-16.3390017195986,11.5585480285869,0.));
#14471=CARTESIAN_POINT('Ctrl Pts',(-13.7309291201476,11.0793586530485,8.));
#14472=CARTESIAN_POINT('Ctrl Pts',(-13.6852152716991,11.0367124842021,8.));
#14473=CARTESIAN_POINT('Ctrl Pts',(-13.6422346164434,10.9914156431349,8.));
#14474=CARTESIAN_POINT('Ctrl Pts',(-13.601998738308,10.9438052169207,8.));
#14475=CARTESIAN_POINT('Ctrl Pts',(-13.5764667336105,10.9135936325813,8.));
#14476=CARTESIAN_POINT('Ctrl Pts',(-13.5520403842569,10.8824494351603,8.));
#14477=CARTESIAN_POINT('Ctrl Pts',(-13.5287280007931,10.850449719119,8.));
#14478=CARTESIAN_POINT('Ctrl Pts',(-13.5126489582125,10.8283788400261,8.));
#14479=CARTESIAN_POINT('Ctrl Pts',(-13.497099934263,10.8059008351366,8.));
#14480=CARTESIAN_POINT('Ctrl Pts',(-13.4820849794618,10.7830393699546,8.));
#14481=CARTESIAN_POINT('Ctrl Pts',(-13.4742666591409,10.7711353542471,8.));
#14482=CARTESIAN_POINT('Ctrl Pts',(-13.4665935957101,10.7591278087324,8.));
#14483=CARTESIAN_POINT('Ctrl Pts',(-13.4590733535016,10.7470317213655,8.));
#14484=CARTESIAN_POINT('Ctrl Pts',(-13.4242375073996,10.6909992923205,8.));
#14485=CARTESIAN_POINT('Ctrl Pts',(-13.3926366847534,10.6330080071976,8.));
#14486=CARTESIAN_POINT('Ctrl Pts',(-13.3643038144212,10.5734090455691,8.));
#14487=CARTESIAN_POINT('Ctrl Pts',(-13.3438796821625,10.5304463291022,8.));
#14488=CARTESIAN_POINT('Ctrl Pts',(-13.3251543285811,10.4866471329582,8.));
#14489=CARTESIAN_POINT('Ctrl Pts',(-13.3081517237824,10.4421310384001,8.));
#14490=CARTESIAN_POINT('Ctrl Pts',(-13.3034050847435,10.4297034230557,8.));
#14491=CARTESIAN_POINT('Ctrl Pts',(-13.2987927744426,10.4172198853085,8.));
#14492=CARTESIAN_POINT('Ctrl Pts',(-13.2943154661998,10.4046829194981,8.));
#14493=CARTESIAN_POINT('Ctrl Pts',(-13.2899383781238,10.3924265814078,8.));
#14494=CARTESIAN_POINT('Ctrl Pts',(-13.2856933225078,10.3801275302436,8.));
#14495=CARTESIAN_POINT('Ctrl Pts',(-13.2815814261066,10.367791367639,8.));
#14496=CARTESIAN_POINT('Ctrl Pts',(-13.2601244711192,10.303418032346,8.));
#14497=CARTESIAN_POINT('Ctrl Pts',(-13.2422813001474,10.2380113738685,8.));
#14498=CARTESIAN_POINT('Ctrl Pts',(-13.2280844604704,10.1719275884727,8.));
#14499=CARTESIAN_POINT('Ctrl Pts',(-13.213683957365,10.1048957857298,8.));
#14500=CARTESIAN_POINT('Ctrl Pts',(-13.2030346042218,10.0371663785979,8.));
#14501=CARTESIAN_POINT('Ctrl Pts',(-13.1962126701045,9.96907944108561,8.));
#14502=CARTESIAN_POINT('Ctrl Pts',(-13.1919872272218,9.92690702186065,8.));
#14503=CARTESIAN_POINT('Ctrl Pts',(-13.1892310184523,9.88459686452187,8.));
#14504=CARTESIAN_POINT('Ctrl Pts',(-13.1879715509946,9.84222623000023,8.));
#14505=CARTESIAN_POINT('Ctrl Pts',(-13.1869384830453,9.8074720612857,8.));
#14506=CARTESIAN_POINT('Ctrl Pts',(-13.1869125402926,9.77267713446997,8.));
#14507=CARTESIAN_POINT('Ctrl Pts',(-13.1879128834702,9.73788353314392,8.));
#14508=CARTESIAN_POINT('Ctrl Pts',(-13.1883195913401,9.72373755624667,8.));
#14509=CARTESIAN_POINT('Ctrl Pts',(-13.1888962462514,9.70958938159508,8.));
#14510=CARTESIAN_POINT('Ctrl Pts',(-13.1896426561975,9.69546565230446,8.));
#14511=CARTESIAN_POINT('Ctrl Pts',(-13.1933622318364,9.62508304329351,8.));
#14512=CARTESIAN_POINT('Ctrl Pts',(-13.2012954945328,9.55518382486859,8.));
#14513=CARTESIAN_POINT('Ctrl Pts',(-13.2135052750766,9.48612542924265,8.));
#14514=CARTESIAN_POINT('Ctrl Pts',(-13.2148602658297,9.47846161520753,8.));
#14515=CARTESIAN_POINT('Ctrl Pts',(-13.2162679737953,9.4708081370592,8.));
#14516=CARTESIAN_POINT('Ctrl Pts',(-13.2177285223696,9.46316547049678,8.));
#14517=CARTESIAN_POINT('Ctrl Pts',(-13.2303835600112,9.39694498681769,8.));
#14518=CARTESIAN_POINT('Ctrl Pts',(-13.2470012041599,9.33153634460149,8.));
#14519=CARTESIAN_POINT('Ctrl Pts',(-13.2673104055905,9.26714714029771,8.));
#14520=CARTESIAN_POINT('Ctrl Pts',(-13.2891624783375,9.19786634748179,8.));
#14521=CARTESIAN_POINT('Ctrl Pts',(-13.315288085799,9.12976478423422,8.));
#14522=CARTESIAN_POINT('Ctrl Pts',(-13.3454136056875,9.06310682836119,8.));
#14523=CARTESIAN_POINT('Ctrl Pts',(-13.3509659872551,9.05082121779261,8.));
#14524=CARTESIAN_POINT('Ctrl Pts',(-13.35665441154,9.03858468597769,8.));
#14525=CARTESIAN_POINT('Ctrl Pts',(-13.3624773867768,9.02639895256681,8.));
#14526=CARTESIAN_POINT('Ctrl Pts',(-13.3674119000146,9.01607250253326,8.));
#14527=CARTESIAN_POINT('Ctrl Pts',(-13.3724389146256,9.00579117530112,8.));
#14528=CARTESIAN_POINT('Ctrl Pts',(-13.3775566194876,8.99555672351709,8.));
#14529=CARTESIAN_POINT('Ctrl Pts',(-13.4093425266683,8.93199085889207,8.));
#14530=CARTESIAN_POINT('Ctrl Pts',(-13.444627394604,8.87022282259155,8.));
#14531=CARTESIAN_POINT('Ctrl Pts',(-13.4831031309424,8.81047698893777,8.));
#14532=CARTESIAN_POINT('Ctrl Pts',(-13.5223915933793,8.74946913919547,8.));
#14533=CARTESIAN_POINT('Ctrl Pts',(-13.5650075075404,8.69056895823217,8.));
#14534=CARTESIAN_POINT('Ctrl Pts',(-13.6106773499442,8.63402362180269,8.));
#14535=CARTESIAN_POINT('Ctrl Pts',(-13.6566251153189,8.57713417978688,8.));
#14536=CARTESIAN_POINT('Ctrl Pts',(-13.7056646272697,8.52262739947179,8.));
#14537=CARTESIAN_POINT('Ctrl Pts',(-13.7575649500188,8.47077690562292,8.));
#14538=CARTESIAN_POINT('Ctrl Pts',(-13.7703956403815,8.4579585338578,8.));
#14539=CARTESIAN_POINT('Ctrl Pts',(-13.7834013784189,8.44530264814056,8.));
#14540=CARTESIAN_POINT('Ctrl Pts',(-13.7965790599829,8.43281369133694,8.));
#14541=CARTESIAN_POINT('Ctrl Pts',(-13.8068736174222,8.42305717365612,8.));
#14542=CARTESIAN_POINT('Ctrl Pts',(-13.8172743724373,8.41340154458166,8.));
#14543=CARTESIAN_POINT('Ctrl Pts',(-13.8277637530731,8.40386320384444,8.));
#14544=CARTESIAN_POINT('Ctrl Pts',(-13.8835124617526,8.35316905921277,8.));
#14545=CARTESIAN_POINT('Ctrl Pts',(-13.9418585842011,8.3056917081039,8.));
#14546=CARTESIAN_POINT('Ctrl Pts',(-14.0025043610684,8.26168470116104,8.));
#14547=CARTESIAN_POINT('Ctrl Pts',(-14.0632169295863,8.21762922751878,8.));
#14548=CARTESIAN_POINT('Ctrl Pts',(-14.1262348596866,8.1770508152945,8.));
#14549=CARTESIAN_POINT('Ctrl Pts',(-14.1913041268544,8.14023030306485,8.));
#14550=CARTESIAN_POINT('Ctrl Pts',(-14.2548907910063,8.10424874607246,8.));
#14551=CARTESIAN_POINT('Ctrl Pts',(-14.3204371099339,8.07185505382328,8.));
#14552=CARTESIAN_POINT('Ctrl Pts',(-14.3877383485173,8.04334865248953,8.));
#14553=CARTESIAN_POINT('Ctrl Pts',(-14.4022444047088,8.03720440509873,8.));
#14554=CARTESIAN_POINT('Ctrl Pts',(-14.4168320883943,8.03124091428558,8.));
#14555=CARTESIAN_POINT('Ctrl Pts',(-14.431499502301,8.02546146405585,8.));
#14556=CARTESIAN_POINT('Ctrl Pts',(-14.4438537777607,8.02059346751615,8.));
#14557=CARTESIAN_POINT('Ctrl Pts',(-14.4562646196476,8.01585604250524,8.));
#14558=CARTESIAN_POINT('Ctrl Pts',(-14.4687302296836,8.0112487681312,8.));
#14559=CARTESIAN_POINT('Ctrl Pts',(-16.6673099161007,9.99870037981829,6.87148036339021));
#14560=CARTESIAN_POINT('Ctrl Pts',(-16.6680395399047,9.91361837787032,6.87718308383007));
#14561=CARTESIAN_POINT('Ctrl Pts',(-16.6620893791087,9.82863879732174,6.88288580426994));
#14562=CARTESIAN_POINT('Ctrl Pts',(-16.6491046531255,9.7447481484841,6.8885885247098));
#14563=CARTESIAN_POINT('Ctrl Pts',(-16.5647509157971,9.19976246565146,6.92563557388614));
#14564=CARTESIAN_POINT('Ctrl Pts',(-16.1835175908403,8.70073294196944,6.96268262306248));
#14565=CARTESIAN_POINT('Ctrl Pts',(-15.6798878737819,8.47604423892347,6.99972967223882));
#14566=CARTESIAN_POINT('Ctrl Pts',(-15.1762581567236,8.25135553587751,7.03677672141516));
#14567=CARTESIAN_POINT('Ctrl Pts',(-14.5502320475638,8.30100765346761,7.0738237705915));
#14568=CARTESIAN_POINT('Ctrl Pts',(-14.0883288583003,8.6022976718347,7.11087081976784));
#14569=CARTESIAN_POINT('Ctrl Pts',(-13.6264256690369,8.90358769020179,7.14791786894418));
#14570=CARTESIAN_POINT('Ctrl Pts',(-13.3286453996698,9.45651560934587,7.18496491812052));
#14571=CARTESIAN_POINT('Ctrl Pts',(-13.3312770902519,10.0079748626876,7.22201196729686));
#14572=CARTESIAN_POINT('Ctrl Pts',(-13.333908780834,10.5594341160293,7.2590590164732));
#14573=CARTESIAN_POINT('Ctrl Pts',(-13.6369524313653,11.1094247035687,7.29610606564955));
#14574=CARTESIAN_POINT('Ctrl Pts',(-14.1017092135812,11.4063089541492,7.33315311482589));
#14575=CARTESIAN_POINT('Ctrl Pts',(-14.5664659957971,11.7031932047297,7.37020016400223));
#14576=CARTESIAN_POINT('Ctrl Pts',(-15.1929359096976,11.7469711183514,7.40724721317856));
#14577=CARTESIAN_POINT('Ctrl Pts',(-15.6943994429207,11.5174471764597,7.4442942623549));
#14578=CARTESIAN_POINT('Ctrl Pts',(-16.1958629761437,11.287923234568,7.48134131153124));
#14579=CARTESIAN_POINT('Ctrl Pts',(-16.5723201286892,10.7850974371629,7.51838836070758));
#14580=CARTESIAN_POINT('Ctrl Pts',(-16.6514672347769,10.2394121432165,7.55543540988392));
#14581=CARTESIAN_POINT('Ctrl Pts',(-16.6628933507166,10.1606339826064,7.56078372771935));
#14582=CARTESIAN_POINT('Ctrl Pts',(-16.6681231050028,10.080962569501,7.56613204555478));
#14583=CARTESIAN_POINT('Ctrl Pts',(-16.6674569633666,10.0012065537184,7.57148036339021));
#14584=CARTESIAN_POINT('Ctrl Pts',(-15.5301702171886,8.01482567432828,8.));
#14585=CARTESIAN_POINT('Ctrl Pts',(-16.1903072548812,8.1911250512252,7.96295295082366));
#14586=CARTESIAN_POINT('Ctrl Pts',(-17.3094430093426,9.25114168831851,7.88885885247098));
#14587=CARTESIAN_POINT('Ctrl Pts',(-16.8810963203827,11.5386107605189,7.77771770494196));
#14588=CARTESIAN_POINT('Ctrl Pts',(-14.7276622354211,12.4126888235087,7.66657655741294));
#14589=CARTESIAN_POINT('Ctrl Pts',(-12.8251333276493,11.0807508020576,7.55543540988392));
#14590=CARTESIAN_POINT('Ctrl Pts',(-12.9125602025977,8.75827697936691,7.4442942623549));
#14591=CARTESIAN_POINT('Ctrl Pts',(-14.9111754557965,7.5730758609676,7.33315311482589));
#14592=CARTESIAN_POINT('Ctrl Pts',(-16.9908761101702,8.6090506269142,7.22201196729686));
#14593=CARTESIAN_POINT('Ctrl Pts',(-17.2483215538839,10.9184180559112,7.11087081976785));
#14594=CARTESIAN_POINT('Ctrl Pts',(-15.447683477411,12.3870128478829,6.99972967223881));
#14595=CARTESIAN_POINT('Ctrl Pts',(-13.2372840161297,11.670676405265,6.88858852470981));
#14596=CARTESIAN_POINT('Ctrl Pts',(-12.6403894048645,9.42504512087116,6.77744737718078));
#14597=CARTESIAN_POINT('Ctrl Pts',(-14.2033971295295,7.70571703676082,6.66630622965177));
#14598=CARTESIAN_POINT('Ctrl Pts',(-16.4955794550137,8.08647855754376,6.55516508212274));
#14599=CARTESIAN_POINT('Ctrl Pts',(-17.4187696292973,10.218805211767,6.44402393459373));
#14600=CARTESIAN_POINT('Ctrl Pts',(-16.1279126020198,12.1508445448559,6.33288278706471));
#14601=CARTESIAN_POINT('Ctrl Pts',(-13.8046095450231,12.114086684316,6.22174163953567));
#14602=CARTESIAN_POINT('Ctrl Pts',(-12.5755193539972,10.1421770075384,6.11060049200667));
#14603=CARTESIAN_POINT('Ctrl Pts',(-13.5657030451356,8.04012435007543,5.99945934447765));
#14604=CARTESIAN_POINT('Ctrl Pts',(-15.8687853839106,7.73206425811983,5.88831819694862));
#14605=CARTESIAN_POINT('Ctrl Pts',(-17.3766159710247,9.4999829410875,5.7771770494196));
#14606=CARTESIAN_POINT('Ctrl Pts',(-16.7089862387355,11.7255974394772,5.66603590189059));
#14607=CARTESIAN_POINT('Ctrl Pts',(-14.4770180804847,12.3716682810349,5.55489475436156));
#14608=CARTESIAN_POINT('Ctrl Pts',(-12.7237668892609,10.8468077355158,5.44375360683255));
#14609=CARTESIAN_POINT('Ctrl Pts',(-13.0540894977656,8.54681287249504,5.33261245930352));
#14610=CARTESIAN_POINT('Ctrl Pts',(-15.1656216453787,7.57700805081118,5.22147131177451));
#14611=CARTESIAN_POINT('Ctrl Pts',(-17.1255502875653,8.82511426562272,5.11033016424548));
#14612=CARTESIAN_POINT('Ctrl Pts',(-17.139834231474,11.1486644310237,4.99918901671647));
#14613=CARTESIAN_POINT('Ctrl Pts',(-15.195398520178,12.4207725899548,4.88804786918745));
#14614=CARTESIAN_POINT('Ctrl Pts',(-13.0721027286448,11.4770012270902,4.77690672165843));
#14615=CARTESIAN_POINT('Ctrl Pts',(-12.7135278783817,9.18124133547139,4.66576557412941));
#14616=CARTESIAN_POINT('Ctrl Pts',(-14.4478992106895,7.63494075503149,4.55462442660039));
#14617=CARTESIAN_POINT('Ctrl Pts',(-16.687641777794,8.25352190292165,4.44348327907136));
#14618=CARTESIAN_POINT('Ctrl Pts',(-17.3825837837853,10.4707600524374,4.33234213154235));
#14619=CARTESIAN_POINT('Ctrl Pts',(-15.8966027914863,12.2570830618385,4.22120098401332));
#14620=CARTESIAN_POINT('Ctrl Pts',(-13.5899070517775,11.9773614720396,4.11005983648431));
#14621=CARTESIAN_POINT('Ctrl Pts',(-12.5739546477039,9.8876413673274,3.99891868895528));
#14622=CARTESIAN_POINT('Ctrl Pts',(-13.7787082434502,7.90076991277298,3.88777754142627));
#14623=CARTESIAN_POINT('Ctrl Pts',(-16.1013840283822,7.83545068530234,3.77663639389724));
#14624=CARTESIAN_POINT('Ctrl Pts',(-17.4158964178437,9.75147432329159,3.66549524636823));
#14625=CARTESIAN_POINT('Ctrl Pts',(-16.518992740837,11.8949885400772,3.5543540988392));
#14626=CARTESIAN_POINT('Ctrl Pts',(-14.2316631634768,12.3039051671823,3.44321295131019));
#14627=CARTESIAN_POINT('Ctrl Pts',(-12.647638749453,10.6039180910149,3.33207180378117));
#14628=CARTESIAN_POINT('Ctrl Pts',(-13.2168728216632,8.35112827071217,3.22093065625215));
#14629=CARTESIAN_POINT('Ctrl Pts',(-15.4183110155551,7.60765044194128,3.10978950872313));
#14630=CARTESIAN_POINT('Ctrl Pts',(-17.2368438440502,9.05403481509122,2.99864836119411));
#14631=CARTESIAN_POINT('Ctrl Pts',(-17.0078582531826,11.3663183190935,2.88750721366509));
#14632=CARTESIAN_POINT('Ctrl Pts',(-14.9409585995702,12.4279280521305,2.77636606613606));
#14633=CARTESIAN_POINT('Ctrl Pts',(-12.9281031098292,11.2671084366828,2.66522491860705));
#14634=CARTESIAN_POINT('Ctrl Pts',(-12.8117801189011,8.94642785381579,2.55408377107803));
#14635=CARTESIAN_POINT('Ctrl Pts',(-14.6984670947123,7.59014556097653,2.44294262354901));
#14636=CARTESIAN_POINT('Ctrl Pts',(-16.8611653694553,8.43974874366516,2.33180147601999));
#14637=CARTESIAN_POINT('Ctrl Pts',(-17.3202264500472,10.7175442452619,2.22066032849097));
#14638=CARTESIAN_POINT('Ctrl Pts',(-15.655443965717,12.3385281044116,2.10951918096195));
#14639=CARTESIAN_POINT('Ctrl Pts',(-13.3906939975623,11.8189158098855,1.99837803343293));
#14640=CARTESIAN_POINT('Ctrl Pts',(-12.5990391016035,9.63433986139397,1.88723688590391));
#14641=CARTESIAN_POINT('Ctrl Pts',(-14.0051289214666,7.7844748128269,1.77609573837489));
#14642=CARTESIAN_POINT('Ctrl Pts',(-16.3218843289188,7.96261380065688,1.66495459084587));
#14643=CARTESIAN_POINT('Ctrl Pts',(-17.4286392087695,10.0056958124645,1.55381344331685));
#14644=CARTESIAN_POINT('Ctrl Pts',(-16.3123135322607,12.0435636244015,1.44267229578783));
#14645=CARTESIAN_POINT('Ctrl Pts',(-13.9947484023904,12.2108350155113,1.33153114825881));
#14646=CARTESIAN_POINT('Ctrl Pts',(-12.5973499293358,10.3543936440402,1.22039000072979));
#14647=CARTESIAN_POINT('Ctrl Pts',(-13.3992441080921,8.17355782375309,1.10924885320077));
#14648=CARTESIAN_POINT('Ctrl Pts',(-15.6664035170272,7.66456821418318,0.998107705671752));
#14649=CARTESIAN_POINT('Ctrl Pts',(-17.323570133058,9.29335360493268,0.886966558142732));
#14650=CARTESIAN_POINT('Ctrl Pts',(-16.8538196455965,11.5689498250439,0.775825410613712));
#14651=CARTESIAN_POINT('Ctrl Pts',(-14.6871808849242,12.408440519574,0.664684263084692));
#14652=CARTESIAN_POINT('Ctrl Pts',(-12.8068360443054,11.0432447977232,0.553543115555672));
#14653=CARTESIAN_POINT('Ctrl Pts',(-12.9341204463425,8.72328850320409,0.442401968026654));
#14654=CARTESIAN_POINT('Ctrl Pts',(-14.9522477729176,7.57162591585277,0.331260820497632));
#14655=CARTESIAN_POINT('Ctrl Pts',(-17.0144376022166,8.64349401570581,0.220119672968612));
#14656=CARTESIAN_POINT('Ctrl Pts',(-17.2320070103418,10.9557091204361,0.108978525439593));
#14657=CARTESIAN_POINT('Ctrl Pts',(-15.4078276845629,12.3957301639888,-0.00216262208942797));
#14658=CARTESIAN_POINT('Ctrl Pts',(-13.2075704878879,11.6375323595232,-0.113303769618446));
#14659=CARTESIAN_POINT('Ctrl Pts',(-12.839200671623,10.1407345153594,-0.187397867971127));
#14660=CARTESIAN_POINT('Ctrl Pts',(-13.0122087991468,9.47972727890995,-0.224444917147467));
#14661=CARTESIAN_POINT('Ctrl Pts',(-15.4967348970877,8.14002119999723,8.07481497238249));
#14662=CARTESIAN_POINT('Ctrl Pts',(-16.1152402239634,8.30520221168044,8.03776792320615));
#14663=CARTESIAN_POINT('Ctrl Pts',(-17.1637973963513,9.29836862893029,7.96367382485347));
#14664=CARTESIAN_POINT('Ctrl Pts',(-16.7624645006887,11.4415778800953,7.85253267732445));
#14665=CARTESIAN_POINT('Ctrl Pts',(-14.7448372860729,12.260531986888,7.74139152979543));
#14666=CARTESIAN_POINT('Ctrl Pts',(-12.9622918495906,11.0125929768072,7.63025038226641));
#14667=CARTESIAN_POINT('Ctrl Pts',(-13.04420512635,8.83658655867844,7.5191092347374));
#14668=CARTESIAN_POINT('Ctrl Pts',(-14.9167771983538,7.72613045139609,7.40796808720836));
#14669=CARTESIAN_POINT('Ctrl Pts',(-16.8653210000062,8.69677120424107,7.29682693967935));
#14670=CARTESIAN_POINT('Ctrl Pts',(-17.1065305810855,10.8604977867405,7.18568579215034));
#14671=CARTESIAN_POINT('Ctrl Pts',(-15.4194502046132,12.2364752732202,7.07454464462131));
#14672=CARTESIAN_POINT('Ctrl Pts',(-13.3484501496788,11.5653147712387,6.96340349709229));
#14673=CARTESIAN_POINT('Ctrl Pts',(-12.7891988494618,9.461304797111,6.85226234956327));
#14674=CARTESIAN_POINT('Ctrl Pts',(-14.2536350929307,7.85040657757425,6.74112120203425));
#14675=CARTESIAN_POINT('Ctrl Pts',(-16.4012603548577,8.20715527583956,6.62998005450523));
#14676=CARTESIAN_POINT('Ctrl Pts',(-17.2662293051071,10.2050062052253,6.51883890697622));
#14677=CARTESIAN_POINT('Ctrl Pts',(-16.0567805058142,12.0152009845181,6.40769775944719));
#14678=CARTESIAN_POINT('Ctrl Pts',(-13.8799971492527,11.9807612678375,6.29655661191817));
#14679=CARTESIAN_POINT('Ctrl Pts',(-12.7284198449139,10.1332105782598,6.18541546438915));
#14680=CARTESIAN_POINT('Ctrl Pts',(-13.6561573487741,8.16372440829958,6.07427431686013));
#14681=CARTESIAN_POINT('Ctrl Pts',(-15.813995211871,7.87509220469174,5.96313316933111));
#14682=CARTESIAN_POINT('Ctrl Pts',(-17.2267340780554,9.53151664456354,5.8519920218021));
#14683=CARTESIAN_POINT('Ctrl Pts',(-16.6012085852808,11.6167721964068,5.74085087427307));
#14684=CARTESIAN_POINT('Ctrl Pts',(-14.5100000687576,12.222098415398,5.62970972674406));
#14685=CARTESIAN_POINT('Ctrl Pts',(-12.8673181115183,10.7934035894831,5.51856857921503));
#14686=CARTESIAN_POINT('Ctrl Pts',(-13.1768088403853,8.63845848969381,5.40742743168602));
#14687=CARTESIAN_POINT('Ctrl Pts',(-15.1551766740293,7.72981465668329,5.296286284157));
#14688=CARTESIAN_POINT('Ctrl Pts',(-16.9915019160211,8.89920873441279,5.18514513662797));
#14689=CARTESIAN_POINT('Ctrl Pts',(-17.0048850393605,11.076223615424,5.07400398909895));
#14690=CARTESIAN_POINT('Ctrl Pts',(-15.1830756626172,12.2681059485394,4.96286284156994));
#14691=CARTESIAN_POINT('Ctrl Pts',(-13.1936860622603,11.3838537676213,4.85172169404091));
#14692=CARTESIAN_POINT('Ctrl Pts',(-12.8577248264742,9.23287655968122,4.74058054651189));
#14693=CARTESIAN_POINT('Ctrl Pts',(-14.4827175879203,7.78409382012157,4.62943939898288));
#14694=CARTESIAN_POINT('Ctrl Pts',(-16.5812102182179,8.36366398999456,4.51829825145385));
#14695=CARTESIAN_POINT('Ctrl Pts',(-17.2323255291807,10.4410714495441,4.40715710392484));
#14696=CARTESIAN_POINT('Ctrl Pts',(-15.8400583075361,12.1147395423041,4.29601595639581));
#14697=CARTESIAN_POINT('Ctrl Pts',(-13.6788349235578,11.8526586659796,4.1848748088668));
#14698=CARTESIAN_POINT('Ctrl Pts',(-12.7269538172226,9.89472729318237,4.07373366133777));
#14699=CARTESIAN_POINT('Ctrl Pts',(-13.8557293198762,8.03315839416316,3.96259251380876));
#14700=CARTESIAN_POINT('Ctrl Pts',(-16.0319249634459,7.97195854044916,3.85145136627973));
#14701=CARTESIAN_POINT('Ctrl Pts',(-17.2635372934674,9.76714765854248,3.74031021875072));
#14702=CARTESIAN_POINT('Ctrl Pts',(-16.423197075833,11.7754806040014,3.62916907122169));
#14703=CARTESIAN_POINT('Ctrl Pts',(-14.2801185222307,12.1586087996206,3.51802792369268));
#14704=CARTESIAN_POINT('Ctrl Pts',(-12.795991012283,10.5658318424231,3.40688677616365));
#14705=CARTESIAN_POINT('Ctrl Pts',(-13.3293261924023,8.45511478728119,3.29574562863464));
#14706=CARTESIAN_POINT('Ctrl Pts',(-15.3919301245631,7.7585245775937,3.18460448110562));
#14707=CARTESIAN_POINT('Ctrl Pts',(-17.0957767159528,9.113692350985,3.0734633335766));
#14708=CARTESIAN_POINT('Ctrl Pts',(-16.8812321598339,11.2801511054751,2.96232218604758));
#14709=CARTESIAN_POINT('Ctrl Pts',(-14.9446820605617,12.2748101496661,2.85118103851856));
#14710=CARTESIAN_POINT('Ctrl Pts',(-13.0587678161688,11.1871979196271,2.74003989098954));
#14711=CARTESIAN_POINT('Ctrl Pts',(-12.9497807643611,9.01287165019477,2.62889874346052));
#14712=CARTESIAN_POINT('Ctrl Pts',(-14.7174833443665,7.74212364641602,2.5177575959315));
#14713=CARTESIAN_POINT('Ctrl Pts',(-16.74379050027,8.53814638748237,2.40661644840248));
#14714=CARTESIAN_POINT('Ctrl Pts',(-17.1739007766148,10.6722921342434,2.29547530087346));
#14715=CARTESIAN_POINT('Ctrl Pts',(-15.6141082246824,12.1910482324743,2.18433415334444));
#14716=CARTESIAN_POINT('Ctrl Pts',(-13.4921852914663,11.7042054199608,2.07319300581542));
#14717=CARTESIAN_POINT('Ctrl Pts',(-12.7504563136328,9.65740031138922,1.9620518582864));
#14718=CARTESIAN_POINT('Ctrl Pts',(-14.0678707200277,7.92419747438564,1.85091071075738));
#14719=CARTESIAN_POINT('Ctrl Pts',(-16.2385193562348,8.09110208146877,1.73976956322836));
#14720=CARTESIAN_POINT('Ctrl Pts',(-17.2754764570301,10.0053366045973,1.62862841569934));
#14721=CARTESIAN_POINT('Ctrl Pts',(-16.2295521443114,11.9146857627012,1.51748726817032));
#14722=CARTESIAN_POINT('Ctrl Pts',(-14.0581448510371,12.0714081408258,1.4063461206413));
#14723=CARTESIAN_POINT('Ctrl Pts',(-12.7488736694455,10.3320437184011,1.29520497311228));
#14724=CARTESIAN_POINT('Ctrl Pts',(-13.5001961870926,8.28874286589384,1.18406382558326));
#14725=CARTESIAN_POINT('Ctrl Pts',(-15.6243766090913,7.81185281599787,1.07292267805424));
#14726=CARTESIAN_POINT('Ctrl Pts',(-17.1770335894029,9.33791844024638,0.961781530525221));
#14727=CARTESIAN_POINT('Ctrl Pts',(-16.7369080363618,11.4700036037703,0.8506403829962));
#14728=CARTESIAN_POINT('Ctrl Pts',(-14.70690890228,12.2565516033255,0.739499235467183));
#14729=CARTESIAN_POINT('Ctrl Pts',(-12.9451484890921,10.9774522982115,0.628358087938161));
#14730=CARTESIAN_POINT('Ctrl Pts',(-13.0644056678186,8.80380463969748,0.517216940409144));
#14731=CARTESIAN_POINT('Ctrl Pts',(-14.9552592793098,7.72477194744011,0.406075792880121));
#14732=CARTESIAN_POINT('Ctrl Pts',(-16.8873965805413,8.72904241192503,0.294934645351101));
#14733=CARTESIAN_POINT('Ctrl Pts',(-17.0912449183971,10.8954370807606,0.183793497822082));
#14734=CARTESIAN_POINT('Ctrl Pts',(-15.3821079275164,12.2446428295604,0.0726523502930611));
#14735=CARTESIAN_POINT('Ctrl Pts',(-13.3206105126815,11.5342609632034,-0.0384887972359573));
#14736=CARTESIAN_POINT('Ctrl Pts',(-12.9754720329252,10.1318590572183,-0.112582895588638));
#14737=CARTESIAN_POINT('Ctrl Pts',(-13.1375693587171,9.51253841089255,-0.149629944764978));
#14738=CARTESIAN_POINT('Ctrl Pts',(-15.4632995769868,8.26521672566619,8.14962994476498));
#14739=CARTESIAN_POINT('Ctrl Pts',(-16.0401731930456,8.41927937213568,8.11258289558864));
#14740=CARTESIAN_POINT('Ctrl Pts',(-17.0181517833599,9.34559556954207,8.03848879723596));
#14741=CARTESIAN_POINT('Ctrl Pts',(-16.6438326809947,11.3445449996716,7.92734764970694));
#14742=CARTESIAN_POINT('Ctrl Pts',(-14.7620123367246,12.1083751502674,7.81620650217792));
#14743=CARTESIAN_POINT('Ctrl Pts',(-13.0994503715318,10.9444351515568,7.7050653546489));
#14744=CARTESIAN_POINT('Ctrl Pts',(-13.1758500501023,8.91489613798999,7.59392420711989));
#14745=CARTESIAN_POINT('Ctrl Pts',(-14.9223789409112,7.87918504182458,7.48278305959085));
#14746=CARTESIAN_POINT('Ctrl Pts',(-16.7397658898422,8.78449178156794,7.37164191206185));
#14747=CARTESIAN_POINT('Ctrl Pts',(-16.9647396082871,10.8025775175698,7.26050076453282));
#14748=CARTESIAN_POINT('Ctrl Pts',(-15.3912169318155,12.0859376985576,7.1493596170038));
#14749=CARTESIAN_POINT('Ctrl Pts',(-13.4596162832278,11.4599531372124,7.03821846947478));
#14750=CARTESIAN_POINT('Ctrl Pts',(-12.9380082940591,9.49756447335083,6.92707732194576));
#14751=CARTESIAN_POINT('Ctrl Pts',(-14.3038730563318,7.99509611838767,6.81593617441674));
#14752=CARTESIAN_POINT('Ctrl Pts',(-16.3069412547017,8.32783199413537,6.70479502688772));
#14753=CARTESIAN_POINT('Ctrl Pts',(-17.113688980917,10.1912071986836,6.5936538793587));
#14754=CARTESIAN_POINT('Ctrl Pts',(-15.9856484096087,11.8795574241802,6.48251273182968));
#14755=CARTESIAN_POINT('Ctrl Pts',(-13.9553847534823,11.8474358513589,6.37137158430066));
#14756=CARTESIAN_POINT('Ctrl Pts',(-12.8813203358307,10.1242441489812,6.26023043677164));
#14757=CARTESIAN_POINT('Ctrl Pts',(-13.7466116524126,8.28732446652372,6.14908928924262));
#14758=CARTESIAN_POINT('Ctrl Pts',(-15.7592050398313,8.01812015126366,6.0379481417136));
#14759=CARTESIAN_POINT('Ctrl Pts',(-17.0768521850862,9.56305034803959,5.92680699418459));
#14760=CARTESIAN_POINT('Ctrl Pts',(-16.4934309318261,11.5079469533364,5.81566584665556));
#14761=CARTESIAN_POINT('Ctrl Pts',(-14.5429820570306,12.0725285497611,5.70452469912655));
#14762=CARTESIAN_POINT('Ctrl Pts',(-13.0108693337756,10.7399994434505,5.59338355159753));
#14763=CARTESIAN_POINT('Ctrl Pts',(-13.299528183005,8.73010410689258,5.4822424040685));
#14764=CARTESIAN_POINT('Ctrl Pts',(-15.1447317026798,7.8826212625554,5.37110125653949));
#14765=CARTESIAN_POINT('Ctrl Pts',(-16.857453544477,8.97330320320286,5.25996010901046));
#14766=CARTESIAN_POINT('Ctrl Pts',(-16.869935847247,11.0037827998243,5.14881896148144));
#14767=CARTESIAN_POINT('Ctrl Pts',(-15.1707528050564,12.115439307124,5.03767781395243));
#14768=CARTESIAN_POINT('Ctrl Pts',(-13.3152693958758,11.2907063081524,4.9265366664234));
#14769=CARTESIAN_POINT('Ctrl Pts',(-13.0019217745667,9.28451178389106,4.81539551889439));
#14770=CARTESIAN_POINT('Ctrl Pts',(-14.517535965151,7.93324688521165,4.70425437136536));
#14771=CARTESIAN_POINT('Ctrl Pts',(-16.4747786586417,8.47380607706747,4.59311322383635));
#14772=CARTESIAN_POINT('Ctrl Pts',(-17.082067274576,10.4113828466508,4.48197207630732));
#14773=CARTESIAN_POINT('Ctrl Pts',(-15.7835138235858,11.9723960227698,4.3708309287783));
#14774=CARTESIAN_POINT('Ctrl Pts',(-13.7677627953381,11.7279558599196,4.25968978124929));
#14775=CARTESIAN_POINT('Ctrl Pts',(-12.8799529867411,9.90181321903733,4.14854863372026));
#14776=CARTESIAN_POINT('Ctrl Pts',(-13.9327503963021,8.16554687555337,4.03740748619125));
#14777=CARTESIAN_POINT('Ctrl Pts',(-15.9624658985096,8.10846639559596,3.92626633866222));
#14778=CARTESIAN_POINT('Ctrl Pts',(-17.1111781690911,9.78282099379339,3.81512519113321));
#14779=CARTESIAN_POINT('Ctrl Pts',(-16.3274014108291,11.6559726679257,3.70398404360419));
#14780=CARTESIAN_POINT('Ctrl Pts',(-14.3285738809845,12.0133124320589,3.59284289607517));
#14781=CARTESIAN_POINT('Ctrl Pts',(-12.9443432751131,10.5277455938313,3.48170174854614));
#14782=CARTESIAN_POINT('Ctrl Pts',(-13.4417795631413,8.55910130385022,3.37056060101713));
#14783=CARTESIAN_POINT('Ctrl Pts',(-15.3655492335712,7.90939871324609,3.2594194534881));
#14784=CARTESIAN_POINT('Ctrl Pts',(-16.9547095878554,9.17334988687881,3.14827830595909));
#14785=CARTESIAN_POINT('Ctrl Pts',(-16.7546060664852,11.1939838918566,3.03713715843006));
#14786=CARTESIAN_POINT('Ctrl Pts',(-14.9484055215533,12.1216922472018,2.92599601090105));
#14787=CARTESIAN_POINT('Ctrl Pts',(-13.1894325225084,11.1072874025715,2.81485486337203));
#14788=CARTESIAN_POINT('Ctrl Pts',(-13.0877814098212,9.07931544657375,2.703713715843));
#14789=CARTESIAN_POINT('Ctrl Pts',(-14.7364995940206,7.8941017318555,2.59257256831399));
#14790=CARTESIAN_POINT('Ctrl Pts',(-16.6264156310847,8.63654403129957,2.48143142078497));
#14791=CARTESIAN_POINT('Ctrl Pts',(-17.0275751031823,10.627040023225,2.37029027325595));
#14792=CARTESIAN_POINT('Ctrl Pts',(-15.5727724836478,12.0435683605368,2.25914912572693));
#14793=CARTESIAN_POINT('Ctrl Pts',(-13.5936765853703,11.5894950300362,2.14800797819791));
#14794=CARTESIAN_POINT('Ctrl Pts',(-12.9018735256621,9.68046076138442,2.03686683066889));
#14795=CARTESIAN_POINT('Ctrl Pts',(-14.1306125185887,8.06392013594442,1.92572568313987));
#14796=CARTESIAN_POINT('Ctrl Pts',(-16.1551543835509,8.21959036228063,1.81458453561085));
#14797=CARTESIAN_POINT('Ctrl Pts',(-17.1223137052908,10.0049773967301,1.70344338808183));
#14798=CARTESIAN_POINT('Ctrl Pts',(-16.1467907563622,11.7858079010009,1.59230224055281));
#14799=CARTESIAN_POINT('Ctrl Pts',(-14.1215412996839,11.9319812661403,1.48116109302379));
#14800=CARTESIAN_POINT('Ctrl Pts',(-12.900397409555,10.3096937927621,1.37001994549477));
#14801=CARTESIAN_POINT('Ctrl Pts',(-13.6011482660932,8.40392790803455,1.25887879796575));
#14802=CARTESIAN_POINT('Ctrl Pts',(-15.5823497011553,7.95913741781259,1.14773765043673));
#14803=CARTESIAN_POINT('Ctrl Pts',(-17.0304970457477,9.38248327556005,1.03659650290771));
#14804=CARTESIAN_POINT('Ctrl Pts',(-16.6199964271269,11.3710573824967,0.925455355378691));
#14805=CARTESIAN_POINT('Ctrl Pts',(-14.7266369196359,12.1046626870771,0.814314207849671));
#14806=CARTESIAN_POINT('Ctrl Pts',(-13.0834609338788,10.9116597986998,0.70317306032065));
#14807=CARTESIAN_POINT('Ctrl Pts',(-13.1946908892948,8.88432077619087,0.592031912791632));
#14808=CARTESIAN_POINT('Ctrl Pts',(-14.958270785702,7.87791797902744,0.48089076526261));
#14809=CARTESIAN_POINT('Ctrl Pts',(-16.760355558866,8.81459080814426,0.36974961773359));
#14810=CARTESIAN_POINT('Ctrl Pts',(-16.9504828264524,10.8351650410851,0.258608470204571));
#14811=CARTESIAN_POINT('Ctrl Pts',(-15.3563881704699,12.0935554951319,0.14746732267555));
#14812=CARTESIAN_POINT('Ctrl Pts',(-13.433650537475,11.4309895668835,0.0363261751465318));
#14813=CARTESIAN_POINT('Ctrl Pts',(-13.1117433942273,10.1229835990773,-0.0377679232061492));
#14814=CARTESIAN_POINT('Ctrl Pts',(-13.2629299182875,9.54534954287515,-0.0748149723824891));
#14815=CARTESIAN_POINT('Ctrl Pts',(-15.4298642568859,8.39041225133515,8.22444491714747));
#14816=CARTESIAN_POINT('Ctrl Pts',(-15.9651061621278,8.53335653259092,8.18739786797113));
#14817=CARTESIAN_POINT('Ctrl Pts',(-16.8725061703686,9.39282251015386,8.11330376961845));
#14818=CARTESIAN_POINT('Ctrl Pts',(-16.5252008613007,11.2475121192479,8.00216262208942));
#14819=CARTESIAN_POINT('Ctrl Pts',(-14.7791873873764,11.9562183136467,7.89102147456041));
#14820=CARTESIAN_POINT('Ctrl Pts',(-13.236608893473,10.8762773263063,7.77988032703139));
#14821=CARTESIAN_POINT('Ctrl Pts',(-13.3074949738546,8.99320571730152,7.66873917950237));
#14822=CARTESIAN_POINT('Ctrl Pts',(-14.9279806834685,8.03223963225308,7.55759803197335));
#14823=CARTESIAN_POINT('Ctrl Pts',(-16.6142107796781,8.87221235889479,7.44645688444433));
#14824=CARTESIAN_POINT('Ctrl Pts',(-16.8229486354888,10.7446572483991,7.33531573691531));
#14825=CARTESIAN_POINT('Ctrl Pts',(-15.3629836590177,11.9354001238949,7.22417458938629));
#14826=CARTESIAN_POINT('Ctrl Pts',(-13.5707824167768,11.3545915031861,7.11303344185727));
#14827=CARTESIAN_POINT('Ctrl Pts',(-13.0868177386564,9.53382414959064,7.00189229432825));
#14828=CARTESIAN_POINT('Ctrl Pts',(-14.3541110197329,8.13978565920112,6.89075114679923));
#14829=CARTESIAN_POINT('Ctrl Pts',(-16.2126221545457,8.44850871243116,6.77960999927022));
#14830=CARTESIAN_POINT('Ctrl Pts',(-16.9611486567268,10.177408192142,6.66846885174119));
#14831=CARTESIAN_POINT('Ctrl Pts',(-15.9145163134031,11.7439138638423,6.55732770421217));
#14832=CARTESIAN_POINT('Ctrl Pts',(-14.0307723577119,11.7141104348804,6.44618655668315));
#14833=CARTESIAN_POINT('Ctrl Pts',(-13.0342208267474,10.1152777197026,6.33504540915413));
#14834=CARTESIAN_POINT('Ctrl Pts',(-13.8370659560511,8.41092452474786,6.22390426162511));
#14835=CARTESIAN_POINT('Ctrl Pts',(-15.7044148677917,8.16114809783556,6.11276311409609));
#14836=CARTESIAN_POINT('Ctrl Pts',(-16.9269702921169,9.59458405151565,6.00162196656707));
#14837=CARTESIAN_POINT('Ctrl Pts',(-16.3856532783713,11.399121710266,5.89048081903805));
#14838=CARTESIAN_POINT('Ctrl Pts',(-14.5759640453036,11.9229586841242,5.77933967150902));
#14839=CARTESIAN_POINT('Ctrl Pts',(-13.154420556033,10.6865952974178,5.66819852398002));
#14840=CARTESIAN_POINT('Ctrl Pts',(-13.4222475256247,8.82174972409137,5.55705737645099));
#14841=CARTESIAN_POINT('Ctrl Pts',(-15.1342867313303,8.0354278684275,5.44591622892198));
#14842=CARTESIAN_POINT('Ctrl Pts',(-16.7234051729329,9.04739767199292,5.33477508139295));
#14843=CARTESIAN_POINT('Ctrl Pts',(-16.7349866551335,10.9313419842246,5.22363393386394));
#14844=CARTESIAN_POINT('Ctrl Pts',(-15.1584299474956,11.9627726657085,5.11249278633491));
#14845=CARTESIAN_POINT('Ctrl Pts',(-13.4368527294913,11.1975588486834,5.00135163880589));
#14846=CARTESIAN_POINT('Ctrl Pts',(-13.1461187226592,9.3361470081009,4.89021049127687));
#14847=CARTESIAN_POINT('Ctrl Pts',(-14.5523543423817,8.08239995030172,4.77906934374785));
#14848=CARTESIAN_POINT('Ctrl Pts',(-16.3683470990655,8.58394816414039,4.66792819621883));
#14849=CARTESIAN_POINT('Ctrl Pts',(-16.9318090199714,10.3816942437575,4.55678704868981));
#14850=CARTESIAN_POINT('Ctrl Pts',(-15.7269693396356,11.8300525032354,4.44564590116079));
#14851=CARTESIAN_POINT('Ctrl Pts',(-13.8566906671183,11.6032530538596,4.33450475363177));
#14852=CARTESIAN_POINT('Ctrl Pts',(-13.0329521562598,9.90889914489231,4.22336360610275));
#14853=CARTESIAN_POINT('Ctrl Pts',(-14.0097714727281,8.29793535694355,4.11222245857373));
#14854=CARTESIAN_POINT('Ctrl Pts',(-15.8930068335733,8.24497425074277,4.00108131104471));
#14855=CARTESIAN_POINT('Ctrl Pts',(-16.9588190447147,9.7984943290443,3.8899401635157));
#14856=CARTESIAN_POINT('Ctrl Pts',(-16.2316057458252,11.5364647318499,3.77879901598667));
#14857=CARTESIAN_POINT('Ctrl Pts',(-14.3770292397384,11.8680160644972,3.66765786845765));
#14858=CARTESIAN_POINT('Ctrl Pts',(-13.0926955379431,10.4896593452395,3.55651672092863));
#14859=CARTESIAN_POINT('Ctrl Pts',(-13.5542329338804,8.66308782041927,3.44537557339962));
#14860=CARTESIAN_POINT('Ctrl Pts',(-15.3391683425793,8.06027284889848,3.33423442587059));
#14861=CARTESIAN_POINT('Ctrl Pts',(-16.813642459758,9.2330074227726,3.22309327834158));
#14862=CARTESIAN_POINT('Ctrl Pts',(-16.6279799731365,11.1078166782381,3.11195213081255));
#14863=CARTESIAN_POINT('Ctrl Pts',(-14.9521289825448,11.9685743447375,3.00081098328354));
#14864=CARTESIAN_POINT('Ctrl Pts',(-13.320097228848,11.0273768855158,2.88966983575452));
#14865=CARTESIAN_POINT('Ctrl Pts',(-13.2257820552813,9.14575924295271,2.77852868822549));
#14866=CARTESIAN_POINT('Ctrl Pts',(-14.7555158436747,8.046079817295,2.66738754069648));
#14867=CARTESIAN_POINT('Ctrl Pts',(-16.5090407618993,8.73494167511676,2.55624639316746));
#14868=CARTESIAN_POINT('Ctrl Pts',(-16.8812494297499,10.5817879122065,2.44510524563843));
#14869=CARTESIAN_POINT('Ctrl Pts',(-15.5314367426132,11.8960884885995,2.33396409810942));
#14870=CARTESIAN_POINT('Ctrl Pts',(-13.6951678792743,11.4747846401115,2.22282295058039));
#14871=CARTESIAN_POINT('Ctrl Pts',(-13.0532907376914,9.70352121137968,2.11168180305138));
#14872=CARTESIAN_POINT('Ctrl Pts',(-14.1933543171498,8.20364279750315,2.00054065552236));
#14873=CARTESIAN_POINT('Ctrl Pts',(-16.0717894108669,8.34807864309253,1.88939950799334));
#14874=CARTESIAN_POINT('Ctrl Pts',(-16.9691509535515,10.0046181888628,1.77825836046432));
#14875=CARTESIAN_POINT('Ctrl Pts',(-16.0640293684129,11.6569300393006,1.6671172129353));
#14876=CARTESIAN_POINT('Ctrl Pts',(-14.1849377483306,11.7925543914548,1.55597606540628));
#14877=CARTESIAN_POINT('Ctrl Pts',(-13.0519211496647,10.287343867123,1.44483491787726));
#14878=CARTESIAN_POINT('Ctrl Pts',(-13.7021003450938,8.51911295017527,1.33369377034824));
#14879=CARTESIAN_POINT('Ctrl Pts',(-15.5403227932193,8.1064220196273,1.22255262281922));
#14880=CARTESIAN_POINT('Ctrl Pts',(-16.8839605020926,9.42704811087374,1.1114114752902));
#14881=CARTESIAN_POINT('Ctrl Pts',(-16.5030848178921,11.2721111612231,1.00027032776118));
#14882=CARTESIAN_POINT('Ctrl Pts',(-14.7463649369917,11.9527737708287,0.88912918023216));
#14883=CARTESIAN_POINT('Ctrl Pts',(-13.2217733786655,10.8458672991881,0.777988032703139));
#14884=CARTESIAN_POINT('Ctrl Pts',(-13.3249761107709,8.96483691268427,0.666846885174121));
#14885=CARTESIAN_POINT('Ctrl Pts',(-14.9612822920943,8.03106401061478,0.555705737645099));
#14886=CARTESIAN_POINT('Ctrl Pts',(-16.6333145371908,8.90013920436348,0.444564590116079));
#14887=CARTESIAN_POINT('Ctrl Pts',(-16.8097207345076,10.7748930014097,0.33342344258706));
#14888=CARTESIAN_POINT('Ctrl Pts',(-15.3306684134234,11.9424681607034,0.222282295058039));
#14889=CARTESIAN_POINT('Ctrl Pts',(-13.5466905622686,11.3277181705637,0.111141147529021));
#14890=CARTESIAN_POINT('Ctrl Pts',(-13.2480147555294,10.1141081409362,0.0370470491763399));
#14891=CARTESIAN_POINT('Ctrl Pts',(-13.3882904778579,9.57816067485776,0.));
#14892=CARTESIAN_POINT('Ctrl Pts',(-16.6638185641669,10.0009395545784,7.3785196366098));
#14893=CARTESIAN_POINT('Ctrl Pts',(-16.6649347763355,10.2169537916664,7.36411833671164));
#14894=CARTESIAN_POINT('Ctrl Pts',(-16.6258964192002,10.4325814095807,7.34971703681347));
#14895=CARTESIAN_POINT('Ctrl Pts',(-16.5448314967751,10.6310402460644,7.33531573691531));
#14896=CARTESIAN_POINT('Ctrl Pts',(-16.3362936433318,11.141571540231,7.29826868773897));
#14897=CARTESIAN_POINT('Ctrl Pts',(-15.8496386511747,11.538485832063,7.26122163856263));
#14898=CARTESIAN_POINT('Ctrl Pts',(-15.3076109480561,11.6401415411941,7.22417458938629));
#14899=CARTESIAN_POINT('Ctrl Pts',(-14.7655832449374,11.7417972503253,7.18712754020995));
#14900=CARTESIAN_POINT('Ctrl Pts',(-14.1681828308571,11.5481943767557,7.15008049103361));
#14901=CARTESIAN_POINT('Ctrl Pts',(-13.7888218441302,11.1479317143716,7.11303344185727));
#14902=CARTESIAN_POINT('Ctrl Pts',(-13.4094608574033,10.7476690519876,7.07598639268093));
#14903=CARTESIAN_POINT('Ctrl Pts',(-13.2481392980299,10.1407466007891,7.03893934350459));
#14904=CARTESIAN_POINT('Ctrl Pts',(-13.3786940651892,9.60494562679162,7.00189229432825));
#14905=CARTESIAN_POINT('Ctrl Pts',(-13.5092488323486,9.06914465279414,6.96484524515191));
#14906=CARTESIAN_POINT('Ctrl Pts',(-13.9316799260408,8.60446515599763,6.92779819597557));
#14907=CARTESIAN_POINT('Ctrl Pts',(-14.452647328689,8.42357924980438,6.89075114679923));
#14908=CARTESIAN_POINT('Ctrl Pts',(-14.9736147313372,8.24269334361113,6.85370409762289));
#14909=CARTESIAN_POINT('Ctrl Pts',(-15.5931184429414,8.34560102802114,6.81665704844655));
#14910=CARTESIAN_POINT('Ctrl Pts',(-16.0276247157737,8.68520478351129,6.77960999927021));
#14911=CARTESIAN_POINT('Ctrl Pts',(-16.4228374490899,8.99409728252362,6.74591321171674));
#14912=CARTESIAN_POINT('Ctrl Pts',(-16.6649994289874,9.49881147642293,6.71221642416327));
#14913=CARTESIAN_POINT('Ctrl Pts',(-16.6681787596498,10.0008675363463,6.67851963660979));
#14914=CARTESIAN_POINT('Ctrl Pts',(-15.5301702171886,8.01482567432828,8.));
#14915=CARTESIAN_POINT('Ctrl Pts',(-15.6001784828994,8.04074713960098,8.));
#14916=CARTESIAN_POINT('Ctrl Pts',(-15.6685003719384,8.07074116686246,8.));
#14917=CARTESIAN_POINT('Ctrl Pts',(-15.7349165600646,8.10452089866272,8.));
#14918=CARTESIAN_POINT('Ctrl Pts',(-15.7995896602114,8.13741408388292,8.));
#14919=CARTESIAN_POINT('Ctrl Pts',(-15.8624562004235,8.17389779453761,8.));
#14920=CARTESIAN_POINT('Ctrl Pts',(-15.9232827418904,8.2137409613008,8.));
#14921=CARTESIAN_POINT('Ctrl Pts',(-15.9368594118801,8.22263407791475,8.));
#14922=CARTESIAN_POINT('Ctrl Pts',(-15.9503360961863,8.23169590343848,8.));
#14923=CARTESIAN_POINT('Ctrl Pts',(-15.963704238615,8.24092008435083,8.));
#14924=CARTESIAN_POINT('Ctrl Pts',(-16.025045951378,8.28324661243913,8.));
#14925=CARTESIAN_POINT('Ctrl Pts',(-16.0839845137402,8.32890401789326,8.));
#14926=CARTESIAN_POINT('Ctrl Pts',(-16.1402813323094,8.37762295878361,8.));
#14927=CARTESIAN_POINT('Ctrl Pts',(-16.1798064165517,8.41182773787818,8.));
#14928=CARTESIAN_POINT('Ctrl Pts',(-16.2180286078769,8.4475424782692,8.));
#14929=CARTESIAN_POINT('Ctrl Pts',(-16.2548524753579,8.48468236692164,8.));
#14930=CARTESIAN_POINT('Ctrl Pts',(-16.2688611594934,8.4988112731053,8.));
#14931=CARTESIAN_POINT('Ctrl Pts',(-16.2826673549471,8.5131464868812,8.));
#14932=CARTESIAN_POINT('Ctrl Pts',(-16.2962653477309,8.52768352141437,8.));
#14933=CARTESIAN_POINT('Ctrl Pts',(-16.3091902201709,8.54150095167668,8.));
#14934=CARTESIAN_POINT('Ctrl Pts',(-16.3219308141586,8.55550525640342,8.));
#14935=CARTESIAN_POINT('Ctrl Pts',(-16.3344602231157,8.56966738394869,8.));
#14936=CARTESIAN_POINT('Ctrl Pts',(-16.3825593087518,8.62403430484007,8.));
#14937=CARTESIAN_POINT('Ctrl Pts',(-16.4276039578114,8.68077946858957,8.));
#14938=CARTESIAN_POINT('Ctrl Pts',(-16.4693716176289,8.73965492650984,8.));
#14939=CARTESIAN_POINT('Ctrl Pts',(-16.5102413746783,8.79726470574788,8.));
#14940=CARTESIAN_POINT('Ctrl Pts',(-16.5479738782328,8.85691503747699,8.));
#14941=CARTESIAN_POINT('Ctrl Pts',(-16.5823154929831,8.91839275710173,8.));
#14942=CARTESIAN_POINT('Ctrl Pts',(-16.6159043360375,8.97852287884562,8.));
#14943=CARTESIAN_POINT('Ctrl Pts',(-16.6462495962695,9.04040187061098,8.));
#14944=CARTESIAN_POINT('Ctrl Pts',(-16.6730657146258,9.10383727944419,8.));
#14945=CARTESIAN_POINT('Ctrl Pts',(-16.6817773057965,9.12444515938257,8.));
#14946=CARTESIAN_POINT('Ctrl Pts',(-16.6901160396164,9.14521730998075,8.));
#14947=CARTESIAN_POINT('Ctrl Pts',(-16.6980709212983,9.1661471082209,8.));
#14948=CARTESIAN_POINT('Ctrl Pts',(-16.7025653313911,9.17797218623112,8.));
#14949=CARTESIAN_POINT('Ctrl Pts',(-16.7069375536196,9.18984887021962,8.));
#14950=CARTESIAN_POINT('Ctrl Pts',(-16.711179782049,9.20175897829843,8.));
#14951=CARTESIAN_POINT('Ctrl Pts',(-16.734096120241,9.26609687739624,8.));
#14952=CARTESIAN_POINT('Ctrl Pts',(-16.7532666512879,9.33152043561446,8.));
#14953=CARTESIAN_POINT('Ctrl Pts',(-16.7684630804155,9.39783015254818,8.));
#14954=CARTESIAN_POINT('Ctrl Pts',(-16.770660460792,9.40741843605486,8.));
#14955=CARTESIAN_POINT('Ctrl Pts',(-16.7727746597823,9.41702526171543,8.));
#14956=CARTESIAN_POINT('Ctrl Pts',(-16.7748048961907,9.42665003738271,8.));
#14957=CARTESIAN_POINT('Ctrl Pts',(-16.7891235197531,9.49453057537518,8.));
#14958=CARTESIAN_POINT('Ctrl Pts',(-16.7992700679188,9.56330447632077,8.));
#14959=CARTESIAN_POINT('Ctrl Pts',(-16.8053412035889,9.63261589594071,8.));
#14960=CARTESIAN_POINT('Ctrl Pts',(-16.8110052242317,9.69727946678601,8.));
#14961=CARTESIAN_POINT('Ctrl Pts',(-16.813121294483,9.76241159112694,8.));
#14962=CARTESIAN_POINT('Ctrl Pts',(-16.8117297557015,9.82771097976151,8.));
#14963=CARTESIAN_POINT('Ctrl Pts',(-16.8114209501081,9.84220199986072,8.));
#14964=CARTESIAN_POINT('Ctrl Pts',(-16.8109392718932,9.85670118401844,8.));
#14965=CARTESIAN_POINT('Ctrl Pts',(-16.8102849391738,9.87120509964638,8.));
#14966=CARTESIAN_POINT('Ctrl Pts',(-16.8097777153087,9.88244820567933,8.));
#14967=CARTESIAN_POINT('Ctrl Pts',(-16.8091667038368,9.89369326677607,8.));
#14968=CARTESIAN_POINT('Ctrl Pts',(-16.8084530650648,9.90492595177548,8.));
#14969=CARTESIAN_POINT('Ctrl Pts',(-16.8041173130474,9.97317075371321,8.));
#14970=CARTESIAN_POINT('Ctrl Pts',(-16.7959925101146,10.0410849030563,8.));
#14971=CARTESIAN_POINT('Ctrl Pts',(-16.7841889169068,10.1083325876079,8.));
#14972=CARTESIAN_POINT('Ctrl Pts',(-16.772440263585,10.1752672674618,8.));
#14973=CARTESIAN_POINT('Ctrl Pts',(-16.7570464996027,10.2415426993447,8.));
#14974=CARTESIAN_POINT('Ctrl Pts',(-16.7380692198235,10.3068079361699,8.));
#14975=CARTESIAN_POINT('Ctrl Pts',(-16.7194994223666,10.3706717903636,8.));
#14976=CARTESIAN_POINT('Ctrl Pts',(-16.6974978125829,10.4335691780139,8.));
#14977=CARTESIAN_POINT('Ctrl Pts',(-16.6720845678673,10.4951388738486,8.));
#14978=CARTESIAN_POINT('Ctrl Pts',(-16.6666982087073,10.5081886240417,8.));
#14979=CARTESIAN_POINT('Ctrl Pts',(-16.6611584673709,10.5211785874357,8.));
#14980=CARTESIAN_POINT('Ctrl Pts',(-16.6554653473059,10.5341050800545,8.));
#14981=CARTESIAN_POINT('Ctrl Pts',(-16.6501415194561,10.5461930776059,8.));
#14982=CARTESIAN_POINT('Ctrl Pts',(-16.6446827914777,10.5582269434921,8.));
#14983=CARTESIAN_POINT('Ctrl Pts',(-16.6390983290274,10.5701847169649,8.));
#14984=CARTESIAN_POINT('Ctrl Pts',(-16.6114456278208,10.6293962775905,8.));
#14985=CARTESIAN_POINT('Ctrl Pts',(-16.5806669622525,10.6868526416772,8.));
#14986=CARTESIAN_POINT('Ctrl Pts',(-16.5468263628228,10.7422402982346,8.));
#14987=CARTESIAN_POINT('Ctrl Pts',(-16.5136306620755,10.796572434874,8.));
#14988=CARTESIAN_POINT('Ctrl Pts',(-16.4774881013739,10.8489146747283,8.));
#14989=CARTESIAN_POINT('Ctrl Pts',(-16.438424559325,10.8989353653364,8.));
#14990=CARTESIAN_POINT('Ctrl Pts',(-16.4006315217879,10.9473291806082,8.));
#14991=CARTESIAN_POINT('Ctrl Pts',(-16.360103934621,10.9935504630778,8.));
#14992=CARTESIAN_POINT('Ctrl Pts',(-16.316839891742,11.0372567981819,8.));
#14993=CARTESIAN_POINT('Ctrl Pts',(-16.3096319230205,11.0445384546198,8.));
#14994=CARTESIAN_POINT('Ctrl Pts',(-16.3023479491257,11.0517501974988,8.));
#14995=CARTESIAN_POINT('Ctrl Pts',(-16.2949879039586,11.0588903115368,8.));
#14996=CARTESIAN_POINT('Ctrl Pts',(-16.2872272673507,11.0664190466369,8.));
#14997=CARTESIAN_POINT('Ctrl Pts',(-16.2793820521969,11.0738681429984,8.));
#14998=CARTESIAN_POINT('Ctrl Pts',(-16.271453753893,11.081236856086,8.));
#14999=CARTESIAN_POINT('Origin',(15.,-10.,9.54592528053767));
#15000=CARTESIAN_POINT('Ctrl Pts',(12.9434529369556,-9.99851181185547,7.79592528053768));
#15001=CARTESIAN_POINT('Ctrl Pts',(12.9426313731505,-9.9001452310185,7.79057696270225));
#15002=CARTESIAN_POINT('Ctrl Pts',(12.9937603976267,-9.12123426690962,7.74818159569048));
#15003=CARTESIAN_POINT('Ctrl Pts',(13.9893910509183,-7.79139173496881,7.66873917950237));
#15004=CARTESIAN_POINT('Ctrl Pts',(16.3073489540956,-7.95337086724347,7.55759803197335));
#15005=CARTESIAN_POINT('Ctrl Pts',(17.4286195209518,-9.9883529914062,7.44645688444433));
#15006=CARTESIAN_POINT('Ctrl Pts',(16.3268235646033,-12.0342028814299,7.33531573691532));
#15007=CARTESIAN_POINT('Ctrl Pts',(14.0105079567266,-12.2179173173397,7.22417458938628));
#15008=CARTESIAN_POINT('Ctrl Pts',(12.9977472715797,-10.8922265383227,7.14437777059375));
#15009=CARTESIAN_POINT('Ctrl Pts',(12.9427343868833,-10.1065382000683,7.10162800097755));
#15010=CARTESIAN_POINT('Ctrl Pts',(12.9436342636416,-10.0016028715607,7.09592528053768));
#15011=CARTESIAN_POINT('Ctrl Pts',(12.9473113312417,-10.0024712008536,7.85407471946232));
#15012=CARTESIAN_POINT('Ctrl Pts',(12.950875636899,-9.53216658348607,7.82862238128887));
#15013=CARTESIAN_POINT('Ctrl Pts',(13.3435593652589,-8.37020036788621,7.76612299393908));
#15014=CARTESIAN_POINT('Ctrl Pts',(15.2723376840439,-7.58731246609672,7.66657655741293));
#15015=CARTESIAN_POINT('Ctrl Pts',(17.1748664515305,-8.91924865455582,7.55543540988393));
#15016=CARTESIAN_POINT('Ctrl Pts',(17.0874396573092,-11.2417232863365,7.44429426235489));
#15017=CARTESIAN_POINT('Ctrl Pts',(15.0888244971834,-12.4269237058338,7.33315311482589));
#15018=CARTESIAN_POINT('Ctrl Pts',(13.2786047494337,-11.5251874796858,7.23641326719502));
#15019=CARTESIAN_POINT('Ctrl Pts',(12.9501054372198,-10.417780757041,7.1767204687405));
#15020=CARTESIAN_POINT('Ctrl Pts',(12.9479406426496,-9.99884121834684,7.15407471946232));
#15021=CARTESIAN_POINT('Ctrl Pts',(16.2690708798524,-8.92064134695149,8.));
#15022=CARTESIAN_POINT('Ctrl Pts',(16.6279938291456,-9.34264997380806,7.96295295082366));
#15023=CARTESIAN_POINT('Ctrl Pts',(16.8854605771123,-10.5656667587716,7.88885885247099));
#15024=CARTESIAN_POINT('Ctrl Pts',(15.5448841833265,-11.8935743297638,7.77771770494195));
#15025=CARTESIAN_POINT('Ctrl Pts',(13.705710965359,-11.4833634608872,7.66657655741295));
#15026=CARTESIAN_POINT('Ctrl Pts',(13.0512228097228,-9.71772794909045,7.55543540988392));
#15027=CARTESIAN_POINT('Ctrl Pts',(14.1805939850735,-8.20925106726273,7.44429426235491));
#15028=CARTESIAN_POINT('Ctrl Pts',(16.0600040674161,-8.34058443354548,7.33315311482588));
#15029=CARTESIAN_POINT('Ctrl Pts',(16.9691349905856,-9.99055655611766,7.22201196729687));
#15030=CARTESIAN_POINT('Ctrl Pts',(16.075794164073,-11.649340309265,7.11087081976784));
#15031=CARTESIAN_POINT('Ctrl Pts',(14.1977156617139,-11.7982967517645,6.99972967223883));
#15032=CARTESIAN_POINT('Ctrl Pts',(13.0540156107808,-10.3012080182464,6.88858852470979));
#15033=CARTESIAN_POINT('Ctrl Pts',(13.6915932046182,-8.52838237790974,6.77744737718079));
#15034=CARTESIAN_POINT('Ctrl Pts',(15.5268344070607,-8.10262919057289,6.66630622965176));
#15035=CARTESIAN_POINT('Ctrl Pts',(16.8798323474503,-9.41364810779719,6.55516508212274));
#15036=CARTESIAN_POINT('Ctrl Pts',(16.5121060130156,-11.2613935227057,6.44402393459372));
#15037=CARTESIAN_POINT('Ctrl Pts',(14.7602576499653,-11.9545075482124,6.33288278706471));
#15038=CARTESIAN_POINT('Ctrl Pts',(13.2278599385176,-10.8585434774938,6.22174163953568));
#15039=CARTESIAN_POINT('Ctrl Pts',(13.3176091852349,-8.97670221714518,6.11060049200667));
#15040=CARTESIAN_POINT('Ctrl Pts',(14.9473524645216,-8.03154751397968,5.99945934447764));
#15041=CARTESIAN_POINT('Ctrl Pts',(16.6252872186854,-8.88823627676186,5.88831819694863));
#15042=CARTESIAN_POINT('Ctrl Pts',(16.8154983086942,-10.7625896568447,5.7771770494196));
#15043=CARTESIAN_POINT('Ctrl Pts',(15.3438740247519,-11.9388985839416,5.66603590189059));
#15044=CARTESIAN_POINT('Ctrl Pts',(13.5574810535658,-11.3404164190708,5.55489475436156));
#15045=CARTESIAN_POINT('Ctrl Pts',(13.091512894956,-9.51497005045939,5.44375360683255));
#15046=CARTESIAN_POINT('Ctrl Pts',(14.3724983786311,-8.13350092582179,5.33261245930352));
#15047=CARTESIAN_POINT('Ctrl Pts',(16.2278740377661,-8.46055125795619,5.22147131177451));
#15048=CARTESIAN_POINT('Ctrl Pts',(16.9593023477033,-10.1967521063248,5.11033016424548));
#15049=CARTESIAN_POINT('Ctrl Pts',(15.8972627511728,-11.7528538547388,4.99918901671647));
#15050=CARTESIAN_POINT('Ctrl Pts',(14.0139043062234,-11.7044624853229,4.88804786918744));
#15051=CARTESIAN_POINT('Ctrl Pts',(13.0331788732669,-10.0958735439955,4.77690672165843));
#15052=CARTESIAN_POINT('Ctrl Pts',(13.8528037398514,-8.39952575101248,4.66576557412941));
#15053=CARTESIAN_POINT('Ctrl Pts',(15.7225267076418,-8.16818880946363,4.55462442660038));
#15054=CARTESIAN_POINT('Ctrl Pts',(16.930877292936,-9.61361940961134,4.44348327907137));
#15055=CARTESIAN_POINT('Ctrl Pts',(16.3717791430773,-11.4127275263198,4.33234213154234));
#15056=CARTESIAN_POINT('Ctrl Pts',(14.5570086000468,-11.9186807187697,4.22120098401333));
#15057=CARTESIAN_POINT('Ctrl Pts',(13.1477348705092,-10.6683494378538,4.1100598364843));
#15058=CARTESIAN_POINT('Ctrl Pts',(13.4339514097027,-8.80623750526538,3.99891868895529));
#15059=CARTESIAN_POINT('Ctrl Pts',(15.1536669134528,-8.03684856398734,3.88777754142627));
#15060=CARTESIAN_POINT('Ctrl Pts',(16.7327217999743,-9.0644508324513,3.77663639389725));
#15061=CARTESIAN_POINT('Ctrl Pts',(16.7257116553616,-10.948417821193,3.66549524636823));
#15062=CARTESIAN_POINT('Ctrl Pts',(15.139053288841,-11.9642406328842,3.55435409883921));
#15063=CARTESIAN_POINT('Ctrl Pts',(13.4251110393005,-11.1820752270774,3.44321295131019));
#15064=CARTESIAN_POINT('Ctrl Pts',(13.1527598798706,-9.31788489271265,3.33207180378117));
#15065=CARTESIAN_POINT('Ctrl Pts',(14.5712992942719,-8.07807575957374,3.22093065625215));
#15066=CARTESIAN_POINT('Ctrl Pts',(16.3822543856635,-8.59752009130784,3.10978950872313));
#15067=CARTESIAN_POINT('Ctrl Pts',(16.927948460973,-10.400739083237,2.9986483611941));
#15068=CARTESIAN_POINT('Ctrl Pts',(15.7088747381036,-11.8371373619946,2.88750721366509));
#15069=CARTESIAN_POINT('Ctrl Pts',(13.8409251059329,-11.5918927321457,2.77636606613606));
#15070=CARTESIAN_POINT('Ctrl Pts',(13.0339468067845,-9.88949243235736,2.66522491860705));
#15071=CARTESIAN_POINT('Ctrl Pts',(14.0266158712758,-8.28824639040892,2.55408377107803));
#15072=CARTESIAN_POINT('Ctrl Pts',(15.910282283518,-8.25387192822464,2.44294262354901));
#15073=CARTESIAN_POINT('Ctrl Pts',(16.960712282471,-9.8178340661976,2.33180147601999));
#15074=CARTESIAN_POINT('Ctrl Pts',(16.21638377583,-11.5485437020743,2.22066032849097));
#15075=CARTESIAN_POINT('Ctrl Pts',(14.3586256526202,-11.8617776479034,2.10951918096195));
#15076=CARTESIAN_POINT('Ctrl Pts',(13.0879562476019,-10.470813957433,1.99837803343293));
#15077=CARTESIAN_POINT('Ctrl Pts',(13.5674961034851,-8.64888575390523,1.88723688590391));
#15078=CARTESIAN_POINT('Ctrl Pts',(15.358293382976,-8.06371417284865,1.77609573837489));
#15079=CARTESIAN_POINT('Ctrl Pts',(16.8211230807301,-9.25094197098372,1.66495459084587));
#15080=CARTESIAN_POINT('Ctrl Pts',(16.6169686796854,-11.1238280959179,1.55381344331685));
#15081=CARTESIAN_POINT('Ctrl Pts',(14.9327051361131,-11.9680059836581,1.44267229578783));
#15082=CARTESIAN_POINT('Ctrl Pts',(13.3100405366278,-11.0107498334803,1.33153114825881));
#15083=CARTESIAN_POINT('Ctrl Pts',(13.234298236499,-9.12829163226479,1.22039000072979));
#15084=CARTESIAN_POINT('Ctrl Pts',(14.7748090948109,-8.04376393624155,1.10924885320077));
#15085=CARTESIAN_POINT('Ctrl Pts',(16.5214516331146,-8.74989132634765,0.998107705671752));
#15086=CARTESIAN_POINT('Ctrl Pts',(16.875415892384,-10.6003305289044,0.886966558142729));
#15087=CARTESIAN_POINT('Ctrl Pts',(15.5127017026779,-11.9012281112315,0.775825410613712));
#15088=CARTESIAN_POINT('Ctrl Pts',(13.6806746106472,-11.4618608197188,0.66468426308469));
#15089=CARTESIAN_POINT('Ctrl Pts',(13.0563175150209,-9.68427830710207,0.553543115555672));
#15090=CARTESIAN_POINT('Ctrl Pts',(14.2111078511261,-8.19586091928163,0.442401968026651));
#15091=CARTESIAN_POINT('Ctrl Pts',(16.0880628102433,-8.35855938932811,0.331260820497632));
#15092=CARTESIAN_POINT('Ctrl Pts',(16.9689629508152,-10.0243915228465,0.220119672968611));
#15093=CARTESIAN_POINT('Ctrl Pts',(16.0477169744579,-11.6666854543434,0.108978525439592));
#15094=CARTESIAN_POINT('Ctrl Pts',(14.1671160606488,-11.7857286633614,-0.00216262208942931));
#15095=CARTESIAN_POINT('Ctrl Pts',(13.0494868752983,-10.2654035044801,-0.113303769618448));
#15096=CARTESIAN_POINT('Ctrl Pts',(13.4941166421103,-9.09734376582132,-0.187397867971128));
#15097=CARTESIAN_POINT('Ctrl Pts',(13.9143317362933,-8.73632265938643,-0.224444917147468));
#15098=CARTESIAN_POINT('Ctrl Pts',(16.3677806246588,-8.83668763019027,8.07481497238249));
#15099=CARTESIAN_POINT('Ctrl Pts',(16.7546210002301,-9.29152055750512,8.03776792320615));
#15100=CARTESIAN_POINT('Ctrl Pts',(17.0321137982713,-10.609664948542,7.96367382485346));
#15101=CARTESIAN_POINT('Ctrl Pts',(15.5872658812593,-12.04085864763,7.85253267732446));
#15102=CARTESIAN_POINT('Ctrl Pts',(13.6050397244193,-11.5987411210352,7.74139152979541));
#15103=CARTESIAN_POINT('Ctrl Pts',(12.8996447519557,-9.69577251495858,7.63025038226642));
#15104=CARTESIAN_POINT('Ctrl Pts',(14.1168596736884,-8.06996462316475,7.51910923473738));
#15105=CARTESIAN_POINT('Ctrl Pts',(16.142452362976,-8.21151324477814,7.40796808720838));
#15106=CARTESIAN_POINT('Ctrl Pts',(17.1222965007077,-9.98982203454717,7.29682693967935));
#15107=CARTESIAN_POINT('Ctrl Pts',(16.1594706309165,-11.77762783332,7.18568579215033));
#15108=CARTESIAN_POINT('Ctrl Pts',(14.1353130933848,-11.9381702736228,7.07454464462131));
#15109=CARTESIAN_POINT('Ctrl Pts',(12.9026547801867,-10.324636312983,6.9634034970923));
#15110=CARTESIAN_POINT('Ctrl Pts',(13.5898238685428,-8.41391832216992,6.85226234956327));
#15111=CARTESIAN_POINT('Ctrl Pts',(15.5678121733162,-7.95504957829503,6.74112120203425));
#15112=CARTESIAN_POINT('Ctrl Pts',(17.026047798645,-9.36804100533744,6.62998005450523));
#15113=CARTESIAN_POINT('Ctrl Pts',(16.6297193008426,-11.3595061141326,6.51883890697621));
#15114=CARTESIAN_POINT('Ctrl Pts',(14.7416102232794,-12.1065313195945,6.4076977594472));
#15115=CARTESIAN_POINT('Ctrl Pts',(13.0900209131272,-10.9253219442557,6.29655661191817));
#15116=CARTESIAN_POINT('Ctrl Pts',(13.1867509560953,-8.89710897723226,6.18541546438916));
#15117=CARTESIAN_POINT('Ctrl Pts',(14.9432574806446,-7.87843908982193,6.07427431686013));
#15118=CARTESIAN_POINT('Ctrl Pts',(16.7517038665974,-8.80176205759242,5.96313316933111));
#15119=CARTESIAN_POINT('Ctrl Pts',(16.9567097867864,-10.8219047286931,5.8519920218021));
#15120=CARTESIAN_POINT('Ctrl Pts',(15.3706209289381,-12.0897082727185,5.74085087427307));
#15121=CARTESIAN_POINT('Ctrl Pts',(13.4452803251892,-11.4446754992856,5.62970972674406));
#15122=CARTESIAN_POINT('Ctrl Pts',(12.9430686448388,-9.47724388141499,5.51856857921503));
#15123=CARTESIAN_POINT('Ctrl Pts',(14.3236906044599,-7.98832255145469,5.40742743168601));
#15124=CARTESIAN_POINT('Ctrl Pts',(16.3233794463658,-8.340811222248,5.29628628415699));
#15125=CARTESIAN_POINT('Ctrl Pts',(17.1116990639237,-10.2120557040307,5.18514513662797));
#15126=CARTESIAN_POINT('Ctrl Pts',(15.9670528461145,-11.8891927775139,5.07400398909896));
#15127=CARTESIAN_POINT('Ctrl Pts',(13.9372046861842,-11.8370374735521,4.96286284156993));
#15128=CARTESIAN_POINT('Ctrl Pts',(12.8801973380494,-10.1033306949015,4.85172169404091));
#15129=CARTESIAN_POINT('Ctrl Pts',(13.7635735385443,-8.27503908348669,4.74058054651189));
#15130=CARTESIAN_POINT('Ctrl Pts',(15.7787256387334,-8.02570849727455,4.62943939898287));
#15131=CARTESIAN_POINT('Ctrl Pts',(17.0810630767753,-9.58356629746378,4.51829825145386));
#15132=CARTESIAN_POINT('Ctrl Pts',(16.4784776508547,-11.5226110448986,4.40715710392483));
#15133=CARTESIAN_POINT('Ctrl Pts',(14.5225522361549,-12.0679178395023,4.29601595639582));
#15134=CARTESIAN_POINT('Ctrl Pts',(13.0036636281943,-10.720334400632,4.18487480886679));
#15135=CARTESIAN_POINT('Ctrl Pts',(13.3121424082065,-8.71338533042983,4.07373366133778));
#15136=CARTESIAN_POINT('Ctrl Pts',(15.1656192969272,-7.88415246139632,3.96259251380876));
#15137=CARTESIAN_POINT('Ctrl Pts',(16.8674948291339,-8.99168277745238,3.85145136627974));
#15138=CARTESIAN_POINT('Ctrl Pts',(16.8599394276748,-11.022186814388,3.74031021875072));
#15139=CARTESIAN_POINT('Ctrl Pts',(15.1498690083362,-12.1170214544196,3.62916907122169));
#15140=CARTESIAN_POINT('Ctrl Pts',(13.3026144239599,-11.2740183532331,3.51802792369268));
#15141=CARTESIAN_POINT('Ctrl Pts',(13.009079488374,-9.26482922085231,3.40688677616365));
#15142=CARTESIAN_POINT('Ctrl Pts',(14.5379544764744,-7.92858635411841,3.29574562863464));
#15143=CARTESIAN_POINT('Ctrl Pts',(16.4897676694624,-8.48843364382804,3.18460448110562));
#15144=CARTESIAN_POINT('Ctrl Pts',(17.077906437004,-10.4319090149314,3.0734633335766));
#15145=CARTESIAN_POINT('Ctrl Pts',(15.7640118038174,-11.9800319497248,2.96232218604758));
#15146=CARTESIAN_POINT('Ctrl Pts',(13.7507709712654,-11.7157119197451,2.85118103851856));
#15147=CARTESIAN_POINT('Ctrl Pts',(12.8810250022902,-9.88089703081255,2.74003989098954));
#15148=CARTESIAN_POINT('Ctrl Pts',(13.9509049709074,-8.15510429042321,2.62889874346052));
#15149=CARTESIAN_POINT('Ctrl Pts',(15.981085052169,-8.11805614433055,2.5177575959315));
#15150=CARTESIAN_POINT('Ctrl Pts',(17.1132186649861,-9.80366499721687,2.40661644840248));
#15151=CARTESIAN_POINT('Ctrl Pts',(16.310995459074,-11.6689911538913,2.29547530087346));
#15152=CARTESIAN_POINT('Ctrl Pts',(14.3087388423873,-12.0065887844825,2.18433415334444));
#15153=CARTESIAN_POINT('Ctrl Pts',(12.9392353574969,-10.5074343907968,2.07319300581542));
#15154=CARTESIAN_POINT('Ctrl Pts',(13.4560743568324,-8.54379458480371,1.9620518582864));
#15155=CARTESIAN_POINT('Ctrl Pts',(15.3861618408855,-7.91310770720139,1.85091071075738));
#15156=CARTESIAN_POINT('Ctrl Pts',(16.9627720598485,-9.19267940420098,1.73976956322836));
#15157=CARTESIAN_POINT('Ctrl Pts',(16.74273830238,-11.2112406954153,1.62862841569934));
#15158=CARTESIAN_POINT('Ctrl Pts',(14.9274708667381,-12.1210796783654,1.51748726817032));
#15159=CARTESIAN_POINT('Ctrl Pts',(13.1785936095798,-11.0893670799319,1.4063461206413));
#15160=CARTESIAN_POINT('Ctrl Pts',(13.0969599890878,-9.06048918569476,1.29520497311228));
#15161=CARTESIAN_POINT('Ctrl Pts',(14.7572934956928,-7.89160571899742,1.18406382558326));
#15162=CARTESIAN_POINT('Ctrl Pts',(16.6397918336695,-8.65265648303387,1.07292267805424));
#15163=CARTESIAN_POINT('Ctrl Pts',(17.0212878267906,-10.6470249052772,0.961781530525217));
#15164=CARTESIAN_POINT('Ctrl Pts',(15.5525802114646,-12.0491077487348,0.850640382996201));
#15165=CARTESIAN_POINT('Ctrl Pts',(13.5780560141864,-11.5755659805163,0.739499235467179));
#15166=CARTESIAN_POINT('Ctrl Pts',(12.9051357290994,-9.65972112260545,0.628358087938161));
#15167=CARTESIAN_POINT('Ctrl Pts',(14.1497469421876,-8.0555329745779,0.51721694040914));
#15168=CARTESIAN_POINT('Ctrl Pts',(16.172693546034,-8.23088631261769,0.406075792880121));
#15169=CARTESIAN_POINT('Ctrl Pts',(17.1221110794925,-10.0262887226278,0.2949346453511));
#15170=CARTESIAN_POINT('Ctrl Pts',(16.1292095662587,-11.796322103078,0.18379349782208));
#15171=CARTESIAN_POINT('Ctrl Pts',(14.1023334213085,-11.9246246253225,0.0726523502930598));
#15172=CARTESIAN_POINT('Ctrl Pts',(12.8977737946205,-10.2860468843054,-0.0384887972359588));
#15173=CARTESIAN_POINT('Ctrl Pts',(13.3769873593213,-9.02713415977151,-0.112582895588639));
#15174=CARTESIAN_POINT('Ctrl Pts',(13.829887250996,-8.638032430062,-0.149629944764979));
#15175=CARTESIAN_POINT('Ctrl Pts',(16.4664903694653,-8.75273391342904,8.14962994476498));
#15176=CARTESIAN_POINT('Ctrl Pts',(16.8812481713146,-9.24039114120218,8.11258289558864));
#15177=CARTESIAN_POINT('Ctrl Pts',(17.1787670194302,-10.6536631383124,8.03848879723595));
#15178=CARTESIAN_POINT('Ctrl Pts',(15.6296475791921,-12.1881429654964,7.92734764970695));
#15179=CARTESIAN_POINT('Ctrl Pts',(13.5043684834796,-11.7141187811832,7.81620650217791));
#15180=CARTESIAN_POINT('Ctrl Pts',(12.7480666941885,-9.67381708082673,7.7050653546489));
#15181=CARTESIAN_POINT('Ctrl Pts',(14.0531253623034,-7.93067817906678,7.59392420711987));
#15182=CARTESIAN_POINT('Ctrl Pts',(16.2249006585358,-8.08244205601081,7.48278305959086));
#15183=CARTESIAN_POINT('Ctrl Pts',(17.2754580108298,-9.98908751297668,7.37164191206184));
#15184=CARTESIAN_POINT('Ctrl Pts',(16.2431470977599,-11.9059153573749,7.26050076453283));
#15185=CARTESIAN_POINT('Ctrl Pts',(14.0729105250557,-12.0780437954813,7.1493596170038));
#15186=CARTESIAN_POINT('Ctrl Pts',(12.7512939495927,-10.3480646077196,7.03821846947479));
#15187=CARTESIAN_POINT('Ctrl Pts',(13.4880545324674,-8.2994542664301,6.92707732194575));
#15188=CARTESIAN_POINT('Ctrl Pts',(15.6087899395717,-7.80746996601717,6.81593617441675));
#15189=CARTESIAN_POINT('Ctrl Pts',(17.1722632498397,-9.32243390287767,6.70479502688772));
#15190=CARTESIAN_POINT('Ctrl Pts',(16.7473325886698,-11.4576187055596,6.5936538793587));
#15191=CARTESIAN_POINT('Ctrl Pts',(14.7229627965935,-12.2585550909766,6.48251273182968));
#15192=CARTESIAN_POINT('Ctrl Pts',(12.9521818877368,-10.9921004110175,6.37137158430066));
#15193=CARTESIAN_POINT('Ctrl Pts',(13.0558927269556,-8.81751573731931,6.26023043677165));
#15194=CARTESIAN_POINT('Ctrl Pts',(14.9391624967676,-7.72533066566421,6.14908928924262));
#15195=CARTESIAN_POINT('Ctrl Pts',(16.8781205145093,-8.71528783842296,6.0379481417136));
#15196=CARTESIAN_POINT('Ctrl Pts',(17.0979212648787,-10.8812198005416,5.92680699418458));
#15197=CARTESIAN_POINT('Ctrl Pts',(15.3973678331242,-12.2405179614955,5.81566584665556));
#15198=CARTESIAN_POINT('Ctrl Pts',(13.3330795968126,-11.5489345795005,5.70452469912655));
#15199=CARTESIAN_POINT('Ctrl Pts',(12.7946243947216,-9.43951771237056,5.59338355159752));
#15200=CARTESIAN_POINT('Ctrl Pts',(14.2748828302889,-7.8431441770876,5.48224240406851));
#15201=CARTESIAN_POINT('Ctrl Pts',(16.4188848549655,-8.2210711865398,5.37110125653948));
#15202=CARTESIAN_POINT('Ctrl Pts',(17.2640957801442,-10.2273593017365,5.25996010901047));
#15203=CARTESIAN_POINT('Ctrl Pts',(16.0368429410561,-12.025531700289,5.14881896148144));
#15204=CARTESIAN_POINT('Ctrl Pts',(13.8605050661451,-11.9696124617812,5.03767781395242));
#15205=CARTESIAN_POINT('Ctrl Pts',(12.7272158028318,-10.1107878458076,4.9265366664234));
#15206=CARTESIAN_POINT('Ctrl Pts',(13.6743433372372,-8.15055241596089,4.81539551889439));
#15207=CARTESIAN_POINT('Ctrl Pts',(15.8349245698249,-7.88322818508548,4.70425437136536));
#15208=CARTESIAN_POINT('Ctrl Pts',(17.2312488606147,-9.55351318531619,4.59311322383635));
#15209=CARTESIAN_POINT('Ctrl Pts',(16.585176158632,-11.6324945634774,4.48197207630732));
#15210=CARTESIAN_POINT('Ctrl Pts',(14.488095872263,-12.2171549602349,4.37083092877831));
#15211=CARTESIAN_POINT('Ctrl Pts',(12.8595923858795,-10.7723193634102,4.25968978124928));
#15212=CARTESIAN_POINT('Ctrl Pts',(13.1903334067103,-8.62053315559428,4.14854863372026));
#15213=CARTESIAN_POINT('Ctrl Pts',(15.1775716804015,-7.7314563588053,4.03740748619125));
#15214=CARTESIAN_POINT('Ctrl Pts',(17.0022678582936,-8.91891472245348,3.92626633866222));
#15215=CARTESIAN_POINT('Ctrl Pts',(16.9941671999881,-11.0959558075831,3.81512519113321));
#15216=CARTESIAN_POINT('Ctrl Pts',(15.1606847278314,-12.269802275955,3.70398404360418));
#15217=CARTESIAN_POINT('Ctrl Pts',(13.1801178086194,-11.3659614793888,3.59284289607517));
#15218=CARTESIAN_POINT('Ctrl Pts',(12.8653990968773,-9.21177354899199,3.48170174854614));
#15219=CARTESIAN_POINT('Ctrl Pts',(14.5046096586769,-7.77909694866307,3.37056060101713));
#15220=CARTESIAN_POINT('Ctrl Pts',(16.5972809532612,-8.37934719634824,3.25941945348811));
#15221=CARTESIAN_POINT('Ctrl Pts',(17.2278644130351,-10.4630789466257,3.14827830595909));
#15222=CARTESIAN_POINT('Ctrl Pts',(15.8191488695313,-12.122926537455,3.03713715843007));
#15223=CARTESIAN_POINT('Ctrl Pts',(13.6606168365978,-11.8395311073445,2.92599601090104));
#15224=CARTESIAN_POINT('Ctrl Pts',(12.7281031977959,-9.87230162926771,2.81485486337203));
#15225=CARTESIAN_POINT('Ctrl Pts',(13.8751940705389,-8.02196219043751,2.70371371584301));
#15226=CARTESIAN_POINT('Ctrl Pts',(16.05188782082,-7.98224036043646,2.59257256831398));
#15227=CARTESIAN_POINT('Ctrl Pts',(17.2657250475012,-9.78949592823614,2.48143142078497));
#15228=CARTESIAN_POINT('Ctrl Pts',(16.4056071423181,-11.7894386057083,2.37029027325595));
#15229=CARTESIAN_POINT('Ctrl Pts',(14.2588520321544,-12.1513999210617,2.25914912572693));
#15230=CARTESIAN_POINT('Ctrl Pts',(12.790514467392,-10.5440548241605,2.14800797819791));
#15231=CARTESIAN_POINT('Ctrl Pts',(13.3446526101798,-8.43870341570221,2.03686683066888));
#15232=CARTESIAN_POINT('Ctrl Pts',(15.414030298795,-7.76250124155411,1.92572568313987));
#15233=CARTESIAN_POINT('Ctrl Pts',(17.1044210389669,-9.13441683741825,1.81458453561085));
#15234=CARTESIAN_POINT('Ctrl Pts',(16.8685079250746,-11.2986532949127,1.70344338808183));
#15235=CARTESIAN_POINT('Ctrl Pts',(14.9222365973632,-12.2741533730727,1.59230224055281));
#15236=CARTESIAN_POINT('Ctrl Pts',(13.0471466825318,-11.1679843263836,1.48116109302379));
#15237=CARTESIAN_POINT('Ctrl Pts',(12.9596217416766,-8.99268673912471,1.37001994549477));
#15238=CARTESIAN_POINT('Ctrl Pts',(14.7397778965747,-7.73944750175331,1.25887879796575));
#15239=CARTESIAN_POINT('Ctrl Pts',(16.7581320342244,-8.55542163972007,1.14773765043673));
#15240=CARTESIAN_POINT('Ctrl Pts',(17.1671597611972,-10.6937192816501,1.03659650290771));
#15241=CARTESIAN_POINT('Ctrl Pts',(15.5924587202513,-12.196987386238,0.925455355378689));
#15242=CARTESIAN_POINT('Ctrl Pts',(13.4754374177256,-11.6892711413137,0.814314207849668));
#15243=CARTESIAN_POINT('Ctrl Pts',(12.7539539431779,-9.63516393810883,0.70317306032065));
#15244=CARTESIAN_POINT('Ctrl Pts',(14.0883860332491,-7.91520502987416,0.592031912791629));
#15245=CARTESIAN_POINT('Ctrl Pts',(16.2573242818248,-8.10321323590726,0.48089076526261));
#15246=CARTESIAN_POINT('Ctrl Pts',(17.2752592081698,-10.028185922409,0.369749617733589));
#15247=CARTESIAN_POINT('Ctrl Pts',(16.2107021580595,-11.9259587518127,0.25860847020457));
#15248=CARTESIAN_POINT('Ctrl Pts',(14.0375507819682,-12.0635205872837,0.147467322675549));
#15249=CARTESIAN_POINT('Ctrl Pts',(12.7460607139427,-10.3066902641307,0.0363261751465303));
#15250=CARTESIAN_POINT('Ctrl Pts',(13.2598580765323,-8.9569245537217,-0.0377679232061503));
#15251=CARTESIAN_POINT('Ctrl Pts',(13.7454427656987,-8.53974220073757,-0.0748149723824902));
#15252=CARTESIAN_POINT('Ctrl Pts',(16.5652001142717,-8.66878019666782,8.22444491714747));
#15253=CARTESIAN_POINT('Ctrl Pts',(17.0078753423991,-9.18926172489923,8.18739786797113));
#15254=CARTESIAN_POINT('Ctrl Pts',(17.3254202405892,-10.6976613280828,8.11330376961845));
#15255=CARTESIAN_POINT('Ctrl Pts',(15.6720292771249,-12.3354272833626,8.00216262208942));
#15256=CARTESIAN_POINT('Ctrl Pts',(13.4036972425399,-11.8294964413313,7.89102147456041));
#15257=CARTESIAN_POINT('Ctrl Pts',(12.5964886364213,-9.65186164669486,7.77988032703138));
#15258=CARTESIAN_POINT('Ctrl Pts',(13.9893910509183,-7.79139173496881,7.66873917950237));
#15259=CARTESIAN_POINT('Ctrl Pts',(16.3073489540956,-7.95337086724347,7.55759803197335));
#15260=CARTESIAN_POINT('Ctrl Pts',(17.4286195209518,-9.9883529914062,7.44645688444433));
#15261=CARTESIAN_POINT('Ctrl Pts',(16.3268235646033,-12.0342028814299,7.33531573691532));
#15262=CARTESIAN_POINT('Ctrl Pts',(14.0105079567266,-12.2179173173397,7.22417458938628));
#15263=CARTESIAN_POINT('Ctrl Pts',(12.5999331189987,-10.3714929024561,7.11303344185728));
#15264=CARTESIAN_POINT('Ctrl Pts',(13.3862851963921,-8.1849902106903,7.00189229432825));
#15265=CARTESIAN_POINT('Ctrl Pts',(15.6497677058271,-7.65989035373928,6.89075114679923));
#15266=CARTESIAN_POINT('Ctrl Pts',(17.3184787010345,-9.27682680041793,6.77960999927021));
#15267=CARTESIAN_POINT('Ctrl Pts',(16.8649458764968,-11.5557312969865,6.66846885174119));
#15268=CARTESIAN_POINT('Ctrl Pts',(14.7043153699076,-12.4105788623587,6.55732770421217));
#15269=CARTESIAN_POINT('Ctrl Pts',(12.8143428623464,-11.0588788777794,6.44618655668315));
#15270=CARTESIAN_POINT('Ctrl Pts',(12.9250344978159,-8.7379224974064,6.33504540915414));
#15271=CARTESIAN_POINT('Ctrl Pts',(14.9350675128906,-7.57222224150645,6.2239042616251));
#15272=CARTESIAN_POINT('Ctrl Pts',(17.0045371624213,-8.62881361925355,6.1127631140961));
#15273=CARTESIAN_POINT('Ctrl Pts',(17.2391327429709,-10.94053487239,6.00162196656707));
#15274=CARTESIAN_POINT('Ctrl Pts',(15.4241147373104,-12.3913276502725,5.89048081903805));
#15275=CARTESIAN_POINT('Ctrl Pts',(13.2208788684359,-11.6531936597153,5.77933967150903));
#15276=CARTESIAN_POINT('Ctrl Pts',(12.6461801446044,-9.40179154332619,5.66819852398002));
#15277=CARTESIAN_POINT('Ctrl Pts',(14.2260750561177,-7.69796580272048,5.55705737645098));
#15278=CARTESIAN_POINT('Ctrl Pts',(16.5143902635653,-8.10133115083163,5.44591622892198));
#15279=CARTESIAN_POINT('Ctrl Pts',(17.4164924963646,-10.2426628994423,5.33477508139295));
#15280=CARTESIAN_POINT('Ctrl Pts',(16.1066330359978,-12.161870623064,5.22363393386394));
#15281=CARTESIAN_POINT('Ctrl Pts',(13.7838054461059,-12.1021874500104,5.1124927863349));
#15282=CARTESIAN_POINT('Ctrl Pts',(12.5742342676142,-10.1182449967136,5.0013516388059));
#15283=CARTESIAN_POINT('Ctrl Pts',(13.5851131359301,-8.02606574843509,4.89021049127687));
#15284=CARTESIAN_POINT('Ctrl Pts',(15.8911235009165,-7.74074787289641,4.77906934374785));
#15285=CARTESIAN_POINT('Ctrl Pts',(17.381434644454,-9.52346007316861,4.66792819621884));
#15286=CARTESIAN_POINT('Ctrl Pts',(16.6918746664094,-11.7423780820561,4.55678704868981));
#15287=CARTESIAN_POINT('Ctrl Pts',(14.453639508371,-12.3663920809676,4.4456459011608));
#15288=CARTESIAN_POINT('Ctrl Pts',(12.7155211435647,-10.8243043261885,4.33450475363177));
#15289=CARTESIAN_POINT('Ctrl Pts',(13.0685244052141,-8.52768098075873,4.22336360610276));
#15290=CARTESIAN_POINT('Ctrl Pts',(15.1895240638759,-7.57876025621427,4.11222245857373));
#15291=CARTESIAN_POINT('Ctrl Pts',(17.1370408874533,-8.84614666745458,4.00108131104471));
#15292=CARTESIAN_POINT('Ctrl Pts',(17.1283949723014,-11.1697248007781,3.8899401635157));
#15293=CARTESIAN_POINT('Ctrl Pts',(15.1715004473266,-12.4225830974903,3.77879901598667));
#15294=CARTESIAN_POINT('Ctrl Pts',(13.0576211932789,-11.4579046055446,3.66765786845765));
#15295=CARTESIAN_POINT('Ctrl Pts',(12.7217187053807,-9.15871787713164,3.55651672092864));
#15296=CARTESIAN_POINT('Ctrl Pts',(14.4712648408794,-7.62960754320777,3.44537557339961));
#15297=CARTESIAN_POINT('Ctrl Pts',(16.7047942370601,-8.27026074886842,3.3342344258706));
#15298=CARTESIAN_POINT('Ctrl Pts',(17.3778223890662,-10.4942488783201,3.22309327834157));
#15299=CARTESIAN_POINT('Ctrl Pts',(15.8742859352451,-12.2658211251852,3.11195213081256));
#15300=CARTESIAN_POINT('Ctrl Pts',(13.5704627019302,-11.9633502949438,3.00081098328354));
#15301=CARTESIAN_POINT('Ctrl Pts',(12.5751813933016,-9.86370622772288,2.88966983575451));
#15302=CARTESIAN_POINT('Ctrl Pts',(13.7994831701705,-7.88882009045181,2.7785286882255));
#15303=CARTESIAN_POINT('Ctrl Pts',(16.122690589471,-7.84642457654237,2.66738754069648));
#15304=CARTESIAN_POINT('Ctrl Pts',(17.4182314300163,-9.77532685925541,2.55624639316745));
#15305=CARTESIAN_POINT('Ctrl Pts',(16.5002188255622,-11.9098860575253,2.44510524563844));
#15306=CARTESIAN_POINT('Ctrl Pts',(14.2089652219215,-12.2962110576408,2.33396409810941));
#15307=CARTESIAN_POINT('Ctrl Pts',(12.641793577287,-10.5806752575243,2.2228229505804));
#15308=CARTESIAN_POINT('Ctrl Pts',(13.2332308635271,-8.3336122466007,2.11168180305138));
#15309=CARTESIAN_POINT('Ctrl Pts',(15.4418987567046,-7.61189477590683,2.00054065552236));
#15310=CARTESIAN_POINT('Ctrl Pts',(17.2460700180853,-9.07615427063553,1.88939950799333));
#15311=CARTESIAN_POINT('Ctrl Pts',(16.9942775477693,-11.3860658944101,1.77825836046432));
#15312=CARTESIAN_POINT('Ctrl Pts',(14.9170023279882,-12.42722706778,1.6671172129353));
#15313=CARTESIAN_POINT('Ctrl Pts',(12.9156997554838,-11.2466015728353,1.55597606540628));
#15314=CARTESIAN_POINT('Ctrl Pts',(12.8222834942654,-8.92488429255467,1.44483491787726));
#15315=CARTESIAN_POINT('Ctrl Pts',(14.7222622974566,-7.58728928450919,1.33369377034824));
#15316=CARTESIAN_POINT('Ctrl Pts',(16.8764722347793,-8.45818679640628,1.22255262281922));
#15317=CARTESIAN_POINT('Ctrl Pts',(17.3130316956038,-10.7404136580229,1.1114114752902));
#15318=CARTESIAN_POINT('Ctrl Pts',(15.632337229038,-12.3448670237413,1.00027032776118));
#15319=CARTESIAN_POINT('Ctrl Pts',(13.3728188212649,-11.8029763021112,0.889129180232157));
#15320=CARTESIAN_POINT('Ctrl Pts',(12.6027721572564,-9.61060675361223,0.777988032703139));
#15321=CARTESIAN_POINT('Ctrl Pts',(14.0270251243106,-7.77487708517042,0.666846885174118));
#15322=CARTESIAN_POINT('Ctrl Pts',(16.3419550176155,-7.97554015919684,0.555705737645099));
#15323=CARTESIAN_POINT('Ctrl Pts',(17.4284073368472,-10.0300831221902,0.444564590116078));
#15324=CARTESIAN_POINT('Ctrl Pts',(16.2921947498604,-12.0555954005474,0.333423442587058));
#15325=CARTESIAN_POINT('Ctrl Pts',(13.9727681426279,-12.2024165492448,0.222282295058038));
#15326=CARTESIAN_POINT('Ctrl Pts',(12.5943476332648,-10.3273336439559,0.111141147529019));
#15327=CARTESIAN_POINT('Ctrl Pts',(13.1427287937432,-8.88671494767188,0.0370470491763388));
#15328=CARTESIAN_POINT('Ctrl Pts',(13.6609982804014,-8.44145197141313,-1.11022302462516E-15));
#15329=CARTESIAN_POINT('Ctrl Pts',(16.2690708798524,-8.92064134695149,8.));
#15330=CARTESIAN_POINT('Ctrl Pts',(16.3147846752501,-8.9632874663071,8.));
#15331=CARTESIAN_POINT('Ctrl Pts',(16.3577652736967,-9.00858426221366,8.));
#15332=CARTESIAN_POINT('Ctrl Pts',(16.3980010936161,-9.05619464640471,8.));
#15333=CARTESIAN_POINT('Ctrl Pts',(16.4235330189367,-9.08640615386467,8.));
#15334=CARTESIAN_POINT('Ctrl Pts',(16.4479592920189,-9.11755027257088,8.));
#15335=CARTESIAN_POINT('Ctrl Pts',(16.471271602956,-9.14954990813044,8.));
#15336=CARTESIAN_POINT('Ctrl Pts',(16.4873497379374,-9.17161955456194,8.));
#15337=CARTESIAN_POINT('Ctrl Pts',(16.502897912595,-9.19409628253225,8.));
#15338=CARTESIAN_POINT('Ctrl Pts',(16.5179120773105,-9.21695643030215,8.));
#15339=CARTESIAN_POINT('Ctrl Pts',(16.5257307264556,-9.22886088707372,8.));
#15340=CARTESIAN_POINT('Ctrl Pts',(16.5334041086722,-9.24086888444548,8.));
#15341=CARTESIAN_POINT('Ctrl Pts',(16.540924657522,-9.25296543092032,8.));
#15342=CARTESIAN_POINT('Ctrl Pts',(16.5757605428611,-9.30899776505104,8.));
#15343=CARTESIAN_POINT('Ctrl Pts',(16.607361406864,-9.36698896324546,8.));
#15344=CARTESIAN_POINT('Ctrl Pts',(16.6356943238752,-9.4265878438185,8.));
#15345=CARTESIAN_POINT('Ctrl Pts',(16.6561185797454,-9.46955069109315,8.));
#15346=CARTESIAN_POINT('Ctrl Pts',(16.6748440447478,-9.51335002846355,8.));
#15347=CARTESIAN_POINT('Ctrl Pts',(16.6918467496953,-9.55786627237312,8.));
#15348=CARTESIAN_POINT('Ctrl Pts',(16.6965928650873,-9.57029248520593,8.));
#15349=CARTESIAN_POINT('Ctrl Pts',(16.7012046820795,-9.58277460807998,8.));
#15350=CARTESIAN_POINT('Ctrl Pts',(16.7056815276087,-9.5953101474753,8.));
#15351=CARTESIAN_POINT('Ctrl Pts',(16.7100593754041,-9.60756848499157,8.));
#15352=CARTESIAN_POINT('Ctrl Pts',(16.7143051500548,-9.61986955747689,8.));
#15353=CARTESIAN_POINT('Ctrl Pts',(16.7184177206078,-9.63220775031721,8.));
#15354=CARTESIAN_POINT('Ctrl Pts',(16.7398746574473,-9.69658107135324,8.));
#15355=CARTESIAN_POINT('Ctrl Pts',(16.757717816168,-9.7619877167845,8.));
#15356=CARTESIAN_POINT('Ctrl Pts',(16.7719146523459,-9.8280714884005,8.));
#15357=CARTESIAN_POINT('Ctrl Pts',(16.7863151656955,-9.89510334137312,8.));
#15358=CARTESIAN_POINT('Ctrl Pts',(16.796964530901,-9.96283279931455,8.));
#15359=CARTESIAN_POINT('Ctrl Pts',(16.8037864817646,-10.0309197852966,8.));
#15360=CARTESIAN_POINT('Ctrl Pts',(16.8080119470385,-10.0730923544962,8.));
#15361=CARTESIAN_POINT('Ctrl Pts',(16.8107681716415,-10.1154026616984,8.));
#15362=CARTESIAN_POINT('Ctrl Pts',(16.8120276488193,-10.1577734446421,8.));
#15363=CARTESIAN_POINT('Ctrl Pts',(16.8130607162965,-10.1925274510017,8.));
#15364=CARTESIAN_POINT('Ctrl Pts',(16.813086670923,-10.2273222138279,8.));
#15365=CARTESIAN_POINT('Ctrl Pts',(16.8120863526574,-10.2621156498343,8.));
#15366=CARTESIAN_POINT('Ctrl Pts',(16.8116796422333,-10.2762620006526,8.));
#15367=CARTESIAN_POINT('Ctrl Pts',(16.8111029763007,-10.2904105498162,8.));
#15368=CARTESIAN_POINT('Ctrl Pts',(16.8103565468589,-10.304534652261,8.));
#15369=CARTESIAN_POINT('Ctrl Pts',(16.8066369705131,-10.3749172958421,8.));
#15370=CARTESIAN_POINT('Ctrl Pts',(16.7987037157801,-10.4448165407578,8.));
#15371=CARTESIAN_POINT('Ctrl Pts',(16.7864939545926,-10.5138749520222,8.));
#15372=CARTESIAN_POINT('Ctrl Pts',(16.7851389335045,-10.521538951517,8.));
#15373=CARTESIAN_POINT('Ctrl Pts',(16.7837311928168,-10.5291926144958,8.));
#15374=CARTESIAN_POINT('Ctrl Pts',(16.7822706091278,-10.5368354652215,8.));
#15375=CARTESIAN_POINT('Ctrl Pts',(16.7696155618455,-10.6030560029649,8.));
#15376=CARTESIAN_POINT('Ctrl Pts',(16.7529979131475,-10.6684646869657,8.));
#15377=CARTESIAN_POINT('Ctrl Pts',(16.7326887106986,-10.7328539224424,8.));
#15378=CARTESIAN_POINT('Ctrl Pts',(16.7108366552886,-10.8021346903597,8.));
#15379=CARTESIAN_POINT('Ctrl Pts',(16.6847110764563,-10.8702362184114,8.));
#15380=CARTESIAN_POINT('Ctrl Pts',(16.6545855938628,-10.9368941313461,8.));
#15381=CARTESIAN_POINT('Ctrl Pts',(16.6490331062011,-10.949179983962,8.));
#15382=CARTESIAN_POINT('Ctrl Pts',(16.6433445705813,-10.9614167555639,8.));
#15383=CARTESIAN_POINT('Ctrl Pts',(16.6375214788432,-10.9736027264117,8.));
#15384=CARTESIAN_POINT('Ctrl Pts',(16.6325870746563,-10.9839289428405,8.));
#15385=CARTESIAN_POINT('Ctrl Pts',(16.6275601738243,-10.9942100372499,8.));
#15386=CARTESIAN_POINT('Ctrl Pts',(16.6224425866455,-11.004444258572,8.));
#15387=CARTESIAN_POINT('Ctrl Pts',(16.5906566971579,-11.068010118141,8.));
#15388=CARTESIAN_POINT('Ctrl Pts',(16.5553718494201,-11.129778140702,8.));
#15389=CARTESIAN_POINT('Ctrl Pts',(16.5168961339094,-11.1895239538667,8.));
#15390=CARTESIAN_POINT('Ctrl Pts',(16.4776077060262,-11.2505317620566,8.));
#15391=CARTESIAN_POINT('Ctrl Pts',(16.4349918293265,-11.3094318958527,8.));
#15392=CARTESIAN_POINT('Ctrl Pts',(16.389322025044,-11.3659771816407,8.));
#15393=CARTESIAN_POINT('Ctrl Pts',(16.343374309462,-11.4228665585434,8.));
#15394=CARTESIAN_POINT('Ctrl Pts',(16.2943348495141,-11.4773732714099,8.));
#15395=CARTESIAN_POINT('Ctrl Pts',(16.2424345785477,-11.5292236977579,8.));
#15396=CARTESIAN_POINT('Ctrl Pts',(16.2296038331093,-11.5420421206477,8.));
#15397=CARTESIAN_POINT('Ctrl Pts',(16.216598038131,-11.5546980557672,8.));
#15398=CARTESIAN_POINT('Ctrl Pts',(16.2034202977729,-11.567187060214,8.));
#15399=CARTESIAN_POINT('Ctrl Pts',(16.1931258534052,-11.5769434644223,8.));
#15400=CARTESIAN_POINT('Ctrl Pts',(16.1827252138162,-11.5865989818742,8.));
#15401=CARTESIAN_POINT('Ctrl Pts',(16.1722359503905,-11.5961372133929,8.));
#15402=CARTESIAN_POINT('Ctrl Pts',(16.1164872924449,-11.6468312978828,8.));
#15403=CARTESIAN_POINT('Ctrl Pts',(16.0581412184438,-11.6943085897836,8.));
#15404=CARTESIAN_POINT('Ctrl Pts',(15.9974954853088,-11.7383155407977,8.));
#15405=CARTESIAN_POINT('Ctrl Pts',(15.9367829685185,-11.7823709526826,8.));
#15406=CARTESIAN_POINT('Ctrl Pts',(15.8737650860283,-11.8229493073405,8.));
#15407=CARTESIAN_POINT('Ctrl Pts',(15.808695859843,-11.859769768599,8.));
#15408=CARTESIAN_POINT('Ctrl Pts',(15.7451092258783,-11.8957512813619,8.));
#15409=CARTESIAN_POINT('Ctrl Pts',(15.679562930207,-11.9281449345628,8.));
#15410=CARTESIAN_POINT('Ctrl Pts',(15.6122617056636,-11.9566513041652,8.));
#15411=CARTESIAN_POINT('Ctrl Pts',(15.5977557447019,-11.9627955056625,8.));
#15412=CARTESIAN_POINT('Ctrl Pts',(15.5831681568552,-11.9687589532201,8.));
#15413=CARTESIAN_POINT('Ctrl Pts',(15.5685008393369,-11.9745383629168,8.));
#15414=CARTESIAN_POINT('Ctrl Pts',(15.5561465682195,-11.9794063555953,8.));
#15415=CARTESIAN_POINT('Ctrl Pts',(15.5437357303612,-11.9841437770524,8.));
#15416=CARTESIAN_POINT('Ctrl Pts',(15.5312701240486,-11.9887510481705,8.));
#15417=CARTESIAN_POINT('Ctrl Pts',(13.3326899541194,-10.0012996150481,6.87148036339021));
#15418=CARTESIAN_POINT('Ctrl Pts',(13.3319603302336,-10.0863816237079,6.87718308383007));
#15419=CARTESIAN_POINT('Ctrl Pts',(13.3379104914095,-10.1713612111695,6.88288580426994));
#15420=CARTESIAN_POINT('Ctrl Pts',(13.3508952182425,-10.25525186711,6.8885885247098));
#15421=CARTESIAN_POINT('Ctrl Pts',(13.4352489610918,-10.8002375960858,6.92563557388614));
#15422=CARTESIAN_POINT('Ctrl Pts',(13.8164823114028,-11.2992671739251,6.96268262306248));
#15423=CARTESIAN_POINT('Ctrl Pts',(14.3201120702849,-11.5239558890949,6.99972967223882));
#15424=CARTESIAN_POINT('Ctrl Pts',(14.8237418291669,-11.7486446042646,7.03677672141516));
#15425=CARTESIAN_POINT('Ctrl Pts',(15.44976799662,-11.6989924567648,7.0738237705915));
#15426=CARTESIAN_POINT('Ctrl Pts',(15.9116712180986,-11.397702424157,7.11087081976784));
#15427=CARTESIAN_POINT('Ctrl Pts',(16.3735744395772,-11.0964123915492,7.14791786894418));
#15428=CARTESIAN_POINT('Ctrl Pts',(16.6713547150814,-10.5434844738334,7.18496491812052));
#15429=CARTESIAN_POINT('Ctrl Pts',(16.6687230323053,-9.99202516121352,7.22201196729686));
#15430=CARTESIAN_POINT('Ctrl Pts',(16.6660913495291,-9.4405658485936,7.2590590164732));
#15431=CARTESIAN_POINT('Ctrl Pts',(16.3630477084726,-8.89057514106954,7.29610606564954));
#15432=CARTESIAN_POINT('Ctrl Pts',(15.8982908742206,-8.59369089292705,7.33315311482588));
#15433=CARTESIAN_POINT('Ctrl Pts',(15.4335340399686,-8.29680664478456,7.37020016400222));
#15434=CARTESIAN_POINT('Ctrl Pts',(14.8070640125211,-8.25302885602365,7.40724721317856));
#15435=CARTESIAN_POINT('Ctrl Pts',(14.3056004695722,-8.48255277528114,7.4442942623549));
#15436=CARTESIAN_POINT('Ctrl Pts',(13.8041369266233,-8.71207669453864,7.48134131153124));
#15437=CARTESIAN_POINT('Ctrl Pts',(13.4276798681731,-9.21490232181455,7.51838836070758));
#15438=CARTESIAN_POINT('Ctrl Pts',(13.3485326982206,-9.76058772075195,7.55543540988392));
#15439=CARTESIAN_POINT('Ctrl Pts',(13.3371065730611,-9.83936589651917,7.56078372771935));
#15440=CARTESIAN_POINT('Ctrl Pts',(13.3318768062629,-9.91903733051551,7.56613204555478));
#15441=CARTESIAN_POINT('Ctrl Pts',(13.3325429336747,-9.99879337075124,7.57148036339021));
#15442=CARTESIAN_POINT('Ctrl Pts',(14.4698297828114,-11.9851743256717,8.));
#15443=CARTESIAN_POINT('Ctrl Pts',(13.8096927451188,-11.8088749487748,7.96295295082366));
#15444=CARTESIAN_POINT('Ctrl Pts',(12.6905564701468,-10.7488614939858,7.88885885247098));
#15445=CARTESIAN_POINT('Ctrl Pts',(13.1189041392622,-8.4613875493231,7.77771770494197));
#15446=CARTESIAN_POINT('Ctrl Pts',(15.2723376840439,-7.58731246609672,7.66657655741293));
#15447=CARTESIAN_POINT('Ctrl Pts',(17.1748664515305,-8.91924865455582,7.55543540988393));
#15448=CARTESIAN_POINT('Ctrl Pts',(17.0874396573092,-11.2417232863365,7.44429426235489));
#15449=CARTESIAN_POINT('Ctrl Pts',(15.0888244971834,-12.4269237058338,7.33315311482589));
#15450=CARTESIAN_POINT('Ctrl Pts',(13.009124094798,-11.3909493747081,7.22201196729685));
#15451=CARTESIAN_POINT('Ctrl Pts',(12.7516786265559,-9.08158195460343,7.11087081976784));
#15452=CARTESIAN_POINT('Ctrl Pts',(14.5523165742456,-7.61298740370139,6.99972967223882));
#15453=CARTESIAN_POINT('Ctrl Pts',(16.7627158202625,-8.32932372056038,6.88858852470981));
#15454=CARTESIAN_POINT('Ctrl Pts',(17.3596103902574,-10.5749548405481,6.77744737718078));
#15455=CARTESIAN_POINT('Ctrl Pts',(15.7966027972857,-12.2942827529436,6.66630622965177));
#15456=CARTESIAN_POINT('Ctrl Pts',(13.5044206790732,-11.9135212765543,6.55516508212274));
#15457=CARTESIAN_POINT('Ctrl Pts',(12.5812305843409,-9.78119480556567,6.44402393459373));
#15458=CARTESIAN_POINT('Ctrl Pts',(13.8720874984692,-7.84915564699463,6.3328827870647));
#15459=CARTESIAN_POINT('Ctrl Pts',(16.1953903487128,-7.88591350252874,6.22174163953568));
#15460=CARTESIAN_POINT('Ctrl Pts',(17.4244804311674,-9.85782300540329,6.11060049200668));
#15461=CARTESIAN_POINT('Ctrl Pts',(16.4342968275999,-11.959875475957,5.99945934447763));
#15462=CARTESIAN_POINT('Ctrl Pts',(14.1312146931719,-12.2679355408755,5.88831819694863));
#15463=CARTESIAN_POINT('Ctrl Pts',(12.62338423969,-10.500017014522,5.7771770494196));
#15464=CARTESIAN_POINT('Ctrl Pts',(13.2910139128176,-8.27440271356362,5.66603590189059));
#15465=CARTESIAN_POINT('Ctrl Pts',(15.522981873134,-7.62833192925066,5.55489475436156));
#15466=CARTESIAN_POINT('Ctrl Pts',(17.2762329089047,-9.15319233958071,5.44375360683254));
#15467=CARTESIAN_POINT('Ctrl Pts',(16.9459103296842,-11.4531869986434,5.33261245930353));
#15468=CARTESIAN_POINT('Ctrl Pts',(14.8343783693084,-12.4229917343393,5.2214713117745));
#15469=CARTESIAN_POINT('Ctrl Pts',(12.8744499009111,-11.1748856301964,5.11033016424549));
#15470=CARTESIAN_POINT('Ctrl Pts',(12.86016595827,-8.85133567083148,4.99918901671646));
#15471=CARTESIAN_POINT('Ctrl Pts',(14.8046014971482,-7.57922762469993,4.88804786918745));
#15472=CARTESIAN_POINT('Ctrl Pts',(16.9278971004046,-8.52299890387884,4.77690672165843));
#15473=CARTESIAN_POINT('Ctrl Pts',(17.2864719188719,-10.8187585919275,4.6657655741294));
#15474=CARTESIAN_POINT('Ctrl Pts',(15.5521007403545,-12.3650590352537,4.55462442660039));
#15475=CARTESIAN_POINT('Ctrl Pts',(13.3123583718527,-11.7464779422144,4.44348327907137));
#15476=CARTESIAN_POINT('Ctrl Pts',(12.6174164274835,-9.52923998930584,4.33234213154235));
#15477=CARTESIAN_POINT('Ctrl Pts',(14.1033972880174,-7.74291713830186,4.22120098401333));
#15478=CARTESIAN_POINT('Ctrl Pts',(16.4100928231865,-8.02263870329727,4.1100598364843));
#15479=CARTESIAN_POINT('Ctrl Pts',(17.4260451371735,-10.1123586227095,3.99891868895528));
#15480=CARTESIAN_POINT('Ctrl Pts',(16.2212916482552,-12.0992299010838,3.88777754142627));
#15481=CARTESIAN_POINT('Ctrl Pts',(13.8986160692799,-12.1645491227624,3.77663639389725));
#15482=CARTESIAN_POINT('Ctrl Pts',(12.584103796379,-10.2485256546711,3.66549524636823));
#15483=CARTESIAN_POINT('Ctrl Pts',(13.4810073938554,-8.10501162795545,3.5543540988392));
#15484=CARTESIAN_POINT('Ctrl Pts',(15.7683367683932,-7.69609503710994,3.44321295131019));
#15485=CARTESIAN_POINT('Ctrl Pts',(17.3523610419581,-9.39608196253575,3.33207180378117));
#15486=CARTESIAN_POINT('Ctrl Pts',(16.7831270202232,-11.6488715830789,3.22093065625215));
#15487=CARTESIAN_POINT('Ctrl Pts',(14.5816890215374,-12.3923493459239,3.10978950872313));
#15488=CARTESIAN_POINT('Ctrl Pts',(12.7631563542956,-10.9459651010282,2.9986483611941));
#15489=CARTESIAN_POINT('Ctrl Pts',(12.9921419248582,-8.63368180206047,2.88750721366509));
#15490=CARTESIAN_POINT('Ctrl Pts',(15.0590413951949,-7.57207216315973,2.77636606613607));
#15491=CARTESIAN_POINT('Ctrl Pts',(17.0718967064505,-8.73289167567321,2.66522491860705));
#15492=CARTESIAN_POINT('Ctrl Pts',(17.1882196870663,-11.053572052764,2.55408377107803));
#15493=CARTESIAN_POINT('Ctrl Pts',(15.3015328785473,-12.4098542253325,2.44294262354901));
#15494=CARTESIAN_POINT('Ctrl Pts',(13.1388347955833,-11.5602511179916,2.33180147601999));
#15495=CARTESIAN_POINT('Ctrl Pts',(12.6797737556826,-9.2824558183502,2.22066032849097));
#15496=CARTESIAN_POINT('Ctrl Pts',(14.3445560924207,-7.66147210297657,2.10951918096195));
#15497=CARTESIAN_POINT('Ctrl Pts',(16.6093058597035,-8.18108435135386,1.99837803343293));
#15498=CARTESIAN_POINT('Ctrl Pts',(17.4009606855609,-10.3656601062701,1.88723688590391));
#15499=CARTESIAN_POINT('Ctrl Pts',(15.9948709901991,-12.2155249905566,1.77609573837489));
#15500=CARTESIAN_POINT('Ctrl Pts',(13.6781157885129,-12.0373860189781,1.66495459084587));
#15501=CARTESIAN_POINT('Ctrl Pts',(12.5713610061794,-9.99430418750461,1.55381344331685));
#15502=CARTESIAN_POINT('Ctrl Pts',(13.6876865848533,-7.95643655777695,1.44267229578783));
#15503=CARTESIAN_POINT('Ctrl Pts',(16.0052515070878,-7.78916517877589,1.33153114825881));
#15504=CARTESIAN_POINT('Ctrl Pts',(17.4026498601701,-9.64560639052843,1.22039000072979));
#15505=CARTESIAN_POINT('Ctrl Pts',(16.6007557452642,-11.8264420086883,1.10924885320077));
#15506=CARTESIAN_POINT('Ctrl Pts',(14.3335965506935,-12.3354315886432,0.998107705671752));
#15507=CARTESIAN_POINT('Ctrl Pts',(12.6764300571871,-10.7066463150279,0.88696655814273));
#15508=CARTESIAN_POINT('Ctrl Pts',(13.1461805475805,-8.43105034420652,0.775825410613713));
#15509=CARTESIAN_POINT('Ctrl Pts',(15.3128190350351,-7.59155964248331,0.664684263084691));
#15510=CARTESIAN_POINT('Ctrl Pts',(17.1931638558005,-8.95675538126231,0.553543115555674));
#15511=CARTESIAN_POINT('Ctrl Pts',(17.0658792003075,-11.2767112418142,0.442401968026652));
#15512=CARTESIAN_POINT('Ctrl Pts',(15.0477525273048,-12.4283740936836,0.331260820497633));
#15513=CARTESIAN_POINT('Ctrl Pts',(12.9855620345442,-11.3565055237641,0.220119672968612));
#15514=CARTESIAN_POINT('Ctrl Pts',(12.7679941505457,-9.04429144693358,0.108978525439592));
#15515=CARTESIAN_POINT('Ctrl Pts',(14.5921706189672,-7.6042694002394,-0.00216262208942743));
#15516=CARTESIAN_POINT('Ctrl Pts',(16.7924325358215,-8.36246876082203,-0.113303769618448));
#15517=CARTESIAN_POINT('Ctrl Pts',(17.160799328377,-9.85926548464068,-0.187397867971127));
#15518=CARTESIAN_POINT('Ctrl Pts',(16.9877912008532,-10.5202727210901,-0.224444917147467));
#15519=CARTESIAN_POINT('Ctrl Pts',(14.5032651029123,-11.8599788000028,8.07481497238249));
#15520=CARTESIAN_POINT('Ctrl Pts',(13.8847597760366,-11.6947977883195,8.03776792320615));
#15521=CARTESIAN_POINT('Ctrl Pts',(12.8362021159643,-10.7016343526812,7.96367382485347));
#15522=CARTESIAN_POINT('Ctrl Pts',(13.2375359299686,-8.55842053633704,7.85253267732444));
#15523=CARTESIAN_POINT('Ctrl Pts',(15.2551626384711,-7.73946922138811,7.74139152979544));
#15524=CARTESIAN_POINT('Ctrl Pts',(17.0377079435153,-8.98740651407504,7.6302503822664));
#15525=CARTESIAN_POINT('Ctrl Pts',(16.9557947423919,-11.1634136902684,7.51910923473739));
#15526=CARTESIAN_POINT('Ctrl Pts',(15.0832227575914,-12.2738691427251,7.40796808720837));
#15527=CARTESIAN_POINT('Ctrl Pts',(13.1346791920357,-11.303228797279,7.29682693967935));
#15528=CARTESIAN_POINT('Ctrl Pts',(12.8934695879748,-9.13950222311102,7.18568579215032));
#15529=CARTESIAN_POINT('Ctrl Pts',(14.5805498437857,-7.76352496249786,7.07454464462133));
#15530=CARTESIAN_POINT('Ctrl Pts',(16.6515496970314,-8.43468534665149,6.96340349709228));
#15531=CARTESIAN_POINT('Ctrl Pts',(17.2108009585808,-10.5386951667414,6.85226234956328));
#15532=CARTESIAN_POINT('Ctrl Pts',(15.7463648385,-12.1495932253925,6.74112120203425));
#15533=CARTESIAN_POINT('Ctrl Pts',(13.598739770773,-11.7928445687211,6.62998005450523));
#15534=CARTESIAN_POINT('Ctrl Pts',(12.7337708950579,-9.79499381101423,6.51883890697621));
#15535=CARTESIAN_POINT('Ctrl Pts',(13.9432195883374,-7.98479919523341,6.40769775944719));
#15536=CARTESIAN_POINT('Ctrl Pts',(16.1200027511848,-8.01923890722387,6.29655661191817));
#15537=CARTESIAN_POINT('Ctrl Pts',(17.2715799537993,-9.8667894338657,6.18541546438915));
#15538=CARTESIAN_POINT('Ctrl Pts',(16.3438425319874,-11.8362754287041,6.07427431686013));
#15539=CARTESIAN_POINT('Ctrl Pts',(14.1860048603503,-12.12490760698,5.9631331693311));
#15540=CARTESIAN_POINT('Ctrl Pts',(12.7732661193704,-10.4684833138455,5.8519920218021));
#15541=CARTESIAN_POINT('Ctrl Pts',(13.3987915567146,-8.38322794698246,5.74085087427306));
#15542=CARTESIAN_POINT('Ctrl Pts',(15.4899998877861,-7.77790178162586,5.62970972674406));
#15543=CARTESIAN_POINT('Ctrl Pts',(17.1326816993761,-9.20659648087737,5.51856857921503));
#15544=CARTESIAN_POINT('Ctrl Pts',(16.8231909979464,-11.3615413895713,5.40742743168601));
#15545=CARTESIAN_POINT('Ctrl Pts',(14.8448233397317,-12.2701851420167,5.29628628415699));
#15546=CARTESIAN_POINT('Ctrl Pts',(13.008498260569,-11.1007911679765,5.18514513662798));
#15547=CARTESIAN_POINT('Ctrl Pts',(12.9951151384173,-8.92377648000767,5.07400398909895));
#15548=CARTESIAN_POINT('Ctrl Pts',(14.8169243536164,-7.73189425257807,4.96286284156993));
#15549=CARTESIAN_POINT('Ctrl Pts',(16.8063137775701,-8.61614635508818,4.85172169404091));
#15550=CARTESIAN_POINT('Ctrl Pts',(17.1422749835657,-10.7671233722962,4.74058054651189));
#15551=CARTESIAN_POINT('Ctrl Pts',(15.5172823662112,-12.2159059833894,4.62943939898287));
#15552=CARTESIAN_POINT('Ctrl Pts',(13.4187899219914,-11.636335864908,4.51829825145386));
#15553=CARTESIAN_POINT('Ctrl Pts',(12.7676746687644,-9.55892858956661,4.40715710392483));
#15554=CARTESIAN_POINT('Ctrl Pts',(14.1599417669537,-7.88526064521431,4.29601595639582));
#15555=CARTESIAN_POINT('Ctrl Pts',(16.3211649592917,-8.14734149829962,4.18487480886679));
#15556=CARTESIAN_POINT('Ctrl Pts',(17.2730459812216,-10.1052726974829,4.07373366133778));
#15557=CARTESIAN_POINT('Ctrl Pts',(16.1442705786589,-11.9668414314328,3.96259251380876));
#15558=CARTESIAN_POINT('Ctrl Pts',(13.9680751280571,-12.0280412797201,3.85145136627974));
#15559=CARTESIAN_POINT('Ctrl Pts',(12.7364629072453,-10.23285232081,3.74031021875071));
#15560=CARTESIAN_POINT('Ctrl Pts',(13.5768030503649,-8.22451955343418,3.6291690712217));
#15561=CARTESIAN_POINT('Ctrl Pts',(15.7198814139359,-7.84139139178789,3.51802792369267));
#15562=CARTESIAN_POINT('Ctrl Pts',(17.2040087922828,-9.43416820775037,3.40688677616366));
#15563=CARTESIAN_POINT('Ctrl Pts',(16.6706736594555,-11.5448850757306,3.29574562863463));
#15564=CARTESIAN_POINT('Ctrl Pts',(14.6080699101901,-12.2414752236498,3.18460448110562));
#15565=CARTESIAN_POINT('Ctrl Pts',(12.9042234698843,-10.8863075704243,3.0734633335766));
#15566=CARTESIAN_POINT('Ctrl Pts',(13.1187680069787,-8.71984900803833,2.96232218604758));
#15567=CARTESIAN_POINT('Ctrl Pts',(15.0553179345335,-7.72519005204671,2.85118103851856));
#15568=CARTESIAN_POINT('Ctrl Pts',(16.9412320116973,-8.81280218564314,2.74003989098954));
#15569=CARTESIAN_POINT('Ctrl Pts',(17.0502190538429,-10.9871282622765,2.62889874346052));
#15570=CARTESIAN_POINT('Ctrl Pts',(15.2825166305796,-12.2578761533695,2.5177575959315));
#15571=CARTESIAN_POINT('Ctrl Pts',(13.2562096543604,-11.461853482899,2.40661644840248));
#15572=CARTESIAN_POINT('Ctrl Pts',(12.8260994161406,-9.32770792535695,2.29547530087346));
#15573=CARTESIAN_POINT('Ctrl Pts',(14.3858918297888,-7.80895196183496,2.18433415334444));
#15574=CARTESIAN_POINT('Ctrl Pts',(16.5078145748011,-8.29579473110992,2.07319300581542));
#15575=CARTESIAN_POINT('Ctrl Pts',(17.2495434869541,-10.3425996583141,1.9620518582864));
#15576=CARTESIAN_POINT('Ctrl Pts',(15.9321291972088,-12.0758023413976,1.85091071075738));
#15577=CARTESIAN_POINT('Ctrl Pts',(13.761480753791,-11.908897749541,1.73976956322836));
#15578=CARTESIAN_POINT('Ctrl Pts',(12.7245237443629,-9.9946633953738,1.62862841569934));
#15579=CARTESIAN_POINT('Ctrl Pts',(13.7704479654167,-8.08531440798811,1.51748726817032));
#15580=CARTESIAN_POINT('Ctrl Pts',(15.9418550641498,-7.92859204120862,1.4063461206413));
#15581=CARTESIAN_POINT('Ctrl Pts',(17.2511261333354,-9.6679563139874,1.29520497311228));
#15582=CARTESIAN_POINT('Ctrl Pts',(16.4998036755118,-11.7112569771147,1.18406382558326));
#15583=CARTESIAN_POINT('Ctrl Pts',(14.3756234543587,-12.1881469992633,1.07292267805424));
#15584=CARTESIAN_POINT('Ctrl Pts',(12.8229665888444,-10.6620814847619,0.961781530525221));
#15585=CARTESIAN_POINT('Ctrl Pts',(13.2630921446325,-8.5299965548063,0.850640382996201));
#15586=CARTESIAN_POINT('Ctrl Pts',(15.2930910227271,-7.74344854851155,0.73949923546718));
#15587=CARTESIAN_POINT('Ctrl Pts',(17.0548514173136,-9.02254786948623,0.628358087938162));
#15588=CARTESIAN_POINT('Ctrl Pts',(16.9355940011155,-11.1961951214013,0.517216940409141));
#15589=CARTESIAN_POINT('Ctrl Pts',(15.0447410019789,-12.2752280614948,0.406075792880122));
#15590=CARTESIAN_POINT('Ctrl Pts',(13.1126030791273,-11.2709571565884,0.294934645351101));
#15591=CARTESIAN_POINT('Ctrl Pts',(12.9087561692788,-9.10456345082775,0.18379349782208));
#15592=CARTESIAN_POINT('Ctrl Pts',(14.617890483002,-7.75535676214991,0.0726523502930618));
#15593=CARTESIAN_POINT('Ctrl Pts',(16.679392320337,-8.46574008648703,-0.0384887972359591));
#15594=CARTESIAN_POINT('Ctrl Pts',(17.0245279670749,-9.86814094278172,-0.112582895588638));
#15595=CARTESIAN_POINT('Ctrl Pts',(16.8624306412829,-10.4874615891075,-0.149629944764978));
#15596=CARTESIAN_POINT('Ctrl Pts',(14.5367004230132,-11.7347832743338,8.14962994476498));
#15597=CARTESIAN_POINT('Ctrl Pts',(13.9598268069544,-11.5807206278643,8.11258289558864));
#15598=CARTESIAN_POINT('Ctrl Pts',(12.9818477617818,-10.6544072113766,8.03848879723596));
#15599=CARTESIAN_POINT('Ctrl Pts',(13.356167720675,-8.65545352335096,7.92734764970694));
#15600=CARTESIAN_POINT('Ctrl Pts',(15.2379875928983,-7.89162597667949,7.81620650217792));
#15601=CARTESIAN_POINT('Ctrl Pts',(16.9005494355002,-9.05556437359427,7.7050653546489));
#15602=CARTESIAN_POINT('Ctrl Pts',(16.8241498274746,-11.0851040942002,7.59392420711988));
#15603=CARTESIAN_POINT('Ctrl Pts',(15.0776210179994,-12.1208145796164,7.48278305959086));
#15604=CARTESIAN_POINT('Ctrl Pts',(13.2602342892733,-11.2155082198498,7.37164191206184));
#15605=CARTESIAN_POINT('Ctrl Pts',(13.0352605493937,-9.19742249161861,7.26050076453282));
#15606=CARTESIAN_POINT('Ctrl Pts',(14.6087831133256,-7.91406252129431,7.1493596170038));
#15607=CARTESIAN_POINT('Ctrl Pts',(16.5403835738004,-8.5400469727426,7.03821846947478));
#15608=CARTESIAN_POINT('Ctrl Pts',(17.0619915269041,-10.5024354929347,6.92707732194576));
#15609=CARTESIAN_POINT('Ctrl Pts',(15.6961268797143,-12.0049036978414,6.81593617441673));
#15610=CARTESIAN_POINT('Ctrl Pts',(13.6930588624727,-11.672167860888,6.70479502688773));
#15611=CARTESIAN_POINT('Ctrl Pts',(12.886311205775,-9.80879281646281,6.59365387935869));
#15612=CARTESIAN_POINT('Ctrl Pts',(14.0143516782056,-8.12044274347216,6.48251273182969));
#15613=CARTESIAN_POINT('Ctrl Pts',(16.0446151536567,-8.152564311919,6.37137158430066));
#15614=CARTESIAN_POINT('Ctrl Pts',(17.1186794764312,-9.87575586232812,6.26023043677165));
#15615=CARTESIAN_POINT('Ctrl Pts',(16.2533882363748,-11.7126753814513,6.14908928924262));
#15616=CARTESIAN_POINT('Ctrl Pts',(14.2407950275287,-11.9818796730845,6.03794814171361));
#15617=CARTESIAN_POINT('Ctrl Pts',(12.9231479990509,-10.4369496131689,5.92680699418458));
#15618=CARTESIAN_POINT('Ctrl Pts',(13.5065692006116,-8.49205318040131,5.81566584665556));
#15619=CARTESIAN_POINT('Ctrl Pts',(15.4570179024382,-7.92747163400105,5.70452469912655));
#15620=CARTESIAN_POINT('Ctrl Pts',(16.9891304898475,-9.26000062217405,5.59338355159752));
#15621=CARTESIAN_POINT('Ctrl Pts',(16.7004716662086,-11.2698957804992,5.48224240406851));
#15622=CARTESIAN_POINT('Ctrl Pts',(14.8552683101549,-12.1173785496942,5.37110125653948));
#15623=CARTESIAN_POINT('Ctrl Pts',(13.1425466202268,-11.0266967057566,5.25996010901047));
#15624=CARTESIAN_POINT('Ctrl Pts',(13.1300643185645,-8.99621728918384,5.14881896148144));
#15625=CARTESIAN_POINT('Ctrl Pts',(14.8292472100845,-7.88456088045623,5.03767781395242));
#15626=CARTESIAN_POINT('Ctrl Pts',(16.6847304547357,-8.70929380629751,4.9265366664234));
#15627=CARTESIAN_POINT('Ctrl Pts',(16.9980780482594,-10.715488152665,4.81539551889438));
#15628=CARTESIAN_POINT('Ctrl Pts',(15.4824639920679,-12.066752931525,4.70425437136536));
#15629=CARTESIAN_POINT('Ctrl Pts',(13.5252214721301,-11.5261937876016,4.59311322383634));
#15630=CARTESIAN_POINT('Ctrl Pts',(12.9179329100453,-9.58861718982735,4.48197207630733));
#15631=CARTESIAN_POINT('Ctrl Pts',(14.21648624589,-8.02760415212678,4.3708309287783));
#15632=CARTESIAN_POINT('Ctrl Pts',(16.2322370953968,-8.27204429330195,4.25968978124928));
#15633=CARTESIAN_POINT('Ctrl Pts',(17.1200468252698,-10.0981867722562,4.14854863372027));
#15634=CARTESIAN_POINT('Ctrl Pts',(16.0672495090626,-11.8344529617818,4.03740748619125));
#15635=CARTESIAN_POINT('Ctrl Pts',(14.0375341868343,-11.8915334366777,3.92626633866222));
#15636=CARTESIAN_POINT('Ctrl Pts',(12.8888220181116,-10.2171789869489,3.81512519113321));
#15637=CARTESIAN_POINT('Ctrl Pts',(13.6725987068744,-8.34402747891293,3.70398404360418));
#15638=CARTESIAN_POINT('Ctrl Pts',(15.6714260594787,-7.98668774646583,3.59284289607517));
#15639=CARTESIAN_POINT('Ctrl Pts',(17.0556565426075,-9.47225445296499,3.48170174854615));
#15640=CARTESIAN_POINT('Ctrl Pts',(16.5582202986879,-11.4408985683823,3.37056060101712));
#15641=CARTESIAN_POINT('Ctrl Pts',(14.6344507988427,-12.0906011013757,3.25941945348811));
#15642=CARTESIAN_POINT('Ctrl Pts',(13.045290585473,-10.8266500398205,3.14827830595908));
#15643=CARTESIAN_POINT('Ctrl Pts',(13.2453940890993,-8.80601621401618,3.03713715843007));
#15644=CARTESIAN_POINT('Ctrl Pts',(15.0515944738721,-7.87830794093373,2.92599601090105));
#15645=CARTESIAN_POINT('Ctrl Pts',(16.810567316944,-8.89271269561304,2.81485486337202));
#15646=CARTESIAN_POINT('Ctrl Pts',(16.9122184206196,-10.9206844717891,2.70371371584301));
#15647=CARTESIAN_POINT('Ctrl Pts',(15.2635003826118,-12.1058980814064,2.59257256831398));
#15648=CARTESIAN_POINT('Ctrl Pts',(13.3735845131376,-11.3634558478065,2.48143142078497));
#15649=CARTESIAN_POINT('Ctrl Pts',(12.9724250765987,-9.3729600323637,2.37029027325594));
#15650=CARTESIAN_POINT('Ctrl Pts',(14.4272275671569,-7.95643182069336,2.25914912572693));
#15651=CARTESIAN_POINT('Ctrl Pts',(16.4063232898986,-8.41050511086595,2.14800797819791));
#15652=CARTESIAN_POINT('Ctrl Pts',(17.0981262883473,-10.3195392103582,2.03686683066889));
#15653=CARTESIAN_POINT('Ctrl Pts',(15.8693874042187,-11.9360796922385,1.92572568313987));
#15654=CARTESIAN_POINT('Ctrl Pts',(13.8448457190691,-11.7804094801039,1.81458453561085));
#15655=CARTESIAN_POINT('Ctrl Pts',(12.8776864825464,-9.99502260324298,1.70344338808183));
#15656=CARTESIAN_POINT('Ctrl Pts',(13.8532093459802,-8.21419225819928,1.59230224055281));
#15657=CARTESIAN_POINT('Ctrl Pts',(15.8784586212119,-8.06801890364133,1.48116109302379));
#15658=CARTESIAN_POINT('Ctrl Pts',(17.0996024065006,-9.69030623744639,1.37001994549477));
#15659=CARTESIAN_POINT('Ctrl Pts',(16.3988516057594,-11.5960719455411,1.25887879796575));
#15660=CARTESIAN_POINT('Ctrl Pts',(14.4176503580238,-12.0408624098834,1.14773765043673));
#15661=CARTESIAN_POINT('Ctrl Pts',(12.9695031205017,-10.6175166544959,1.03659650290771));
#15662=CARTESIAN_POINT('Ctrl Pts',(13.3800037416846,-8.62894276540608,0.92545535537869));
#15663=CARTESIAN_POINT('Ctrl Pts',(15.273363010419,-7.8953374545398,0.81431420784967));
#15664=CARTESIAN_POINT('Ctrl Pts',(16.9165389788268,-9.08834035771014,0.703173060320651));
#15665=CARTESIAN_POINT('Ctrl Pts',(16.8053088019234,-11.1156790009884,0.59203191279163));
#15666=CARTESIAN_POINT('Ctrl Pts',(15.0417294766531,-12.1220820293061,0.480890765262611));
#15667=CARTESIAN_POINT('Ctrl Pts',(13.2396441237103,-11.1854087894126,0.36974961773359));
#15668=CARTESIAN_POINT('Ctrl Pts',(13.0495181880118,-9.16483545472189,0.25860847020457));
#15669=CARTESIAN_POINT('Ctrl Pts',(14.6436103470368,-7.90644412406044,0.14746732267555));
#15670=CARTESIAN_POINT('Ctrl Pts',(16.5663521048524,-8.56901141215202,0.0363261751465301));
#15671=CARTESIAN_POINT('Ctrl Pts',(16.8882566057727,-9.87701640092277,-0.0377679232061492));
#15672=CARTESIAN_POINT('Ctrl Pts',(16.7370700817125,-10.4546504571249,-0.0748149723824891));
#15673=CARTESIAN_POINT('Ctrl Pts',(14.5701357431141,-11.6095877486648,8.22444491714747));
#15674=CARTESIAN_POINT('Ctrl Pts',(14.0348938378722,-11.4666434674091,8.18739786797113));
#15675=CARTESIAN_POINT('Ctrl Pts',(13.1274934075993,-10.6071800700719,8.11330376961845));
#15676=CARTESIAN_POINT('Ctrl Pts',(13.4747995113813,-8.75248651036489,8.00216262208942));
#15677=CARTESIAN_POINT('Ctrl Pts',(15.2208125473255,-8.04378273197088,7.89102147456042));
#15678=CARTESIAN_POINT('Ctrl Pts',(16.763390927485,-9.1237222331135,7.77988032703139));
#15679=CARTESIAN_POINT('Ctrl Pts',(16.6925049125573,-11.006794498132,7.66873917950237));
#15680=CARTESIAN_POINT('Ctrl Pts',(15.0720192784074,-11.9677600165076,7.55759803197335));
#15681=CARTESIAN_POINT('Ctrl Pts',(13.385789386511,-11.1277876424206,7.44645688444433));
#15682=CARTESIAN_POINT('Ctrl Pts',(13.1770515108126,-9.2553427601262,7.33531573691531));
#15683=CARTESIAN_POINT('Ctrl Pts',(14.6370163828657,-8.06460008009077,7.22417458938628));
#15684=CARTESIAN_POINT('Ctrl Pts',(16.4292174505694,-8.64540859883372,7.11303344185728));
#15685=CARTESIAN_POINT('Ctrl Pts',(16.9131820952275,-10.4661758191279,7.00189229432824));
#15686=CARTESIAN_POINT('Ctrl Pts',(15.6458889209286,-11.8602141702903,6.89075114679924));
#15687=CARTESIAN_POINT('Ctrl Pts',(13.7873779541725,-11.5514911530548,6.7796099992702));
#15688=CARTESIAN_POINT('Ctrl Pts',(13.038851516492,-9.82259182191137,6.6684688517412));
#15689=CARTESIAN_POINT('Ctrl Pts',(14.0854837680738,-8.25608629171094,6.55732770421216));
#15690=CARTESIAN_POINT('Ctrl Pts',(15.9692275561287,-8.28588971661412,6.44618655668316));
#15691=CARTESIAN_POINT('Ctrl Pts',(16.9657789990631,-9.88472229079055,6.33504540915413));
#15692=CARTESIAN_POINT('Ctrl Pts',(16.1629339407623,-11.5890753341985,6.22390426162511));
#15693=CARTESIAN_POINT('Ctrl Pts',(14.295585194707,-11.838851739189,6.11276311409609));
#15694=CARTESIAN_POINT('Ctrl Pts',(13.0730298787315,-10.4054159124924,6.00162196656708));
#15695=CARTESIAN_POINT('Ctrl Pts',(13.6143468445086,-8.60087841382016,5.89048081903805));
#15696=CARTESIAN_POINT('Ctrl Pts',(15.4240359170902,-8.07704148637625,5.77933967150903));
#15697=CARTESIAN_POINT('Ctrl Pts',(16.8455792803189,-9.31340476347071,5.66819852398002));
#15698=CARTESIAN_POINT('Ctrl Pts',(16.5777523344708,-11.1782501714271,5.55705737645098));
#15699=CARTESIAN_POINT('Ctrl Pts',(14.8657132805781,-11.9645719573716,5.44591622892198));
#15700=CARTESIAN_POINT('Ctrl Pts',(13.2765949798846,-10.9526022435367,5.33477508139295));
#15701=CARTESIAN_POINT('Ctrl Pts',(13.2650134987117,-9.06865809836003,5.22363393386394));
#15702=CARTESIAN_POINT('Ctrl Pts',(14.8415700665526,-8.03722750833437,5.11249278633491));
#15703=CARTESIAN_POINT('Ctrl Pts',(16.5631471319012,-8.80244125750684,5.00135163880589));
#15704=CARTESIAN_POINT('Ctrl Pts',(16.8538811129532,-10.6638529330338,4.89021049127687));
#15705=CARTESIAN_POINT('Ctrl Pts',(15.4476456179246,-11.9175998796606,4.77906934374785));
#15706=CARTESIAN_POINT('Ctrl Pts',(13.6316530222687,-11.4160517102953,4.66792819621883));
#15707=CARTESIAN_POINT('Ctrl Pts',(13.0681911513262,-9.61830579008811,4.55678704868982));
#15708=CARTESIAN_POINT('Ctrl Pts',(14.2730307248264,-8.16994765903925,4.44564590116079));
#15709=CARTESIAN_POINT('Ctrl Pts',(16.143309231502,-8.39674708830429,4.33450475363177));
#15710=CARTESIAN_POINT('Ctrl Pts',(16.9670476693179,-10.0911008470296,4.22336360610275));
#15711=CARTESIAN_POINT('Ctrl Pts',(15.9902284394662,-11.7020644921307,4.11222245857374));
#15712=CARTESIAN_POINT('Ctrl Pts',(14.1069932456115,-11.7550255936353,4.00108131104471));
#15713=CARTESIAN_POINT('Ctrl Pts',(13.0411811289779,-10.2015056530877,3.88994016351569));
#15714=CARTESIAN_POINT('Ctrl Pts',(13.7683943633839,-8.46353540439168,3.77879901598667));
#15715=CARTESIAN_POINT('Ctrl Pts',(15.6229707050215,-8.13198410114376,3.66765786845766));
#15716=CARTESIAN_POINT('Ctrl Pts',(16.9073042929321,-9.51034069817962,3.55651672092863));
#15717=CARTESIAN_POINT('Ctrl Pts',(16.4457669379203,-11.3369120610339,3.44537557339962));
#15718=CARTESIAN_POINT('Ctrl Pts',(14.6608316874954,-11.9397269791017,3.33423442587059));
#15719=CARTESIAN_POINT('Ctrl Pts',(13.1863577010617,-10.7669925092167,3.22309327834158));
#15720=CARTESIAN_POINT('Ctrl Pts',(13.3720201712198,-8.89218341999404,3.11195213081255));
#15721=CARTESIAN_POINT('Ctrl Pts',(15.0478710132107,-8.03142582982071,3.00081098328354));
#15722=CARTESIAN_POINT('Ctrl Pts',(16.6799026221908,-8.97262320558296,2.88966983575451));
#15723=CARTESIAN_POINT('Ctrl Pts',(16.7742177873962,-10.8542406813017,2.7785286882255));
#15724=CARTESIAN_POINT('Ctrl Pts',(15.2444841346441,-11.9539200094434,2.66738754069648));
#15725=CARTESIAN_POINT('Ctrl Pts',(13.4909593719147,-11.2650582127139,2.55624639316746));
#15726=CARTESIAN_POINT('Ctrl Pts',(13.1187507370567,-9.41821213937045,2.44510524563843));
#15727=CARTESIAN_POINT('Ctrl Pts',(14.4685633045251,-8.10391167955175,2.33396409810942));
#15728=CARTESIAN_POINT('Ctrl Pts',(16.3048320049962,-8.52521549062199,2.2228229505804));
#15729=CARTESIAN_POINT('Ctrl Pts',(16.9467090897406,-10.2964787624023,2.11168180305138));
#15730=CARTESIAN_POINT('Ctrl Pts',(15.8066456112284,-11.7963570430794,2.00054065552236));
#15731=CARTESIAN_POINT('Ctrl Pts',(13.9282106843473,-11.6519212106668,1.88939950799334));
#15732=CARTESIAN_POINT('Ctrl Pts',(13.0308492207299,-9.99538181111215,1.77825836046432));
#15733=CARTESIAN_POINT('Ctrl Pts',(13.9359707265436,-8.34307010841046,1.6671172129353));
#15734=CARTESIAN_POINT('Ctrl Pts',(15.8150621782739,-8.20744576607403,1.55597606540628));
#15735=CARTESIAN_POINT('Ctrl Pts',(16.9480786796658,-9.71265616090539,1.44483491787726));
#15736=CARTESIAN_POINT('Ctrl Pts',(16.2978995360069,-11.4808869139675,1.33369377034824));
#15737=CARTESIAN_POINT('Ctrl Pts',(14.459677261689,-11.8935778205035,1.22255262281922));
#15738=CARTESIAN_POINT('Ctrl Pts',(13.116039652159,-10.5729518242299,1.1114114752902));
#15739=CARTESIAN_POINT('Ctrl Pts',(13.4969153387366,-8.72788897600587,1.00027032776118));
#15740=CARTESIAN_POINT('Ctrl Pts',(15.2536349981109,-8.04722636056805,0.889129180232159));
#15741=CARTESIAN_POINT('Ctrl Pts',(16.77822654034,-9.15413284593406,0.77798803270314));
#15742=CARTESIAN_POINT('Ctrl Pts',(16.6750236027314,-11.0351628805755,0.66684688517412));
#15743=CARTESIAN_POINT('Ctrl Pts',(15.0387179513273,-11.9689359971173,0.5557057376451));
#15744=CARTESIAN_POINT('Ctrl Pts',(13.3666851682933,-11.0998604222368,0.44456459011608));
#15745=CARTESIAN_POINT('Ctrl Pts',(13.1902802067449,-9.22510745861606,0.333423442587058));
#15746=CARTESIAN_POINT('Ctrl Pts',(14.6693302110716,-8.05753148597096,0.22228229505804));
#15747=CARTESIAN_POINT('Ctrl Pts',(16.4533118893679,-8.67228273781702,0.111141147529019));
#15748=CARTESIAN_POINT('Ctrl Pts',(16.7519852444706,-9.88589185906381,0.0370470491763399));
#15749=CARTESIAN_POINT('Ctrl Pts',(16.6117095221421,-10.4218393251423,0.));
#15750=CARTESIAN_POINT('Ctrl Pts',(13.3361815844527,-9.99906045492932,7.3785196366098));
#15751=CARTESIAN_POINT('Ctrl Pts',(13.3350653698557,-9.78304622671375,7.36411833671163));
#15752=CARTESIAN_POINT('Ctrl Pts',(13.3741037210664,-9.56741861718908,7.34971703681347));
#15753=CARTESIAN_POINT('Ctrl Pts',(13.4551686354378,-9.36895979383603,7.33531573691531));
#15754=CARTESIAN_POINT('Ctrl Pts',(13.6637064681636,-8.85842853344772,7.29826868773897));
#15755=CARTESIAN_POINT('Ctrl Pts',(14.1503614255146,-8.46151430676925,7.26122163856262));
#15756=CARTESIAN_POINT('Ctrl Pts',(14.6923890821408,-8.3598586132205,7.22417458938629));
#15757=CARTESIAN_POINT('Ctrl Pts',(15.2344167387669,-8.25820291967176,7.18712754020995));
#15758=CARTESIAN_POINT('Ctrl Pts',(15.8318170946681,-8.45180575925274,7.15008049103361));
#15759=CARTESIAN_POINT('Ctrl Pts',(16.2111780467284,-8.8520683824256,7.11303344185727));
#15760=CARTESIAN_POINT('Ctrl Pts',(16.5905389987887,-9.25233100559846,7.07598639268093));
#15761=CARTESIAN_POINT('Ctrl Pts',(16.7518605470081,-9.8592534123632,7.03893934350459));
#15762=CARTESIAN_POINT('Ctrl Pts',(16.621305792068,-10.3950543409393,7.00189229432825));
#15763=CARTESIAN_POINT('Ctrl Pts',(16.4907510371279,-10.9308552695154,6.96484524515191));
#15764=CARTESIAN_POINT('Ctrl Pts',(16.0683199790282,-11.3955347199029,6.92779819597557));
#15765=CARTESIAN_POINT('Ctrl Pts',(15.5473526221857,-11.5764206088907,6.89075114679923));
#15766=CARTESIAN_POINT('Ctrl Pts',(15.0263852653432,-11.7573064978785,6.85370409762289));
#15767=CARTESIAN_POINT('Ctrl Pts',(14.4068816097579,-11.6543988254667,6.81665704844655));
#15768=CARTESIAN_POINT('Ctrl Pts',(13.9723753756851,-11.3147951007368,6.77960999927021));
#15769=CARTESIAN_POINT('Ctrl Pts',(13.5771626776233,-11.0059026297031,6.74591321171674));
#15770=CARTESIAN_POINT('Ctrl Pts',(13.3350007187014,-10.5011884793045,6.71221642416327));
#15771=CARTESIAN_POINT('Ctrl Pts',(13.331821388128,-9.99913246339926,6.6785196366098));
#15772=CARTESIAN_POINT('Ctrl Pts',(13.1998077676745,-10.0021672449552,7.99999999904539));
#15773=CARTESIAN_POINT('Ctrl Pts',(13.2074798175735,-9.93506922612593,7.99999999936359));
#15774=CARTESIAN_POINT('Ctrl Pts',(13.2188240784654,-9.86823467174956,8.));
#15775=CARTESIAN_POINT('Ctrl Pts',(13.2338166554418,-9.80202407246294,8.));
#15776=CARTESIAN_POINT('Ctrl Pts',(13.2487940185892,-9.73588066087505,8.));
#15777=CARTESIAN_POINT('Ctrl Pts',(13.2673389547068,-9.67068097467151,8.));
#15778=CARTESIAN_POINT('Ctrl Pts',(13.2893701892982,-9.6067646838403,8.));
#15779=CARTESIAN_POINT('Ctrl Pts',(13.3109714057993,-9.54409594730352,8.));
#15780=CARTESIAN_POINT('Ctrl Pts',(13.3359247078376,-9.48266014999381,8.));
#15781=CARTESIAN_POINT('Ctrl Pts',(13.3641933030361,-9.42280701535511,8.));
#15782=CARTESIAN_POINT('Ctrl Pts',(13.3758894405641,-9.39804276763416,8.));
#15783=CARTESIAN_POINT('Ctrl Pts',(13.3881535513658,-9.37354987995325,8.));
#15784=CARTESIAN_POINT('Ctrl Pts',(13.4009847510562,-9.34935515259193,8.));
#15785=CARTESIAN_POINT('Ctrl Pts',(13.4067964172714,-9.33839657638825,8.));
#15786=CARTESIAN_POINT('Ctrl Pts',(13.4127244333369,-9.32749918518064,8.));
#15787=CARTESIAN_POINT('Ctrl Pts',(13.4187687789279,-9.31666556315984,8.));
#15788=CARTESIAN_POINT('Ctrl Pts',(13.425159640313,-9.30521086130789,8.));
#15789=CARTESIAN_POINT('Ctrl Pts',(13.431676443445,-9.2938348748043,8.));
#15790=CARTESIAN_POINT('Ctrl Pts',(13.4383166419856,-9.28254377672475,8.));
#15791=CARTESIAN_POINT('Ctrl Pts',(13.4709216418811,-9.22710172187461,8.));
#15792=CARTESIAN_POINT('Ctrl Pts',(13.5065145504896,-9.17367537459915,8.));
#15793=CARTESIAN_POINT('Ctrl Pts',(13.5450538037118,-9.12258927669459,8.));
#15794=CARTESIAN_POINT('Ctrl Pts',(13.5823769497808,-9.07311520195852,8.));
#15795=CARTESIAN_POINT('Ctrl Pts',(13.6224639480267,-9.02583549550675,8.));
#15796=CARTESIAN_POINT('Ctrl Pts',(13.6653053703033,-8.9810847385994,8.));
#15797=CARTESIAN_POINT('Ctrl Pts',(13.6782878320201,-8.96752368115845,8.));
#15798=CARTESIAN_POINT('Ctrl Pts',(13.6915234071565,-8.9541951706708,8.));
#15799=CARTESIAN_POINT('Ctrl Pts',(13.7050122636503,-8.94110937848357,8.));
#15800=CARTESIAN_POINT('Ctrl Pts',(13.7127736320724,-8.93357992968962,8.));
#15801=CARTESIAN_POINT('Ctrl Pts',(13.7206188601492,-8.92613084760238,8.));
#15802=CARTESIAN_POINT('Ctrl Pts',(13.7285464165792,-8.9187628208919,8.));
#15803=CARTESIAN_POINT('Ctrl Pts',(14.4698297828114,-11.9851743256717,8.));
#15804=CARTESIAN_POINT('Ctrl Pts',(14.3998214683822,-11.9592528423604,8.));
#15805=CARTESIAN_POINT('Ctrl Pts',(14.3314995298914,-11.9292588102101,8.));
#15806=CARTESIAN_POINT('Ctrl Pts',(14.2650832927778,-11.8954790830356,8.));
#15807=CARTESIAN_POINT('Ctrl Pts',(14.200410195712,-11.8625859281483,8.));
#15808=CARTESIAN_POINT('Ctrl Pts',(14.1375436561858,-11.8261022624894,8.));
#15809=CARTESIAN_POINT('Ctrl Pts',(14.0767171136307,-11.7862591514963,8.));
#15810=CARTESIAN_POINT('Ctrl Pts',(14.0631404357672,-11.7773660423319,8.));
#15811=CARTESIAN_POINT('Ctrl Pts',(14.0496637435695,-11.7683042245779,8.));
#15812=CARTESIAN_POINT('Ctrl Pts',(14.0362955933952,-11.7590800518159,8.));
#15813=CARTESIAN_POINT('Ctrl Pts',(13.9749538754163,-11.7167535820521,8.));
#15814=CARTESIAN_POINT('Ctrl Pts',(13.9160153064361,-11.6710962446947,8.));
#15815=CARTESIAN_POINT('Ctrl Pts',(13.8597184805936,-11.6223773773913,8.));
#15816=CARTESIAN_POINT('Ctrl Pts',(13.8201933952585,-11.5881726534344,8.));
#15817=CARTESIAN_POINT('Ctrl Pts',(13.7819712022528,-11.5524579711967,8.));
#15818=CARTESIAN_POINT('Ctrl Pts',(13.7451473327347,-11.5153181422045,8.));
#15819=CARTESIAN_POINT('Ctrl Pts',(13.7311386073503,-11.5011892178959,8.));
#15820=CARTESIAN_POINT('Ctrl Pts',(13.717332371766,-11.4868539850208,8.));
#15821=CARTESIAN_POINT('Ctrl Pts',(13.7037343400326,-11.4723169303692,8.));
#15822=CARTESIAN_POINT('Ctrl Pts',(13.6908095393624,-11.4584995972883,8.));
#15823=CARTESIAN_POINT('Ctrl Pts',(13.6780690151191,-11.4444953919844,8.));
#15824=CARTESIAN_POINT('Ctrl Pts',(13.6655396735727,-11.4303333656545,8.));
#15825=CARTESIAN_POINT('Ctrl Pts',(13.6174405812511,-11.3759665332569,8.));
#15826=CARTESIAN_POINT('Ctrl Pts',(13.5723959249184,-11.3192214581869,8.));
#15827=CARTESIAN_POINT('Ctrl Pts',(13.5306282578393,-11.2603460850308,8.));
#15828=CARTESIAN_POINT('Ctrl Pts',(13.4897585016075,-11.2027363999032,8.));
#15829=CARTESIAN_POINT('Ctrl Pts',(13.4520259976655,-11.1430861593352,8.));
#15830=CARTESIAN_POINT('Ctrl Pts',(13.4176843817239,-11.0816085238734,8.));
#15831=CARTESIAN_POINT('Ctrl Pts',(13.3840955339157,-11.0214784780236,8.));
#15832=CARTESIAN_POINT('Ctrl Pts',(13.3537502688523,-10.9595995550916,8.));
#15833=CARTESIAN_POINT('Ctrl Pts',(13.3269341460252,-10.8961642041122,8.));
#15834=CARTESIAN_POINT('Ctrl Pts',(13.3182225174315,-10.8755562578776,8.));
#15835=CARTESIAN_POINT('Ctrl Pts',(13.3098837493054,-10.8547840384658,8.));
#15836=CARTESIAN_POINT('Ctrl Pts',(13.3019288365863,-10.8338541688359,8.));
#15837=CARTESIAN_POINT('Ctrl Pts',(13.2974344402897,-10.8220291329271,8.));
#15838=CARTESIAN_POINT('Ctrl Pts',(13.2930622312048,-10.8101524909552,8.));
#15839=CARTESIAN_POINT('Ctrl Pts',(13.2888200152093,-10.7982424246399,8.));
#15840=CARTESIAN_POINT('Ctrl Pts',(13.265903681499,-10.7339045751566,8.));
#15841=CARTESIAN_POINT('Ctrl Pts',(13.2467331549497,-10.6684810537996,8.));
#15842=CARTESIAN_POINT('Ctrl Pts',(13.2315367307289,-10.6021713571593,8.));
#15843=CARTESIAN_POINT('Ctrl Pts',(13.2293393441876,-10.5925830465909,8.));
#15844=CARTESIAN_POINT('Ctrl Pts',(13.2272251395615,-10.5829761934059,8.));
#15845=CARTESIAN_POINT('Ctrl Pts',(13.2251948980547,-10.5733513897451,8.));
#15846=CARTESIAN_POINT('Ctrl Pts',(13.2108418424753,-10.5053075922838,8.));
#15847=CARTESIAN_POINT('Ctrl Pts',(13.2006809368273,-10.4363661073907,8.));
#15848=CARTESIAN_POINT('Ctrl Pts',(13.1946148801756,-10.3668853682355,8.));
#15849=CARTESIAN_POINT('Ctrl Pts',(13.1893452075922,-10.3065264287755,8.));
#15850=CARTESIAN_POINT('Ctrl Pts',(13.1871667948597,-10.245760095398,8.));
#15851=CARTESIAN_POINT('Ctrl Pts',(13.188045983141,-10.1848309054691,8.));
#15852=CARTESIAN_POINT('Ctrl Pts',(13.1882953481151,-10.1675495037619,8.));
#15853=CARTESIAN_POINT('Ctrl Pts',(13.1887908474924,-10.1502550857216,8.));
#15854=CARTESIAN_POINT('Ctrl Pts',(13.1895320856308,-10.1329534599018,8.));
#15855=CARTESIAN_POINT('Ctrl Pts',(13.1900857549631,-10.1200299753721,8.));
#15856=CARTESIAN_POINT('Ctrl Pts',(13.1907767641003,-10.1071003962073,8.));
#15857=CARTESIAN_POINT('Ctrl Pts',(13.1916034374083,-10.0941871331301,8.));
#15858=CARTESIAN_POINT('Ctrl Pts',(13.1935720387064,-10.0634360901101,8.));
#15859=CARTESIAN_POINT('Ctrl Pts',(13.1963106067788,-10.0327526423872,8.));
#15860=CARTESIAN_POINT('Ctrl Pts',(13.1998077693062,-10.0021672451286,8.));
#15861=CARTESIAN_POINT('Origin',(0.,0.,8.));
#15862=CARTESIAN_POINT('',(-12.,10.,8.));
#15863=CARTESIAN_POINT('',(-6.,10.,8.));
#15864=CARTESIAN_POINT('',(-16.,6.,8.));
#15865=CARTESIAN_POINT('',(-13.5,8.5,8.));
#15866=CARTESIAN_POINT('',(-16.,-5.,8.));
#15867=CARTESIAN_POINT('',(2.,4.,8.));
#15868=CARTESIAN_POINT('',(-2.,4.,8.));
#15869=CARTESIAN_POINT('',(1.,4.,8.));
#15870=CARTESIAN_POINT('',(-2.,6.,8.));
#15871=CARTESIAN_POINT('',(-2.,2.,8.));
#15872=CARTESIAN_POINT('',(2.,6.,8.));
#15873=CARTESIAN_POINT('',(-1.,6.,8.));
#15874=CARTESIAN_POINT('',(2.,3.,8.));
#15875=CARTESIAN_POINT('',(10.,-6.,8.));
#15876=CARTESIAN_POINT('',(6.,-6.,8.));
#15877=CARTESIAN_POINT('',(5.,-6.,8.));
#15878=CARTESIAN_POINT('',(6.,-4.,8.));
#15879=CARTESIAN_POINT('',(6.,-3.,8.));
#15880=CARTESIAN_POINT('',(10.,-4.,8.));
#15881=CARTESIAN_POINT('',(3.,-4.,8.));
#15882=CARTESIAN_POINT('',(10.,-2.,8.));
#15883=CARTESIAN_POINT('',(-6.,-6.,8.));
#15884=CARTESIAN_POINT('',(-10.,-6.,8.));
#15885=CARTESIAN_POINT('',(-3.,-6.,8.));
#15886=CARTESIAN_POINT('',(-10.,-4.,8.));
#15887=CARTESIAN_POINT('',(-10.,-3.,8.));
#15888=CARTESIAN_POINT('',(-6.,-4.,8.));
#15889=CARTESIAN_POINT('',(-5.,-4.,8.));
#15890=CARTESIAN_POINT('',(-6.,-2.,8.));
#15891=CARTESIAN_POINT('Origin',(15.,-10.,8.));
#15892=CARTESIAN_POINT('Origin',(15.,-10.,4.));
#15893=CARTESIAN_POINT('Origin',(-15.,-10.,8.));
#15894=CARTESIAN_POINT('',(-16.,-5.,8.));
#15895=CARTESIAN_POINT('Origin',(-15.,-10.,4.));
#15896=CARTESIAN_POINT('Origin',(-15.,10.,4.));
#15897=CARTESIAN_POINT('Origin',(-15.,10.,8.));
#15898=CARTESIAN_POINT('Origin',(15.,10.,4.));
#15899=CARTESIAN_POINT('Origin',(15.,10.,8.));
#15900=CARTESIAN_POINT('Origin',(-6.,-6.,8.));
#15901=CARTESIAN_POINT('',(-6.,-6.,8.));
#15902=CARTESIAN_POINT('',(-10.,-6.,8.));
#15903=CARTESIAN_POINT('Origin',(-6.,-4.,8.));
#15904=CARTESIAN_POINT('',(-6.,-4.,8.));
#15905=CARTESIAN_POINT('Origin',(-10.,-4.,8.));
#15906=CARTESIAN_POINT('',(-10.,-4.,8.));
#15907=CARTESIAN_POINT('Origin',(-10.,-6.,8.));
#15908=CARTESIAN_POINT('Origin',(10.,-6.,8.));
#15909=CARTESIAN_POINT('',(10.,-6.,8.));
#15910=CARTESIAN_POINT('',(6.,-6.,8.));
#15911=CARTESIAN_POINT('Origin',(10.,-4.,8.));
#15912=CARTESIAN_POINT('',(10.,-4.,8.));
#15913=CARTESIAN_POINT('Origin',(6.,-4.,8.));
#15914=CARTESIAN_POINT('',(6.,-4.,8.));
#15915=CARTESIAN_POINT('Origin',(6.,-6.,8.));
#15916=CARTESIAN_POINT('Origin',(2.,4.,8.));
#15917=CARTESIAN_POINT('',(2.,4.,8.));
#15918=CARTESIAN_POINT('',(-2.,4.,8.));
#15919=CARTESIAN_POINT('Origin',(2.,6.,8.));
#15920=CARTESIAN_POINT('',(2.,6.,8.));
#15921=CARTESIAN_POINT('Origin',(-2.,6.,8.));
#15922=CARTESIAN_POINT('',(-2.,6.,8.));
#15923=CARTESIAN_POINT('Origin',(-2.,4.,8.));
#15924=CARTESIAN_POINT('Origin',(0.,0.,24.));
#15925=CARTESIAN_POINT('',(-34.,-20.,24.));
#15926=CARTESIAN_POINT('',(-34.,20.,24.));
#15927=CARTESIAN_POINT('',(-34.,-20.,24.));
#15928=CARTESIAN_POINT('',(-20.,10.,24.));
#15929=CARTESIAN_POINT('',(-16.,14.,24.));
#15930=CARTESIAN_POINT('',(-15.5,14.5,24.));
#15931=CARTESIAN_POINT('',(-20.,-14.,24.));
#15932=CARTESIAN_POINT('',(-20.,5.,24.));
#15933=CARTESIAN_POINT('',(20.,-14.,24.));
#15934=CARTESIAN_POINT('',(-10.,-14.,24.));
#15935=CARTESIAN_POINT('',(20.,10.,24.));
#15936=CARTESIAN_POINT('',(20.,-7.,24.));
#15937=CARTESIAN_POINT('',(16.,14.,24.));
#15938=CARTESIAN_POINT('',(17.5,12.5,24.));
#15939=CARTESIAN_POINT('',(8.,14.,24.));
#15940=CARTESIAN_POINT('Origin',(-34.,-20.,24.));
#15941=CARTESIAN_POINT('',(-34.,-20.,24.));
#15942=CARTESIAN_POINT('Origin',(-34.,20.,24.));
#15943=CARTESIAN_POINT('Origin',(-12.,10.,0.));
#15944=CARTESIAN_POINT('',(-12.,10.,0.));
#15945=CARTESIAN_POINT('Origin',(-16.,6.,0.));
#15946=CARTESIAN_POINT('',(-16.,6.,0.));
#15947=CARTESIAN_POINT('Origin',(20.,-14.,0.));
#15948=CARTESIAN_POINT('',(20.,-14.,0.));
#15949=CARTESIAN_POINT('',(20.,10.,0.));
#15950=CARTESIAN_POINT('Origin',(-20.,-14.,0.));
#15951=CARTESIAN_POINT('',(-20.,-14.,0.));
#15952=CARTESIAN_POINT('Origin',(-20.,10.,0.));
#15953=CARTESIAN_POINT('',(-20.,10.,0.));
#15954=CARTESIAN_POINT('Origin',(-16.,-10.,0.));
#15955=CARTESIAN_POINT('Origin',(-16.,14.,0.));
#15956=CARTESIAN_POINT('',(-16.,14.,0.));
#15957=CARTESIAN_POINT('Origin',(16.,14.,0.));
#15958=CARTESIAN_POINT('',(16.,14.,0.));
#15959=CARTESIAN_POINT('Origin',(20.,10.,0.));
#21858=UNCERTAINTY_MEASURE_WITH_UNIT(LENGTH_MEASURE(0.01),#21881,
'DISTANCE_ACCURACY_VALUE',
'Maximum model space distance between geometric entities at asserted c
onnectivities');
#21868=UNCERTAINTY_MEASURE_WITH_UNIT(LENGTH_MEASURE(0.01),#21881,
'DISTANCE_ACCURACY_VALUE',
'Maximum model space distance between geometric entities at asserted c
onnectivities');
#21870=(
GEOMETRIC_REPRESENTATION_CONTEXT(3)
GLOBAL_UNCERTAINTY_ASSIGNED_CONTEXT((#21858))
GLOBAL_UNIT_ASSIGNED_CONTEXT((#21881,#21883,#21884))
REPRESENTATION_CONTEXT('','3D')
);
#21880=(
GEOMETRIC_REPRESENTATION_CONTEXT(3)
GLOBAL_UNCERTAINTY_ASSIGNED_CONTEXT((#21868))
GLOBAL_UNIT_ASSIGNED_CONTEXT((#21881,#21883,#21884))
REPRESENTATION_CONTEXT('','3D')
);
#21881=(
LENGTH_UNIT()
NAMED_UNIT(*)
SI_UNIT(.MILLI.,.METRE.)
);
#21883=(
NAMED_UNIT(*)
PLANE_ANGLE_UNIT()
SI_UNIT($,.RADIAN.)
);
#21884=(
NAMED_UNIT(*)
SI_UNIT($,.STERADIAN.)
SOLID_ANGLE_UNIT()
);
#21886=SHAPE_DEFINITION_REPRESENTATION(#21897,#21925);
#21897=PRODUCT_DEFINITION_SHAPE('',$,#21937);
#21925=SHAPE_REPRESENTATION('',(#6503),#21870);
#21935=PRODUCT_DEFINITION_CONTEXT('part definition',#21970,'design');
#21937=PRODUCT_DEFINITION('Inlet housing','Inlet housing',#21948,#21935);
#21948=PRODUCT_DEFINITION_FORMATION('',$,#21973);
#21970=APPLICATION_CONTEXT(
'Core Data for Automotive Mechanical Design Process');
#21971=PRODUCT_CONTEXT('part definition',#21970,'mechanical');
#21973=PRODUCT('Inlet housing','Inlet housing',$,(#21971));
#21984=PRESENTATION_STYLE_ASSIGNMENT((#21990));
#21990=SURFACE_STYLE_USAGE(.BOTH.,#21996);
#21996=SURFACE_SIDE_STYLE('',(#22002));
#22002=SURFACE_STYLE_FILL_AREA(#22008);
#22008=FILL_AREA_STYLE('Dark blue',(#22014));
#22014=FILL_AREA_STYLE_COLOUR('Dark blue',#22020);
#22020=COLOUR_RGB('Dark blue',0.0901960784313725,0.270588235294118,0.513725490196078);
ENDSEC;
END-ISO-10303-21;
